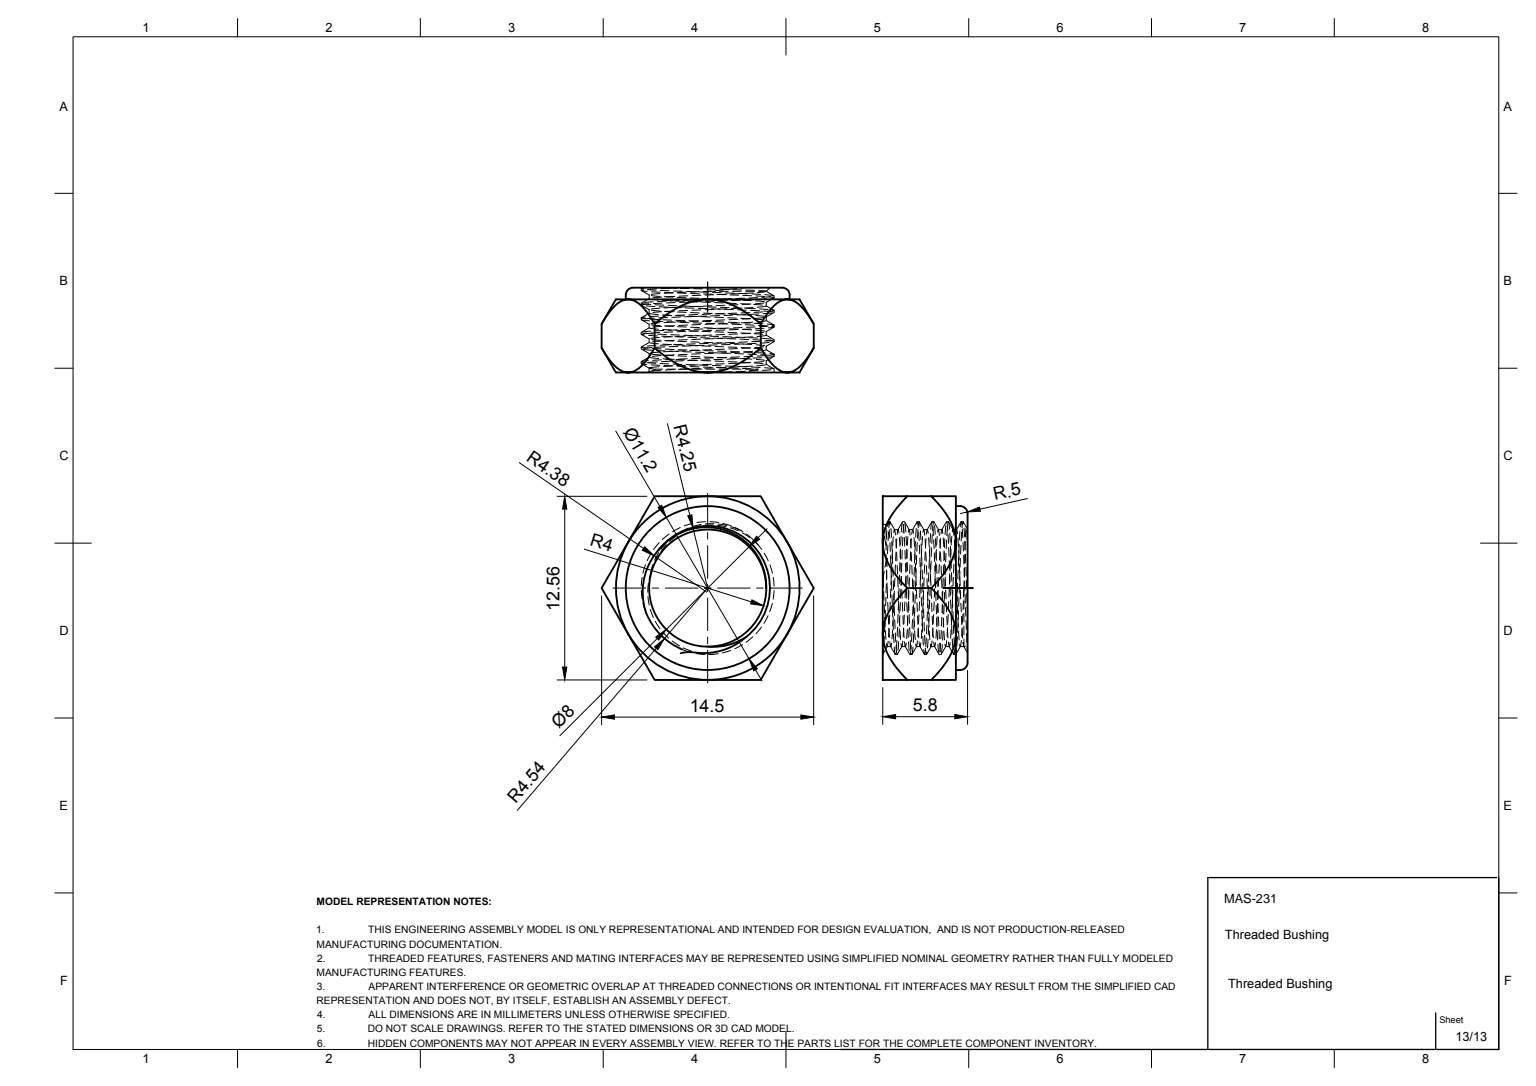
ISO-10303-21;
HEADER;
FILE_DESCRIPTION (('STEP AP214'),
    '1' );
FILE_NAME ( 'Threaded Bushing.step', '2026-10-04T02:08:54', ( '' ), ( '' ), 'STEP AP214', 'Unspecified', '' );
FILE_SCHEMA (( 'AUTOMOTIVE_DESIGN' ));
ENDSEC;
DATA;
#4=CARTESIAN_POINT ( 'NONE',  ( 0.07405724077823318263, -0.4114173227808823330, -0.1787899950787401604 ) ) ;
#5=CARTESIAN_POINT ( 'NONE',  ( -1.094772975963752103E-17, -0.9552165353793071745, -0.1787899950787401882 ) ) ;
#6=CONICAL_SURFACE ( 'NONE', #32970, 0.2471922904502826812, 0.5235987755982992597 ) ;
#7=CARTESIAN_POINT ( 'NONE',  ( -0.2471922332845153669, -0.07944658092495102131, -0.07441910580874835923 ) ) ;
#12=CARTESIAN_POINT ( 'NONE',  ( -0.07444174185955065859, -0.2446304237562738071, -0.1797182628040039087 ) ) ;
#13=CARTESIAN_POINT ( 'NONE',  ( -1.094772975963752103E-17, -0.1049468028749080684, -0.1787899950787401882 ) ) ;
#14=CARTESIAN_POINT ( 'NONE',  ( -1.094772975963752103E-17, -0.2465551180564728440, -0.1787899950787401882 ) ) ;
#15=CARTESIAN_POINT ( 'NONE',  ( 0.1787899950787401604, -0.1013779527021420185, -0.07405724077823318263 ) ) ;
#16=CARTESIAN_POINT ( 'NONE',  ( 0.2471913174570561644, -0.07307272215611475275, -0.08638584879597815958 ) ) ;
#20=DIRECTION ( 'NONE',  ( 0.000000000000000000, 0.000000000000000000, 1.000000000000000000 ) ) ;
#21=CARTESIAN_POINT ( 'NONE',  ( 0.1264236179284866091, -0.4581692912848189247, 0.1264236179284866091 ) ) ;
#25=CARTESIAN_POINT ( 'NONE',  ( -0.1632645169450111788, -0.09126532511120305502, 0.1911722030494052427 ) ) ;
#28=CARTESIAN_POINT ( 'NONE',  ( 0.000000000000000000, 0.09842519685039370636, 0.000000000000000000 ) ) ;
#30=CARTESIAN_POINT ( 'NONE',  ( -0.06523048226347956391, -0.9306102361129453548, -0.1574803149606300301 ) ) ;
#31=CARTESIAN_POINT ( 'NONE',  ( 0.1787899950787401604, -0.3425196849856064762, 0.07405724077823318263 ) ) ;
#34=CARTESIAN_POINT ( 'NONE',  ( -0.07405724077823318263, -1.016732283410803905, 0.1787899950787401604 ) ) ;
#43=CARTESIAN_POINT ( 'NONE',  ( 0.1574803149606299191, -1.139763779420031486, -1.928577636452523993E-17 ) ) ;
#55=CARTESIAN_POINT ( 'NONE',  ( 0.1787899950787401604, 0.01181102367581077228, 0.07405724077823318263 ) ) ;
#64=CARTESIAN_POINT ( 'NONE',  ( 0.1264236179284866091, -1.340183023347348623, 0.1264236179284866091 ) ) ;
#66=CARTESIAN_POINT ( 'NONE',  ( 0.1264236179284866091, -0.3006889763241893943, 0.1264236179284866091 ) ) ;
#74=CARTESIAN_POINT ( 'NONE',  ( -0.1264236179284866091, -1.693405511757259951, 0.1264236179284866091 ) ) ;
#77=CARTESIAN_POINT ( 'NONE',  ( -0.1540809957184832990, -0.09842519685039370636, 0.06850209239233011338 ) ) ;
#78=CARTESIAN_POINT ( 'NONE',  ( 0.1797182628040039087, -1.440496565488557978, 0.07444174185955046430 ) ) ;
#88=CARTESIAN_POINT ( 'NONE',  ( -0.1574803149606297803, -0.7632874014672766938, 0.06523048226347956391 ) ) ;
#89=CARTESIAN_POINT ( 'NONE',  ( 3.284318927891251994E-17, 0.1225393701325037388, 0.1787899950787401882 ) ) ;
#109=CARTESIAN_POINT ( 'NONE',  ( 0.1264236179284866091, -0.1038385826234017734, 0.1264236179284866091 ) ) ;
#117=CARTESIAN_POINT ( 'NONE',  ( 0.1113553986120547346, 0.1250000001075269596, -0.1113553986120547346 ) ) ;
#125=CARTESIAN_POINT ( 'NONE',  ( -0.1787899950787401604, -0.7668562516938051132, -0.07405724077823318263 ) ) ;
#133=ORIENTED_EDGE ( 'NONE', *, *, #14771, .F. ) ;
#135=CARTESIAN_POINT ( 'NONE',  ( 0.07405724077823318263, -0.4901574802611972093, -0.1787899950787401604 ) ) ;
#138=CARTESIAN_POINT ( 'NONE',  ( 3.301370929368692659E-17, -0.8573272741499744498, 0.1797182628040039365 ) ) ;
#149=CARTESIAN_POINT ( 'NONE',  ( 0.1113553986120547346, -0.6328740156405040507, 0.1113553986120547346 ) ) ;
#152=EDGE_CURVE ( 'NONE', #35410, #47206, #15470, .T. ) ;
#155=CARTESIAN_POINT ( 'NONE',  ( 0.1787899950787401882, -0.7288385826234015097, -2.189545951927503898E-17 ) ) ;
#164=CARTESIAN_POINT ( 'NONE',  ( 0.1113553986120547346, -1.617125984251968518, -0.1113553986120547346 ) ) ;
#171=CARTESIAN_POINT ( 'NONE',  ( 0.07405724077823318263, -1.435039370024976391, -0.1787899950787401604 ) ) ;
#177=CYLINDRICAL_SURFACE ( 'NONE', #43516, 0.1574803149606299191 ) ;
#178=CARTESIAN_POINT ( 'NONE',  ( -1.094772975963752103E-17, -0.3411672753158531690, -0.1787899950787401882 ) ) ;
#190=CARTESIAN_POINT ( 'NONE',  ( -0.1787899950787401604, -1.262795275536788386, 0.07405724077823318263 ) ) ;
#191=CARTESIAN_POINT ( 'NONE',  ( 0.1264236179284866091, -1.403051181048598384, 0.1264236179284866091 ) ) ;
#193=ADVANCED_FACE ( 'NONE', ( #1523 ), #30571, .F. ) ;
#200=CARTESIAN_POINT ( 'NONE',  ( 0.1113553986120547346, -0.3277559055118110520, 0.1113553986120547346 ) ) ;
#206=CARTESIAN_POINT ( 'NONE',  ( -0.1113553986120547346, -0.4950787400499527813, -0.1113553986120547346 ) ) ;
#211=CARTESIAN_POINT ( 'NONE',  ( -0.1574803149606297803, 0.1028543308161884995, 0.06523048226347956391 ) ) ;
#213=CARTESIAN_POINT ( 'NONE',  ( 0.07405724077823318263, -1.508858267662772867, -0.1787899950787401604 ) ) ;
#214=CARTESIAN_POINT ( 'NONE',  ( -0.1574803149606297803, -1.511318897530268712, 0.06523048226347956391 ) ) ;
#215=CARTESIAN_POINT ( 'NONE',  ( 0.1264236179284866091, -0.7780511810485984947, 0.1264236179284866091 ) ) ;
#216=CARTESIAN_POINT ( 'NONE',  ( -0.06523048226347956391, -1.097933070866141225, -0.1574803149606300301 ) ) ;
#226=CARTESIAN_POINT ( 'NONE',  ( 0.1574803149606300301, -1.339074803042078932, 0.06523048226347956391 ) ) ;
#253=CARTESIAN_POINT ( 'NONE',  ( -0.1787899950787401604, -0.4360236219934807145, 0.07405724077823318263 ) ) ;
#255=CARTESIAN_POINT ( 'NONE',  ( 0.1787899950787401604, -0.8494094487651332459, 0.07405724077823318263 ) ) ;
#258=CARTESIAN_POINT ( 'NONE',  ( -0.1797182628040039087, -0.2003390851735964984, -0.07444174185955065859 ) ) ;
#261=CARTESIAN_POINT ( 'NONE',  ( 0.1787899950787401604, -0.1172499524812071620, 0.07405724077823318263 ) ) ;
#262=CARTESIAN_POINT ( 'NONE',  ( -0.1264236179284866091, -0.1186023621509608300, 0.1264236179284866091 ) ) ;
#263=CARTESIAN_POINT ( 'NONE',  ( 0.2471920270787851259, -0.07566776403336712697, -0.08167830084036972749 ) ) ;
#268=CARTESIAN_POINT ( 'NONE',  ( -0.1787899950787401604, -0.4311023621509605386, 0.07405724077823318263 ) ) ;
#275=CARTESIAN_POINT ( 'NONE',  ( 0.1574803149606299191, -0.9429133857192442125, -1.928577636452523993E-17 ) ) ;
#276=CARTESIAN_POINT ( 'NONE',  ( 0.1264236179284866091, -0.2170275590013547307, -0.1264236179284866091 ) ) ;
#279=CARTESIAN_POINT ( 'NONE',  ( 0.1787899950787401604, -1.041338582623402287, -0.07405724077823318263 ) ) ;
#287=CARTESIAN_POINT ( 'NONE',  ( -0.06523048226347956391, -1.206200787294047228, -0.1574803149606300301 ) ) ;
#297=CARTESIAN_POINT ( 'NONE',  ( -0.1787899950787401604, 0.03149606304588949135, -0.07405724077823318263 ) ) ;
#306=CARTESIAN_POINT ( 'NONE',  ( 0.1787899950787401604, -1.258982235945774075, 0.07405724077823318263 ) ) ;
#309=CARTESIAN_POINT ( 'NONE',  ( -0.07405724077823318263, -0.2047244093950554844, -0.1787899950787401604 ) ) ;
#313=CARTESIAN_POINT ( 'NONE',  ( 0.000000000000000000, -0.09842519685039370636, 0.000000000000000000 ) ) ;
#317=CARTESIAN_POINT ( 'NONE',  ( -0.1787899950787401604, -1.656496062938362268, 0.07405724077823318263 ) ) ;
#318=CARTESIAN_POINT ( 'NONE',  ( 0.1787899950787401604, -1.715551181048599716, 0.07405724077823318263 ) ) ;
#320=APPLICATION_CONTEXT ( 'automotive_design' ) ;
#324=CARTESIAN_POINT ( 'NONE',  ( 3.301370929368692659E-17, -1.369138297772021673, 0.1797182628040039365 ) ) ;
#329=B_SPLINE_CURVE_WITH_KNOTS ( 'NONE', 3,
 ( #40653, #8085, #22708, #37314, #20055, #46161, #9758, #34449, #45674, #2308, #13357, #45919, #24148, #16938, #24370, #42328, #41837, #20757 ),
 .UNSPECIFIED., .F., .F.,
 ( 4, 2, 2, 2, 1, 1, 2, 2, 2, 4 ),
 ( 0.000000000000000000, 0.2499999999999993894, 0.3749999999999990008, 0.4374999999999987788, 0.4687499999999986122, 0.4843749999999986122, 0.4921874999999985567, 0.4999999999999985567, 0.7499999999999992228, 1.000000000000000000 ),
 .UNSPECIFIED. ) ;
#335=CARTESIAN_POINT ( 'NONE',  ( 0.1113553986120547346, -0.8198818896562519720, -0.1113553986120547346 ) ) ;
#349=CARTESIAN_POINT ( 'NONE',  ( -0.1270800023317771588, 0.1515309935665608287, -0.1270800023317771588 ) ) ;
#350=CARTESIAN_POINT ( 'NONE',  ( 0.1574803149606300301, -1.063484251860977059, 0.06523048226347956391 ) ) ;
#356=CARTESIAN_POINT ( 'NONE',  ( 0.07405724077823318263, -0.2244094487651340231, 0.1787899950787401604 ) ) ;
#360=CARTESIAN_POINT ( 'NONE',  ( -0.009745153983727199848, -0.04193537623276894638, 0.2798067035903421540 ) ) ;
#364=CARTESIAN_POINT ( 'NONE',  ( -9.642888182262618425E-18, 0.09055118120988918384, -0.1574803149606299191 ) ) ;
#368=VECTOR ( 'NONE', #12553, 39.37007874015748143 ) ;
#369=CARTESIAN_POINT ( 'NONE',  ( 0.1787899950787401882, -0.9021908973630964335, -2.189545951927503898E-17 ) ) ;
#372=AXIS2_PLACEMENT_3D ( 'NONE', #5692, #17413, #32052 ) ;
#373=ORIENTED_EDGE ( 'NONE', *, *, #26554, .F. ) ;
#379=CARTESIAN_POINT ( 'NONE',  ( -0.1787899950787401604, -0.4753937007336378473, 0.07405724077823318263 ) ) ;
#380=EDGE_CURVE ( 'NONE', #22666, #46167, #21394, .T. ) ;
#383=CARTESIAN_POINT ( 'NONE',  ( -0.1270800023317771588, -1.059098927693281622, 0.1270800023317771588 ) ) ;
#392=CARTESIAN_POINT ( 'NONE',  ( -0.1235961452251413406, -0.09842519685039370636, 0.2140748031496062798 ) ) ;
#396=CARTESIAN_POINT ( 'NONE',  ( -0.1787899950787401604, -0.8248031495525351975, 0.07405724077823318263 ) ) ;
#399=FACE_OUTER_BOUND ( 'NONE', #15103, .T. ) ;
#404=CARTESIAN_POINT ( 'NONE',  ( -0.06523048226347956391, -1.727854330708660902, -0.1574803149606300301 ) ) ;
#418=CARTESIAN_POINT ( 'NONE',  ( 0.07405724077823318263, -0.3436279052371127296, -0.1787899950787401604 ) ) ;
#419=CARTESIAN_POINT ( 'NONE',  ( 0.08603670706143877467, -0.09842519685039370636, 0.1221131442762555253 ) ) ;
#421=PLANE ( 'NONE',  #8031 ) ;
#430=CARTESIAN_POINT ( 'NONE',  ( 0.1787899950787401882, -1.284940944828125930, -2.189545951927503898E-17 ) ) ;
#431=CARTESIAN_POINT ( 'NONE',  ( 0.1264236179284866091, -1.481791338528913426, 0.1264236179284866091 ) ) ;
#438=CARTESIAN_POINT ( 'NONE',  ( -0.1113553986120547346, -0.2194881889763779514, 0.1113553986120547346 ) ) ;
#441=CARTESIAN_POINT ( 'NONE',  ( -0.1787899950787401604, -0.2047244093950554844, -0.07405724077823318263 ) ) ;
#453=CARTESIAN_POINT ( 'NONE',  ( -0.1264236179284866091, -1.531003936954110189, 0.1264236179284866091 ) ) ;
#454=CARTESIAN_POINT ( 'NONE',  ( 0.07405724077823318263, -0.8198818897100156322, 0.1787899950787401604 ) ) ;
#455=CARTESIAN_POINT ( 'NONE',  ( -0.06523048226347956391, -1.240649606299213614, 0.1574803149606297803 ) ) ;
#476=EDGE_CURVE ( 'NONE', #44070, #30751, #10635, .T. ) ;
#478=CARTESIAN_POINT ( 'NONE',  ( -0.2009290272083082973, -0.09842519685039370636, 0.1224581209280712624 ) ) ;
#484=CARTESIAN_POINT ( 'NONE',  ( 0.1787899950787401604, -0.8937007873478103326, 0.07405724077823318263 ) ) ;
#485=CARTESIAN_POINT ( 'NONE',  ( -0.1264236179284866091, -0.9010826771115905132, 0.1264236179284866091 ) ) ;
#488=CARTESIAN_POINT ( 'NONE',  ( 0.1797182628040039087, -0.2544729434413131597, -0.07444174185955065859 ) ) ;
#490=CARTESIAN_POINT ( 'NONE',  ( 0.07405724077823318263, -0.03248031490686641154, 0.1787899950787401604 ) ) ;
#501=CARTESIAN_POINT ( 'NONE',  ( -0.1787899950787401882, -0.3203740156942680994, 0.000000000000000000 ) ) ;
#503=CARTESIAN_POINT ( 'NONE',  ( 0.1787899950787401604, -1.164370078686393306, 0.07405724077823318263 ) ) ;
#524=CARTESIAN_POINT ( 'NONE',  ( -0.1264236179284866091, -0.08907480309584270284, -0.1264236179284866091 ) ) ;
#528=CARTESIAN_POINT ( 'NONE',  ( -0.1750152858685271595, -0.09851385417196180383, -0.1786646369836015769 ) ) ;
#532=CARTESIAN_POINT ( 'NONE',  ( 0.1787899950787401604, -1.455832629646562015, 0.07405724077823318263 ) ) ;
#534=CARTESIAN_POINT ( 'NONE',  ( 0.07405724077823318263, -0.4212598424659216856, 0.1787899950787401604 ) ) ;
#542=CARTESIAN_POINT ( 'NONE',  ( 0.07405724077823318263, -1.646653543253324026, 0.1787899950787401604 ) ) ;
#543=CARTESIAN_POINT ( 'NONE',  ( -0.1787899950787401604, -1.651574803095843258, 0.07405724077823318263 ) ) ;
#548=CARTESIAN_POINT ( 'NONE',  ( -1.100456976456230270E-17, -1.349453258401942746, -0.1797182628040039365 ) ) ;
#557=CARTESIAN_POINT ( 'NONE',  ( -1.094772975963752103E-17, 0.1422244095025824717, -0.1787899950787401882 ) ) ;
#570=CARTESIAN_POINT ( 'NONE',  ( 0.1797182628040039365, -0.06008317966178563369, -2.200913952912460540E-17 ) ) ;
#572=CARTESIAN_POINT ( 'NONE',  ( -0.1787899950787401604, -1.188976377898991688, -0.07405724077823318263 ) ) ;
#579=CARTESIAN_POINT ( 'NONE',  ( 3.284318927891251994E-17, -0.2268700786863941110, 0.1787899950787401882 ) ) ;
#582=EDGE_CURVE ( 'NONE', #35894, #1072, #33031, .T. ) ;
#583=CARTESIAN_POINT ( 'NONE',  ( -0.06523048226347935574, 0.09793307086614168322, 0.1574803149606300301 ) ) ;
#585=ORIENTED_EDGE ( 'NONE', *, *, #39318, .F. ) ;
#586=EDGE_CURVE ( 'NONE', #31109, #36213, #45187, .T. ) ;
#588=CARTESIAN_POINT ( 'NONE',  ( -0.1113553986120547346, 0.1348425197925665342, -0.1113553986120547346 ) ) ;
#594=CARTESIAN_POINT ( 'NONE',  ( 0.07405724077823318263, -0.9883129446071914348, 0.1787899950787401604 ) ) ;
#596=CARTESIAN_POINT ( 'NONE',  ( 0.1787899950787401604, 0.1348425197388028463, 0.07405724077823318263 ) ) ;
#605=CARTESIAN_POINT ( 'NONE',  ( -0.07444174185955065859, -1.071402077299582034, -0.1797182628040039087 ) ) ;
#612=CARTESIAN_POINT ( 'NONE',  ( 0.000000000000000000, -0.09842519685039370636, 0.000000000000000000 ) ) ;
#615=CARTESIAN_POINT ( 'NONE',  ( -0.07405724077823318263, -0.7411417322297018107, 0.1787899950787401604 ) ) ;
#620=LINE ( 'NONE', #7837, #8860 ) ;
#621=CARTESIAN_POINT ( 'NONE',  ( -0.1574803149606300301, -1.644192913385826404, -0.06523048226347956391 ) ) ;
#629=CARTESIAN_POINT ( 'NONE',  ( -0.06523048226347956391, 0.05364173239099160467, -0.1574803149606300301 ) ) ;
#642=CARTESIAN_POINT ( 'NONE',  ( -0.07405724077823318263, -0.5995334170481365632, 0.1787899950787401604 ) ) ;
#645=DIRECTION ( 'NONE',  ( 0.000000000000000000, 1.000000000000000000, 0.000000000000000000 ) ) ;
#647=CARTESIAN_POINT ( 'NONE',  ( -0.1264236179284866091, -1.743726330433962524, 0.1264236179284866091 ) ) ;
#652=CARTESIAN_POINT ( 'NONE',  ( 0.1264236179284866091, -1.289862204670645607, 0.1264236179284866091 ) ) ;
#654=CARTESIAN_POINT ( 'NONE',  ( 0.07405724077823318263, -1.587598425143086800, -0.1787899950787401604 ) ) ;
#663=CARTESIAN_POINT ( 'NONE',  ( -0.1113553986120547346, -0.2293307086614173318, -0.1113553986120547346 ) ) ;
#666=CARTESIAN_POINT ( 'NONE',  ( -0.1427036564498907201, -0.09517011092317628762, -0.1080556551396093801 ) ) ;
#672=CARTESIAN_POINT ( 'NONE',  ( -0.1690815567638284667, -0.08955967048287666321, -0.02567216645670302583 ) ) ;
#681=CARTESIAN_POINT ( 'NONE',  ( -0.07405724077823318263, -1.607283464513165949, 0.1787899950787401604 ) ) ;
#682=CARTESIAN_POINT ( 'NONE',  ( -0.1787899950787401604, -0.7952755904974174728, -0.07405724077823318263 ) ) ;
#683=CARTESIAN_POINT ( 'NONE',  ( -0.1113553986120547346, -1.252952755905511806, -0.1113553986120547346 ) ) ;
#704=CARTESIAN_POINT ( 'NONE',  ( -0.1919739359782932919, -0.09842519685039370636, 0.1351110688617698785 ) ) ;
#713=B_SPLINE_CURVE_WITH_KNOTS ( 'NONE', 3,
 ( #38757, #41598, #38277, #27534 ),
 .UNSPECIFIED., .F., .F.,
 ( 4, 4 ),
 ( 0.000000000000000000, 1.000000000000000000 ),
 .UNSPECIFIED. ) ;
#714=CARTESIAN_POINT ( 'NONE',  ( 0.1264236179284866091, -0.9256889763241890057, -0.1264236179284866091 ) ) ;
#715=CARTESIAN_POINT ( 'NONE',  ( -0.07405724077823318263, -0.9921259841982054128, -0.1787899950787401604 ) ) ;
#718=CARTESIAN_POINT ( 'NONE',  ( 0.07444174185955065859, -0.3824256993468252430, 0.1797182628040039087 ) ) ;
#719=CARTESIAN_POINT ( 'NONE',  ( -0.1574803149606297803, 0.09301181102362203468, 0.06523048226347956391 ) ) ;
#720=CARTESIAN_POINT ( 'NONE',  ( 0.1787899950787401604, -0.02755905506434671789, 0.07405724077823318263 ) ) ;
#733=CARTESIAN_POINT ( 'NONE',  ( -0.07405724077823318263, -0.2342519684501733479, 0.1787899950787401604 ) ) ;
#735=CARTESIAN_POINT ( 'NONE',  ( -1.094772975963752103E-17, -1.270177165300566902, -0.1787899950787401882 ) ) ;
#744=CARTESIAN_POINT ( 'NONE',  ( 0.1574803149606299191, -1.218503936900346529, -1.928577636452523993E-17 ) ) ;
#746=CARTESIAN_POINT ( 'NONE',  ( 0.01529509707327361516, -0.09839281432029055308, -0.1781982434423184380 ) ) ;
#757=FACE_OUTER_BOUND ( 'NONE', #34050, .T. ) ;
#762=CARTESIAN_POINT ( 'NONE',  ( 0.1264236179284866091, -1.379553102087506256, 0.1264236179284866091 ) ) ;
#763=VERTEX_POINT ( 'NONE', #18849 ) ;
#765=CARTESIAN_POINT ( 'NONE',  ( -0.07405724077823318263, -0.4655511810485986057, 0.1787899950787401604 ) ) ;
#774=CARTESIAN_POINT ( 'NONE',  ( -0.1787899950787401604, -1.740157480261197875, -0.07405724077823318263 ) ) ;
#775=CARTESIAN_POINT ( 'NONE',  ( 0.1787899950787401604, -1.710629921206078041, -0.07405724077823318263 ) ) ;
#781=CARTESIAN_POINT ( 'NONE',  ( 3.301370929368692659E-17, -1.447878455252336716, 0.1797182628040039365 ) ) ;
#790=CARTESIAN_POINT ( 'NONE',  ( -0.1574803149606297803, -0.8026574802074324388, 0.06523048226347956391 ) ) ;
#791=CARTESIAN_POINT ( 'NONE',  ( 0.1264236179284866091, 0.1274606299750234428, 0.1264236179284866091 ) ) ;
#799=VERTEX_POINT ( 'NONE', #25603 ) ;
#802=VERTEX_POINT ( 'NONE', #40870 ) ;
#803=CARTESIAN_POINT ( 'NONE',  ( 0.1797182628040039365, -0.02071310092162823024, -2.200913952912460540E-17 ) ) ;
#804=CARTESIAN_POINT ( 'NONE',  ( 0.1264236179284866091, -1.289862204670645607, 0.1264236179284866091 ) ) ;
#812=CARTESIAN_POINT ( 'NONE',  ( -1.094772975963752103E-17, -0.1678149605761578844, -0.1787899950787401882 ) ) ;
#820=CARTESIAN_POINT ( 'NONE',  ( -0.06523048226347956391, -0.08907480304207930633, 0.1574803149606297803 ) ) ;
#826=CARTESIAN_POINT ( 'NONE',  ( -0.1264236179284866091, -0.9267971965756948149, -0.1264236179284866091 ) ) ;
#828=CARTESIAN_POINT ( 'NONE',  ( -0.07405724077823318263, 0.08562992131360593062, 0.1787899950787401604 ) ) ;
#835=AXIS2_PLACEMENT_3D ( 'NONE', #29189, #20976, #40131 ) ;
#836=CARTESIAN_POINT ( 'NONE',  ( 0.07405724077823318263, -0.5442913385289138706, 0.1787899950787401604 ) ) ;
#843=CARTESIAN_POINT ( 'NONE',  ( 0.1270800023317771588, -1.039413888323202695, -0.1270800023317771588 ) ) ;
#844=CARTESIAN_POINT ( 'NONE',  ( 0.1731942250296887864, 0.1299212598425197318, 0.03910837931845940335 ) ) ;
#854=CARTESIAN_POINT ( 'NONE',  ( 0.1113553986120547346, -0.7017716534357795188, -0.1113553986120547346 ) ) ;
#858=CARTESIAN_POINT ( 'NONE',  ( -0.1787899950787401882, -0.7091535432533228045, 0.000000000000000000 ) ) ;
#866=CARTESIAN_POINT ( 'NONE',  ( -0.06523048226347956391, -1.634350393700787496, 0.1574803149606297803 ) ) ;
#874=CARTESIAN_POINT ( 'NONE',  ( -1.094772975963752103E-17, -1.471948818843874074, -0.1787899950787401882 ) ) ;
#883=CARTESIAN_POINT ( 'NONE',  ( 0.07405724077823318263, -0.5798483776780570809, -0.1787899950787401604 ) ) ;
#884=CARTESIAN_POINT ( 'NONE',  ( 0.02785187604205846545, -0.08955996554169548540, 0.2176922158899677329 ) ) ;
#891=CARTESIAN_POINT ( 'NONE',  ( 0.2471922904502826812, -0.03219022224904106305, 0.1427165354330708902 ) ) ;
#896=CARTESIAN_POINT ( 'NONE',  ( 0.1264236179284866091, -1.358759842465921297, -0.1264236179284866091 ) ) ;
#897=CARTESIAN_POINT ( 'NONE',  ( 0.07405724077823318263, -1.523622047190330564, 0.1787899950787401604 ) ) ;
#906=CARTESIAN_POINT ( 'NONE',  ( 0.1574803149606300301, -0.2416338582677168279, -0.06523048226347956391 ) ) ;
#917=CARTESIAN_POINT ( 'NONE',  ( 0.1113553986120547346, -0.5442913384751496553, -0.1113553986120547346 ) ) ;
#919=CARTESIAN_POINT ( 'NONE',  ( -0.1547363509471673670, -0.08956143428533665241, 0.05872201630027999719 ) ) ;
#925=CARTESIAN_POINT ( 'NONE',  ( 2.892866454678787531E-17, -0.01771653543307086590, 0.1574803149606299191 ) ) ;
#926=CARTESIAN_POINT ( 'NONE',  ( 0.1787899950787401604, -1.558070866087969630, 0.07405724077823318263 ) ) ;
#927=CARTESIAN_POINT ( 'NONE',  ( -0.07405724077823318263, -0.9576771653005667906, -0.1787899950787401604 ) ) ;
#928=CARTESIAN_POINT ( 'NONE',  ( 0.06523048226347956391, -1.142224409448818534, -0.1574803149606300301 ) ) ;
#949=CARTESIAN_POINT ( 'NONE',  ( -0.1522652282534474322, -0.09842519685039370636, -0.2000201865208625918 ) ) ;
#958=CARTESIAN_POINT ( 'NONE',  ( 0.1264236179284866091, -0.8174212597887557941, 0.1264236179284866091 ) ) ;
#959=CARTESIAN_POINT ( 'NONE',  ( -0.1787899950787401882, -1.063484251914740275, 0.000000000000000000 ) ) ;
#963=CARTESIAN_POINT ( 'NONE',  ( -0.1797182628040039087, -0.3922682190318645401, 0.07444174185955065859 ) ) ;
#965=CARTESIAN_POINT ( 'NONE',  ( 0.1264236179284866091, -0.1382874015210397711, -0.1264236179284866091 ) ) ;
#977=CARTESIAN_POINT ( 'NONE',  ( 0.1787899950787401604, -0.4557086613635593086, -0.07405724077823318263 ) ) ;
#979=CARTESIAN_POINT ( 'NONE',  ( -0.1787899950787401882, -1.299704724355684959, 0.000000000000000000 ) ) ;
#987=CARTESIAN_POINT ( 'NONE',  ( -0.06523048226347956391, -1.166830708553891371, -0.1574803149606300301 ) ) ;
#992=CARTESIAN_POINT ( 'NONE',  ( -0.05462378473120000494, -0.09842519705081047288, -0.1712222294880737516 ) ) ;
#1009=CARTESIAN_POINT ( 'NONE',  ( -0.1787899950787401882, -1.473057039095379883, 0.000000000000000000 ) ) ;
#1011=CARTESIAN_POINT ( 'NONE',  ( 0.1264236179284866091, -0.3695866141194649179, -0.1264236179284866091 ) ) ;
#1021=CARTESIAN_POINT ( 'NONE',  ( 0.1264236179284866091, -1.722933070812378009, 0.1264236179284866091 ) ) ;
#1022=CARTESIAN_POINT ( 'NONE',  ( -0.1787899950787401882, -1.772145669237574994, 0.000000000000000000 ) ) ;
#1024=ORIENTED_EDGE ( 'NONE', *, *, #5865, .T. ) ;
#1028=CARTESIAN_POINT ( 'NONE',  ( -0.1113553986120547346, -0.7312992125984252301, 0.1113553986120547346 ) ) ;
#1030=CARTESIAN_POINT ( 'NONE',  ( -0.1797182628040039087, -1.342071368638164675, -0.07444174185955065859 ) ) ;
#1039=CARTESIAN_POINT ( 'NONE',  ( -0.07405724077823318263, 0.1200787402112438867, 0.1787899950787401604 ) ) ;
#1051=CARTESIAN_POINT ( 'NONE',  ( 0.1797182628040039365, -0.09945325840194331468, -2.200913952912460540E-17 ) ) ;
#1052=CARTESIAN_POINT ( 'NONE',  ( -0.1787899950787401604, -1.267716535379307619, -0.07405724077823318263 ) ) ;
#1061=CARTESIAN_POINT ( 'NONE',  ( -0.06648378651140092466, -0.08350519546677943883, -0.2470477387548498660 ) ) ;
#1062=CIRCLE ( 'NONE', #4901, 0.2471922904502826812 ) ;
#1065=CARTESIAN_POINT ( 'NONE',  ( -0.06523048226347956391, 0.01427165365083412490, -0.1574803149606300301 ) ) ;
#1071=CARTESIAN_POINT ( 'NONE',  ( -1.094772975963752103E-17, -0.9317184564182144912, -0.1787899950787401882 ) ) ;
#1072=VERTEX_POINT ( 'NONE', #4941 ) ;
#1073=CARTESIAN_POINT ( 'NONE',  ( -0.07405724077823318263, 0.006889763833291078637, 0.1787899950787401604 ) ) ;
#1081=CARTESIAN_POINT ( 'NONE',  ( 3.284318927891251994E-17, -0.5467519684501732646, 0.1787899950787401882 ) ) ;
#1086=CARTESIAN_POINT ( 'NONE',  ( 3.301370929368692659E-17, -0.9360674316302894926, 0.1797182628040039365 ) ) ;
#1097=CARTESIAN_POINT ( 'NONE',  ( -0.1787899950787401604, 0.08070866147108628208, 0.07405724077823318263 ) ) ;
#1102=CARTESIAN_POINT ( 'NONE',  ( 3.284318927891251994E-17, -0.7780511810485984947, 0.1787899950787401882 ) ) ;
#1106=CARTESIAN_POINT ( 'NONE',  ( -0.1113553986120547346, -1.715551180994834723, -0.1113553986120547346 ) ) ;
#1109=CARTESIAN_POINT ( 'NONE',  ( 0.06523048226347956391, -1.654035433070866423, -0.1574803149606300301 ) ) ;
#1115=CARTESIAN_POINT ( 'NONE',  ( 0.1787899950787401604, 0.09547244099864542199, -0.07405724077823318263 ) ) ;
#1116=CARTESIAN_POINT ( 'NONE',  ( -1.094772975963752103E-17, -1.511318897584031484, -0.1787899950787401882 ) ) ;
#1128=CARTESIAN_POINT ( 'NONE',  ( -0.07405724077823318263, -0.5601633383079792639, 0.1787899950787401604 ) ) ;
#1129=CARTESIAN_POINT ( 'NONE',  ( -0.2359654055811763462, -0.08955966323838543408, 0.02109953285558708452 ) ) ;
#1133=CARTESIAN_POINT ( 'NONE',  ( 0.000000000000000000, 0.09842519685039370636, 0.000000000000000000 ) ) ;
#1135=CARTESIAN_POINT ( 'NONE',  ( 3.284318927891251994E-17, -1.778175149331602256, 0.1787899950787401882 ) ) ;
#1138=CARTESIAN_POINT ( 'NONE',  ( -0.1787899950787401604, -1.341535433017102541, 0.07405724077823318263 ) ) ;
#1139=CARTESIAN_POINT ( 'NONE',  ( 3.284318927891251994E-17, -1.486712598371433103, 0.1787899950787401882 ) ) ;
#1146=CARTESIAN_POINT ( 'NONE',  ( -0.06523048226347956391, -0.2317913385826771144, -0.1574803149606300301 ) ) ;
#1152=CARTESIAN_POINT ( 'NONE',  ( -0.1545411696117860445, -0.09842519685039370636, -0.08990488994085453489 ) ) ;
#1156=CARTESIAN_POINT ( 'NONE',  ( -0.06523048226347956391, -0.5369094487113711400, -0.1574803149606300301 ) ) ;
#1157=CARTESIAN_POINT ( 'NONE',  ( -0.1807077244524717130, -0.08350519546717886932, 0.1811005174367878168 ) ) ;
#1159=CARTESIAN_POINT ( 'NONE',  ( -0.1009669065382620273, -0.08956173115452045752, 0.1239132365318445506 ) ) ;
#1165=CARTESIAN_POINT ( 'NONE',  ( 0.07405724077823318263, -1.681102362150960650, 0.1787899950787401604 ) ) ;
#1166=CARTESIAN_POINT ( 'NONE',  ( 0.1264236179284866091, -0.9256889763241890057, -0.1264236179284866091 ) ) ;
#1167=CARTESIAN_POINT ( 'NONE',  ( 0.06523048226347956391, -1.220964566929134687, -0.1574803149606300301 ) ) ;
#1175=CARTESIAN_POINT ( 'NONE',  ( 0.1113553986120547346, -1.371062992018456717, -0.1113553986120547346 ) ) ;
#1185=CARTESIAN_POINT ( 'NONE',  ( 0.05837987205262076124, 0.07899857248962811884, 0.2517274360213053175 ) ) ;
#1191=CARTESIAN_POINT ( 'NONE',  ( 0.01579849016993808974, -0.09851382911741830839, 0.1545074369619750254 ) ) ;
#1201=CARTESIAN_POINT ( 'NONE',  ( 0.1787899950787401604, -0.8887795275052913224, -0.07405724077823318263 ) ) ;
#1202=CARTESIAN_POINT ( 'NONE',  ( -0.1787899950787401604, -1.100393700733639069, 0.07405724077823318263 ) ) ;
#1205=CARTESIAN_POINT ( 'NONE',  ( 0.07444174185955046430, -0.4070319985594234580, -0.1797182628040039087 ) ) ;
#1206=CARTESIAN_POINT ( 'NONE',  ( -0.1574803149606300301, -1.791830708553890261, -0.06523048226347956391 ) ) ;
#1207=CARTESIAN_POINT ( 'NONE',  ( -0.1113553986120547346, 0.1643700787401574936, -0.1113553986120547346 ) ) ;
#1217=CARTESIAN_POINT ( 'NONE',  ( 3.284318927891251994E-17, -0.3892716534895436786, 0.1787899950787401882 ) ) ;
#1219=CARTESIAN_POINT ( 'NONE',  ( -0.07405724077823318263, -1.292322834591905778, 0.1787899950787401604 ) ) ;
#1230=CARTESIAN_POINT ( 'NONE',  ( 0.04979026054520423183, -0.09842589400172224723, -0.1717333828277539942 ) ) ;
#1235=ADVANCED_FACE ( 'NONE', ( #12987 ), #46257, .F. ) ;
#1240=CARTESIAN_POINT ( 'NONE',  ( -0.1947286603072740374, -0.09851385302161634605, -0.1548760358685606353 ) ) ;
#1247=CARTESIAN_POINT ( 'NONE',  ( -0.1264236179284866091, -1.399238141457584739, -0.1264236179284866091 ) ) ;
#1250=CARTESIAN_POINT ( 'NONE',  ( 0.1264236179284866091, -0.4581692912848189247, 0.1264236179284866091 ) ) ;
#1254=CARTESIAN_POINT ( 'NONE',  ( -0.2471922904502826812, -0.09842519685039370636, 5.914624404477007554E-17 ) ) ;
#1257=CARTESIAN_POINT ( 'NONE',  ( -0.07405724077823318263, -1.730314960576156968, 0.1787899950787401604 ) ) ;
#1258=CARTESIAN_POINT ( 'NONE',  ( -0.07405724077823318263, -1.804133858213953889, 0.1787899950787401604 ) ) ;
#1264=CARTESIAN_POINT ( 'NONE',  ( 0.1113553986120547346, -0.7608267716535432879, 0.1113553986120547346 ) ) ;
#1266=CARTESIAN_POINT ( 'NONE',  ( -0.1797182628040039087, -1.573370581236589683, 0.07444174185955065859 ) ) ;
#1275=CARTESIAN_POINT ( 'NONE',  ( -0.1787899950787401604, -0.007874015694267972806, -0.07405724077823318263 ) ) ;
#1288=CARTESIAN_POINT ( 'NONE',  ( -0.07444174185955065859, -0.08715010879564398516, -0.1797182628040039087 ) ) ;
#1289=CARTESIAN_POINT ( 'NONE',  ( 0.1787899950787401604, -1.366141732229700478, 0.07405724077823318263 ) ) ;
#1297=EDGE_CURVE ( 'NONE', #10382, #802, #31438, .T. ) ;
#1299=EDGE_LOOP ( 'NONE', ( #44521, #27760, #38088 ) ) ;
#1306=CARTESIAN_POINT ( 'NONE',  ( -9.642888182262618425E-18, 0.01181102372957427288, -0.1574803149606299191 ) ) ;
#1311=CARTESIAN_POINT ( 'NONE',  ( 0.1787899950787401604, -1.017840503662311047, -0.07405724077823318263 ) ) ;
#1313=CARTESIAN_POINT ( 'NONE',  ( 0.07405724077823318263, 0.09055118115612580121, 0.1787899950787401604 ) ) ;
#1318=CARTESIAN_POINT ( 'NONE',  ( 0.07405724077823318263, -0.7017716534895438452, 0.1787899950787401604 ) ) ;
#1323=CARTESIAN_POINT ( 'NONE',  ( 0.1797182628040039087, -1.041874518244462422, -0.07444174185955065859 ) ) ;
#1331=CARTESIAN_POINT ( 'NONE',  ( 0.06523048226347956391, -0.6993110235145204578, -0.1574803149606300301 ) ) ;
#1337=CARTESIAN_POINT ( 'NONE',  ( -0.07405724077823318263, -0.8592519684501739308, 0.1787899950787401604 ) ) ;
#1343=CARTESIAN_POINT ( 'NONE',  ( -0.1574803149606297803, -1.668799212490898576, 0.06523048226347956391 ) ) ;
#1347=CARTESIAN_POINT ( 'NONE',  ( 2.892866454678787531E-17, -1.789370078740157410, 0.1574803149606299191 ) ) ;
#1352=CARTESIAN_POINT ( 'NONE',  ( -0.06523048226347956391, -0.3400590550105831444, -0.1574803149606300301 ) ) ;
#1353=CARTESIAN_POINT ( 'NONE',  ( 0.1787899950787401882, -1.599901574749385880, -2.189545951927503898E-17 ) ) ;
#1364=CARTESIAN_POINT ( 'NONE',  ( -0.07405724077823318263, -0.4961869603552226948, -0.1787899950787401604 ) ) ;
#1365=CARTESIAN_POINT ( 'NONE',  ( 0.1120789836339634027, -0.08956013912318722126, 0.1830409950616023740 ) ) ;
#1371=CARTESIAN_POINT ( 'NONE',  ( 0.1787899950787401604, -1.558070866087969630, -0.07405724077823318263 ) ) ;
#1372=CARTESIAN_POINT ( 'NONE',  ( 0.1264236179284866091, -1.590059055064346305, -0.1264236179284866091 ) ) ;
#1378=CARTESIAN_POINT ( 'NONE',  ( -0.1113553986120547346, -0.4261811023622047445, -0.1113553986120547346 ) ) ;
#1389=CARTESIAN_POINT ( 'NONE',  ( -0.1154458135679224812, -0.08956175409534371246, 0.1128118131157532372 ) ) ;
#1390=CARTESIAN_POINT ( 'NONE',  ( 0.1787899950787401604, -0.4901574802611972093, -0.07405724077823318263 ) ) ;
#1396=CARTESIAN_POINT ( 'NONE',  ( -0.06523048226347956391, -0.03494094488188976416, -0.1574803149606300301 ) ) ;
#1397=CARTESIAN_POINT ( 'NONE',  ( 0.1787899950787401882, -1.713090551127338657, -2.189545951927503898E-17 ) ) ;
#1398=CARTESIAN_POINT ( 'NONE',  ( 0.07405724077823318263, -0.9379921259304876413, 0.1787899950787401604 ) ) ;
#1399=CARTESIAN_POINT ( 'NONE',  ( -0.1113553986120547346, -1.282480314960629864, 0.1113553986120547346 ) ) ;
#1408=CARTESIAN_POINT ( 'NONE',  ( 0.1574803149606300301, -0.0004921258767249256719, 0.06523048226347956391 ) ) ;
#1422=CARTESIAN_POINT ( 'NONE',  ( -0.2092218244630917323, -0.09842519685039370636, 0.1092665889510173183 ) ) ;
#1424=CIRCLE ( 'NONE', #38924, 0.2471922904502826812 ) ;
#1427=CARTESIAN_POINT ( 'NONE',  ( -0.1264236179284866091, -0.9158464566391496531, -0.1264236179284866091 ) ) ;
#1429=CARTESIAN_POINT ( 'NONE',  ( -0.07405724077823318263, -1.110236220418677533, -0.1787899950787401604 ) ) ;
#1433=CARTESIAN_POINT ( 'NONE',  ( -1.100456976456230270E-17, -0.2864611324176913332, -0.1797182628040039365 ) ) ;
#1434=CARTESIAN_POINT ( 'NONE',  ( -0.06523048226347956391, -1.821358267609009651, 0.1574803149606297803 ) ) ;
#1437=CARTESIAN_POINT ( 'NONE',  ( 0.1264236179284866091, -0.1481299212060789294, 0.1264236179284866091 ) ) ;
#1447=CARTESIAN_POINT ( 'NONE',  ( -0.06523048226347956391, -0.9945866140657014798, 0.1574803149606297803 ) ) ;
#1448=CARTESIAN_POINT ( 'NONE',  ( 0.1264236179284866091, -0.3843503936470239468, 0.1264236179284866091 ) ) ;
#1450=CARTESIAN_POINT ( 'NONE',  ( 0.1787899950787401604, -1.203740157426551383, 0.07405724077823318263 ) ) ;
#1456=CARTESIAN_POINT ( 'NONE',  ( -0.1113553986120547346, -1.233267716427905336, 0.1113553986120547346 ) ) ;
#1460=CARTESIAN_POINT ( 'NONE',  ( -0.1209429854940891474, -0.09842561477428417305, -0.1316810161538188584 ) ) ;
#1465=CARTESIAN_POINT ( 'NONE',  ( -0.1158283541424031532, -0.08956345598586890056, -0.1361971163587911426 ) ) ;
#1477=CARTESIAN_POINT ( 'NONE',  ( 0.1787899950787401882, -1.571482235945773853, -2.189545951927503898E-17 ) ) ;
#1480=CARTESIAN_POINT ( 'NONE',  ( 3.284318927891251994E-17, -0.4630905511273386010, 0.1787899950787401882 ) ) ;
#1487=CARTESIAN_POINT ( 'NONE',  ( -1.094772975963752103E-17, -0.2121062991588350544, -0.1787899950787401882 ) ) ;
#1490=CARTESIAN_POINT ( 'NONE',  ( 0.1787899950787401604, -1.715551181048599716, -0.07405724077823318263 ) ) ;
#1496=CARTESIAN_POINT ( 'NONE',  ( 0.06523048226347956391, -0.8026574803149603143, 0.1574803149606297803 ) ) ;
#1498=CARTESIAN_POINT ( 'NONE',  ( 3.301370929368692659E-17, -1.644728848953123990, 0.1797182628040039365 ) ) ;
#1505=CARTESIAN_POINT ( 'NONE',  ( 0.000000000000000000, 0.09842519685039370636, 0.000000000000000000 ) ) ;
#1509=CARTESIAN_POINT ( 'NONE',  ( 0.1264236179284866091, 0.01919291343959031448, -0.1264236179284866091 ) ) ;
#1517=ORIENTED_EDGE ( 'NONE', *, *, #16320, .F. ) ;
#1521=CARTESIAN_POINT ( 'NONE',  ( -0.1787899950787401604, -1.341535433017102541, 0.07405724077823318263 ) ) ;
#1523=FACE_OUTER_BOUND ( 'NONE', #20708, .T. ) ;
#1537=CARTESIAN_POINT ( 'NONE',  ( -0.06523048226347956391, -0.02509842508932335833, -0.1574803149606300301 ) ) ;
#1539=ORIENTED_EDGE ( 'NONE', *, *, #45161, .T. ) ;
#1545=CARTESIAN_POINT ( 'NONE',  ( -0.1787899950787401882, -1.039986172953647481, 0.000000000000000000 ) ) ;
#1548=CARTESIAN_POINT ( 'NONE',  ( -0.07405724077823318263, 0.04625984257344856188, 0.1787899950787401604 ) ) ;
#1549=EDGE_LOOP ( 'NONE', ( #2403, #29375, #9278, #18291, #6691, #19468 ) ) ;
#1553=CARTESIAN_POINT ( 'NONE',  ( 0.1787899950787401882, -0.5762795275052914334, -2.189545951927503898E-17 ) ) ;
#1558=CARTESIAN_POINT ( 'NONE',  ( 0.1797182628040039087, -1.159984754464934653, -0.07444174185955065859 ) ) ;
#1559=CARTESIAN_POINT ( 'NONE',  ( 0.1540151740152538029, 0.1299212598425197041, -0.07158477921181821690 ) ) ;
#1570=CARTESIAN_POINT ( 'NONE',  ( -0.1787899950787401604, 0.07578740162856664742, -0.07405724077823318263 ) ) ;
#1578=CARTESIAN_POINT ( 'NONE',  ( 0.06523048226347956391, -1.658956692805858557, 0.1574803149606297803 ) ) ;
#1582=CARTESIAN_POINT ( 'NONE',  ( 0.05769093565149619601, -0.07859528327913710422, 0.2521251929553415816 ) ) ;
#1583=CARTESIAN_POINT ( 'NONE',  ( -0.1574803149606297803, -1.796751968503936814, 0.06523048226347956391 ) ) ;
#1586=CARTESIAN_POINT ( 'NONE',  ( 0.000000000000000000, -0.09842519685039370636, 0.000000000000000000 ) ) ;
#1589=CARTESIAN_POINT ( 'NONE',  ( -0.1574803149606297803, -0.3695866140657014243, 0.06523048226347956391 ) ) ;
#1590=CARTESIAN_POINT ( 'NONE',  ( 0.1787899950787401604, -1.518700787347811554, -0.07405724077823318263 ) ) ;
#1594=ORIENTED_EDGE ( 'NONE', *, *, #10024, .F. ) ;
#1597=CARTESIAN_POINT ( 'NONE',  ( -0.07405724077823318263, -0.5749271178355379597, -0.1787899950787401604 ) ) ;
#1598=CARTESIAN_POINT ( 'NONE',  ( 0.2035752408203165831, -0.08956008440634705137, -0.0002272480696794984621 ) ) ;
#1605=CARTESIAN_POINT ( 'NONE',  ( 0.07405724077823318263, -1.815084598150499273, 0.1787899950787401604 ) ) ;
#1609=ADVANCED_FACE ( 'NONE', ( #15284, #29934 ), #13123, .F. ) ;
#1612=CARTESIAN_POINT ( 'NONE',  ( 3.284318927891251994E-17, -1.491633858213953001, 0.1787899950787401882 ) ) ;
#1617=CARTESIAN_POINT ( 'NONE',  ( -0.1270800023317771588, -0.6653981402917066301, 0.1270800023317771588 ) ) ;
#1622=CARTESIAN_POINT ( 'NONE',  ( -0.1574803149606299191, -0.3818897637795276023, 0.000000000000000000 ) ) ;
#1637=CARTESIAN_POINT ( 'NONE',  ( 0.1787899950787401604, -0.6131889763241887836, 0.07405724077823318263 ) ) ;
#1641=CARTESIAN_POINT ( 'NONE',  ( -0.07117121207836790697, -0.08956324299011318713, 0.1404802767937309016 ) ) ;
#1645=CARTESIAN_POINT ( 'NONE',  ( -0.1264236179284866091, -1.777066929080094670, -0.1264236179284866091 ) ) ;
#1646=CARTESIAN_POINT ( 'NONE',  ( -0.1787899950787401604, -0.8346456692375755493, -0.07405724077823318263 ) ) ;
#1648=CARTESIAN_POINT ( 'NONE',  ( 0.1113553986120547346, -1.380905511811023834, -0.1113553986120547346 ) ) ;
#1665=CARTESIAN_POINT ( 'NONE',  ( -0.1572451146043662151, 0.09317026862874178139, 0.1946475616205573522 ) ) ;
#1668=CARTESIAN_POINT ( 'NONE',  ( 0.2033597642235094594, -0.09842519685039370636, -0.03144620579497787310 ) ) ;
#1675=ORIENTED_EDGE ( 'NONE', *, *, #35776, .T. ) ;
#1678=CARTESIAN_POINT ( 'NONE',  ( 0.07405724077823318263, -0.9773622046706458288, 0.1787899950787401604 ) ) ;
#1679=CARTESIAN_POINT ( 'NONE',  ( -0.07405724077823318263, -1.228346456639149542, -0.1787899950787401604 ) ) ;
#1682=CARTESIAN_POINT ( 'NONE',  ( -0.1797182628040039087, -0.3528981402917069077, 0.07444174185955065859 ) ) ;
#1683=CARTESIAN_POINT ( 'NONE',  ( -0.06523048226347956391, -1.781988188868851575, 0.1574803149606297803 ) ) ;
#1685=CARTESIAN_POINT ( 'NONE',  ( 0.1113553986120547346, 0.07578740157480315376, -0.1113553986120547346 ) ) ;
#1692=CARTESIAN_POINT ( 'NONE',  ( 0.07405724077823318263, -0.4114173227808823330, -0.1787899950787401604 ) ) ;
#1694=CARTESIAN_POINT ( 'NONE',  ( 0.1787899950787401604, -1.439960629867495401, 0.07405724077823318263 ) ) ;
#1716=CARTESIAN_POINT ( 'NONE',  ( -0.03350987669894700538, -0.09851384946037776424, 0.2233477092115621898 ) ) ;
#1723=CARTESIAN_POINT ( 'NONE',  ( -0.1787899950787401604, -1.632997983977269030, -0.07405724077823318263 ) ) ;
#1726=CARTESIAN_POINT ( 'NONE',  ( 0.07405724077823318263, -0.6181102361667089040, 0.1787899950787401604 ) ) ;
#1737=CARTESIAN_POINT ( 'NONE',  ( -0.07405724077823318263, 0.1091280002746981559, 0.1787899950787401604 ) ) ;
#1742=CARTESIAN_POINT ( 'NONE',  ( -0.1574803149606299191, -0.8149606299212598381, 0.000000000000000000 ) ) ;
#1744=CARTESIAN_POINT ( 'NONE',  ( 0.1797182628040039087, -1.514315463126352901, -0.07444174185955065859 ) ) ;
#1746=CARTESIAN_POINT ( 'NONE',  ( -9.642888182262618425E-18, -0.06692913375074074911, -0.1574803149606299191 ) ) ;
#1747=CARTESIAN_POINT ( 'NONE',  ( 0.1113553986120547346, -0.4753937006798740206, 0.1113553986120547346 ) ) ;
#1749=CARTESIAN_POINT ( 'NONE',  ( -0.1264236179284866091, -0.3991141731745826982, -0.1264236179284866091 ) ) ;
#1754=DIRECTION ( 'NONE',  ( 0.000000000000000000, 1.000000000000000000, 0.000000000000000000 ) ) ;
#1758=CARTESIAN_POINT ( 'NONE',  ( 0.1264236179284866091, -0.02017716530056720692, -0.1264236179284866091 ) ) ;
#1768=CARTESIAN_POINT ( 'NONE',  ( 0.1574803149606300301, -1.102854330601134913, 0.06523048226347956391 ) ) ;
#1769=CARTESIAN_POINT ( 'NONE',  ( 0.1787899950787401604, -1.326771653489542402, 0.07405724077823318263 ) ) ;
#1781=CARTESIAN_POINT ( 'NONE',  ( -0.07857503534280656232, -0.08918665060152188018, -0.2400663896720299229 ) ) ;
#1784=CARTESIAN_POINT ( 'NONE',  ( -0.1574803149606299191, -0.1358267715460163283, 0.000000000000000000 ) ) ;
#1789=EDGE_CURVE ( 'NONE', #46167, #19219, #12552, .T. ) ;
#1792=CARTESIAN_POINT ( 'NONE',  ( -0.1264236179284866091, -1.113805070591442847, 0.1264236179284866091 ) ) ;
#1794=CARTESIAN_POINT ( 'NONE',  ( -0.1787899950787401604, -0.03740157474938609478, 0.07405724077823318263 ) ) ;
#1802=CARTESIAN_POINT ( 'NONE',  ( -0.1264236179284866091, -0.5516732282926929409, 0.1264236179284866091 ) ) ;
#1805=CARTESIAN_POINT ( 'NONE',  ( -0.1270800023317771588, -1.216579242653911486, 0.1270800023317771588 ) ) ;
#1806=CARTESIAN_POINT ( 'NONE',  ( 0.1746296719420869226, 0.1299212598425197041, -0.002904701756485846172 ) ) ;
#1822=CARTESIAN_POINT ( 'NONE',  ( 0.1113553986120547346, -1.764763779420031486, -0.1113553986120547346 ) ) ;
#1827=CARTESIAN_POINT ( 'NONE',  ( -0.1787899950787401604, 0.1545275591088816070, -0.07405724077823318263 ) ) ;
#1830=DIRECTION ( 'NONE',  ( 1.000000000000000000, 0.000000000000000000, 0.000000000000000000 ) ) ;
#1833=CARTESIAN_POINT ( 'NONE',  ( -0.1264236179284866091, -1.585137795221826629, -0.1264236179284866091 ) ) ;
#1844=CARTESIAN_POINT ( 'NONE',  ( 3.284318927891251994E-17, -0.7151830233473485121, 0.1787899950787401882 ) ) ;
#1845=CARTESIAN_POINT ( 'NONE',  ( 0.03156423158163212256, -0.08956068939121496209, -0.1858659549881094553 ) ) ;
#1854=CARTESIAN_POINT ( 'NONE',  ( -0.1264236179284866091, -1.496555118056472677, 0.1264236179284866091 ) ) ;
#1859=CARTESIAN_POINT ( 'NONE',  ( 0.07444174185955046430, -0.6826225497405251641, -0.1797182628040039087 ) ) ;
#1864=CARTESIAN_POINT ( 'NONE',  ( 0.1574803149606300301, -0.3646653543307084577, 0.06523048226347956391 ) ) ;
#1887=CARTESIAN_POINT ( 'NONE',  ( 0.07405724077823318263, -1.720472440891118726, 0.1787899950787401604 ) ) ;
#1888=CARTESIAN_POINT ( 'NONE',  ( 0.1264236179284866091, -0.9749015747493857686, 0.1264236179284866091 ) ) ;
#1889=CARTESIAN_POINT ( 'NONE',  ( -0.1574803149606297803, -1.442421259842518566, 0.06523048226347956391 ) ) ;
#1896=CARTESIAN_POINT ( 'NONE',  ( -9.642888182262618425E-18, -1.366141732175937040, -0.1574803149606299191 ) ) ;
#1911=CARTESIAN_POINT ( 'NONE',  ( 0.2063724842062263920, -0.09842519685039370636, -0.01079757893850124065 ) ) ;
#1917=CARTESIAN_POINT ( 'NONE',  ( -0.1264236179284866091, -1.033956692859621995, -0.1264236179284866091 ) ) ;
#1918=CARTESIAN_POINT ( 'NONE',  ( -0.1787899950787401604, -1.262795275536788386, -0.07405724077823318263 ) ) ;
#1921=CARTESIAN_POINT ( 'NONE',  ( 0.1797182628040039087, -0.4906934158822578995, -0.07444174185955065859 ) ) ;
#1922=CARTESIAN_POINT ( 'NONE',  ( -9.642888182262618425E-18, -1.799212598317669443, -0.1574803149606299191 ) ) ;
#1924=CARTESIAN_POINT ( 'NONE',  ( 0.1113553986120547346, -0.01279527559055118092, 0.1113553986120547346 ) ) ;
#1925=CARTESIAN_POINT ( 'NONE',  ( -1.094772975963752103E-17, -0.1727362204186775607, -0.1787899950787401882 ) ) ;
#1931=CARTESIAN_POINT ( 'NONE',  ( -0.1787899950787401604, -0.4015748030958427028, -0.07405724077823318263 ) ) ;
#1933=CARTESIAN_POINT ( 'NONE',  ( 0.1787899950787401604, -1.400590551127339323, 0.07405724077823318263 ) ) ;
#1951=CARTESIAN_POINT ( 'NONE',  ( 0.1251454632067010020, -0.09843574689532874622, -0.1277354705666547130 ) ) ;
#1959=CARTESIAN_POINT ( 'NONE',  ( -0.2191150658379515670, -0.09851385013792676726, 0.09090310240979053436 ) ) ;
#1968=CARTESIAN_POINT ( 'NONE',  ( -0.1787899950787401604, -0.6673228345919050009, 0.07405724077823318263 ) ) ;
#1974=CARTESIAN_POINT ( 'NONE',  ( -0.1787899950787401604, -0.8248031495525351975, 0.07405724077823318263 ) ) ;
#1978=CARTESIAN_POINT ( 'NONE',  ( 0.07405724077823318263, 0.07467918137706039405, 0.1787899950787401604 ) ) ;
#1979=CARTESIAN_POINT ( 'NONE',  ( 0.1787899950787401604, 0.1348425197388028463, -0.07405724077823318263 ) ) ;
#1985=CARTESIAN_POINT ( 'NONE',  ( -0.1113553986120547346, -0.8592519685039370358, -0.1113553986120547346 ) ) ;
#1987=CARTESIAN_POINT ( 'NONE',  ( -0.07444174185955065859, -1.529079242653912152, 0.1797182628040039087 ) ) ;
#1993=CARTESIAN_POINT ( 'NONE',  ( 0.000000000000000000, 0.1299212598425196763, 0.000000000000000000 ) ) ;
#1998=CARTESIAN_POINT ( 'NONE',  ( -0.1264236179284866091, 0.1077755906049446960, -0.1264236179284866091 ) ) ;
#2007=EDGE_CURVE ( 'NONE', #36271, #46609, #4854, .T. ) ;
#2010=CARTESIAN_POINT ( 'NONE',  ( 0.1787899950787401604, -1.361220472387181690, -0.07405724077823318263 ) ) ;
#2012=DIRECTION ( 'NONE',  ( 0.000000000000000000, 1.000000000000000000, 0.000000000000000000 ) ) ;
#2022=CARTESIAN_POINT ( 'NONE',  ( -0.1235961452251415349, -0.09842519685039370636, -0.2140748031496062798 ) ) ;
#2025=CARTESIAN_POINT ( 'NONE',  ( -0.1113553986120547346, -0.2588582676090082635, -0.1113553986120547346 ) ) ;
#2029=CARTESIAN_POINT ( 'NONE',  ( 0.07405724077823318263, -1.106423180827663444, 0.1787899950787401604 ) ) ;
#2031=CARTESIAN_POINT ( 'NONE',  ( 0.1787899950787401604, -0.1013779527021420185, 0.07405724077823318263 ) ) ;
#2037=CARTESIAN_POINT ( 'NONE',  ( 0.1264236179284866091, -0.5713582676627716461, -0.1264236179284866091 ) ) ;
#2040=CARTESIAN_POINT ( 'NONE',  ( -0.07444174185955065859, -1.189512313520053821, -0.1797182628040039087 ) ) ;
#2059=EDGE_CURVE ( 'NONE', #13671, #3164, #7934, .T. ) ;
#2061=CARTESIAN_POINT ( 'NONE',  ( 0.1113553986120547346, -1.695866141624755796, 0.1113553986120547346 ) ) ;
#2066=CARTESIAN_POINT ( 'NONE',  ( 0.1178667752584772188, -0.09842519685039369248, 0.2173826564421467711 ) ) ;
#2067=CARTESIAN_POINT ( 'NONE',  ( 0.1574803149606299191, -1.779527559055118058, -1.928577636452523993E-17 ) ) ;
#2075=CARTESIAN_POINT ( 'NONE',  ( -0.1264236179284866091, -1.703248031442299304, -0.1264236179284866091 ) ) ;
#2083=CARTESIAN_POINT ( 'NONE',  ( -0.05855107416953937022, -0.08956097176436082774, -0.1736406213399021847 ) ) ;
#2084=DIRECTION ( 'NONE',  ( -2.392722035830075028E-16, 0.000000000000000000, -1.000000000000000000 ) ) ;
#2092=CARTESIAN_POINT ( 'NONE',  ( -0.1264236179284866091, -1.545767716481669218, -0.1264236179284866091 ) ) ;
#2095=CARTESIAN_POINT ( 'NONE',  ( 0.1797182628040039087, -0.6924650694255656269, 0.07444174185955046430 ) ) ;
#2099=CARTESIAN_POINT ( 'NONE',  ( 0.1113553986120547346, -0.4360236220472440971, -0.1113553986120547346 ) ) ;
#2100=CARTESIAN_POINT ( 'NONE',  ( -0.06162495753422155692, -0.09842519685039370636, 0.1485290488906215733 ) ) ;
#2103=CARTESIAN_POINT ( 'NONE',  ( -9.642888182262618425E-18, 0.04133858267716535029, -0.1574803149606299191 ) ) ;
#2112=CARTESIAN_POINT ( 'NONE',  ( -0.1264236179284866091, -0.5959645668753701386, -0.1264236179284866091 ) ) ;
#2117=EDGE_CURVE ( 'NONE', #30877, #31109, #35949, .T. ) ;
#2121=CARTESIAN_POINT ( 'NONE',  ( 0.1787899950787401604, -1.789370078686394194, -0.07405724077823318263 ) ) ;
#2122=CARTESIAN_POINT ( 'NONE',  ( -0.1787899950787401882, -1.029035433017102319, 0.000000000000000000 ) ) ;
#2123=CARTESIAN_POINT ( 'NONE',  ( 0.06523048226347956391, -1.393208661417322469, 0.1574803149606297803 ) ) ;
#2142=CARTESIAN_POINT ( 'NONE',  ( -0.07405724077823318263, -0.2452027083867192869, 0.1787899950787401604 ) ) ;
#2144=CARTESIAN_POINT ( 'NONE',  ( -0.02999430697247586555, -0.09842519685039370636, -0.1860644942534716850 ) ) ;
#2150=EDGE_LOOP ( 'NONE', ( #36178, #13805, #10108, #5274 ) ) ;
#2151=CARTESIAN_POINT ( 'NONE',  ( -0.1264236179284866091, -1.102854330654897685, 0.1264236179284866091 ) ) ;
#2152=CARTESIAN_POINT ( 'NONE',  ( 0.1264236179284866091, -1.284940944828125930, 0.1264236179284866091 ) ) ;
#2155=CARTESIAN_POINT ( 'NONE',  ( -0.07444174185955065859, -0.5448272741499744498, 0.1797182628040039087 ) ) ;
#2156=CARTESIAN_POINT ( 'NONE',  ( 0.1574803149606300301, -1.772145669183811334, 0.06523048226347956391 ) ) ;
#2159=CARTESIAN_POINT ( 'NONE',  ( -0.1113553986120547346, 0.04625984251968504046, -0.1113553986120547346 ) ) ;
#2168=CARTESIAN_POINT ( 'NONE',  ( 0.1787899950787401604, -0.6131889763241887836, -0.07405724077823318263 ) ) ;
#2169=CARTESIAN_POINT ( 'NONE',  ( -1.094772975963752103E-17, -1.427657480261196987, -0.1787899950787401882 ) ) ;
#2180=CARTESIAN_POINT ( 'NONE',  ( 0.09061490859345046334, -0.09842521672346266071, -0.1541267623450696400 ) ) ;
#2190=CARTESIAN_POINT ( 'NONE',  ( -0.1222724946009781516, -0.09851384947599900466, 0.1962728965156417260 ) ) ;
#2194=CIRCLE ( 'NONE', #36653, 0.2471922904502826812 ) ;
#2196=CARTESIAN_POINT ( 'NONE',  ( -0.1787899950787401604, -1.628076724134750020, 0.07405724077823318263 ) ) ;
#2199=CARTESIAN_POINT ( 'NONE',  ( 0.1787899950787401604, -0.5738188975840317063, 0.07405724077823318263 ) ) ;
#2204=CARTESIAN_POINT ( 'NONE',  ( -0.1787899950787401604, -0.3572834645131658382, 0.07405724077823318263 ) ) ;
#2205=CARTESIAN_POINT ( 'NONE',  ( -1.094772975963752103E-17, -0.7583661416785196785, -0.1787899950787401882 ) ) ;
#2208=ADVANCED_FACE ( 'NONE', ( #12834 ), #42012, .T. ) ;
#2209=CARTESIAN_POINT ( 'NONE',  ( 0.07405724077823318263, 0.01070280342430459698, -0.1787899950787401604 ) ) ;
#2210=CARTESIAN_POINT ( 'NONE',  ( -0.1787899950787401604, 0.07086614178604697112, -0.07405724077823318263 ) ) ;
#2216=CARTESIAN_POINT ( 'NONE',  ( -0.1574803149606300301, -0.9355314960629919074, -0.06523048226347956391 ) ) ;
#2218=CARTESIAN_POINT ( 'NONE',  ( 0.1270800023317771588, -1.600437510370446681, 0.1270800023317771588 ) ) ;
#2227=CARTESIAN_POINT ( 'NONE',  ( 0.1574803149606300301, -0.8666338581601887858, 0.06523048226347956391 ) ) ;
#2228=CARTESIAN_POINT ( 'NONE',  ( -0.1787899950787401882, 0.03395669296714932950, 0.000000000000000000 ) ) ;
#2232=CARTESIAN_POINT ( 'NONE',  ( 0.1264236179284866091, -0.8518700786863936392, 0.1264236179284866091 ) ) ;
#2239=CARTESIAN_POINT ( 'NONE',  ( -0.1787899950787401604, -1.346456692859623550, -0.07405724077823318263 ) ) ;
#2250=CARTESIAN_POINT ( 'NONE',  ( 0.1264236179284866091, 0.08809055123486594918, 0.1264236179284866091 ) ) ;
#2258=CARTESIAN_POINT ( 'NONE',  ( 0.1787899950787401882, -1.177781448544198639, -2.189545951927503898E-17 ) ) ;
#2260=CARTESIAN_POINT ( 'NONE',  ( -0.07405724077823318263, -0.1899606298674962612, 0.1787899950787401604 ) ) ;
#2270=CARTESIAN_POINT ( 'NONE',  ( -1.094772975963752103E-17, -0.6845472440407243120, -0.1787899950787401882 ) ) ;
#2274=CARTESIAN_POINT ( 'NONE',  ( 0.07444174185955065859, -1.169827274149974894, 0.1797182628040039087 ) ) ;
#2293=CARTESIAN_POINT ( 'NONE',  ( -0.1264236179284866091, 0.1520669291876218521, -0.1264236179284866091 ) ) ;
#2295=CARTESIAN_POINT ( 'NONE',  ( 0.000000000000000000, -0.09842519685039370636, 0.000000000000000000 ) ) ;
#2297=CARTESIAN_POINT ( 'NONE',  ( 0.1908328281150623862, 0.07780450164205171548, 0.1752556861836929991 ) ) ;
#2298=CARTESIAN_POINT ( 'NONE',  ( -0.02442443439252901111, 0.05525422739384169835, 0.2713316170948106287 ) ) ;
#2302=CARTESIAN_POINT ( 'NONE',  ( -0.06523048226347956391, -0.4040354329633388808, 0.1574803149606297803 ) ) ;
#2303=CARTESIAN_POINT ( 'NONE',  ( -0.1264236179284866091, -1.663877952702141672, -0.1264236179284866091 ) ) ;
#2308=CARTESIAN_POINT ( 'NONE',  ( 0.1526800167754713278, 0.1252930045944034287, -0.05620926796873287890 ) ) ;
#2310=CARTESIAN_POINT ( 'NONE',  ( 0.1787899950787401604, -0.6635097950008927992, -0.07405724077823318263 ) ) ;
#2312=CARTESIAN_POINT ( 'NONE',  ( 0.1998254672493015582, -0.08956033089349921261, -0.03070792776777759789 ) ) ;
#2317=CARTESIAN_POINT ( 'NONE',  ( 0.1113553986120547346, 0.07578740157480315376, -0.1113553986120547346 ) ) ;
#2329=CARTESIAN_POINT ( 'NONE',  ( -0.1270800023317771588, -0.7146107387169036151, -0.1270800023317771588 ) ) ;
#2333=CARTESIAN_POINT ( 'NONE',  ( 0.1574803149606299191, -0.4015748031496063630, -1.928577636452523993E-17 ) ) ;
#2334=CARTESIAN_POINT ( 'NONE',  ( -0.1650166048207457326, -0.09842519685039370636, -0.06577345936140498173 ) ) ;
#2343=CARTESIAN_POINT ( 'NONE',  ( -1.094772975963752103E-17, -0.5615157479777322935, -0.1787899950787401882 ) ) ;
#2349=CARTESIAN_POINT ( 'NONE',  ( -0.1787899950787401604, -1.809055118056471123, 0.07405724077823318263 ) ) ;
#2350=CARTESIAN_POINT ( 'NONE',  ( 0.07405724077823318263, -1.134842519631275914, 0.1787899950787401604 ) ) ;
#2351=CARTESIAN_POINT ( 'NONE',  ( -0.1574803149606297803, -1.324311023622046779, 0.06523048226347956391 ) ) ;
#2364=CARTESIAN_POINT ( 'NONE',  ( -0.1898978525284567009, 0.07836113345104847583, 0.1757954945903054400 ) ) ;
#2367=CARTESIAN_POINT ( 'NONE',  ( 0.1787899950787401882, -0.1935294800402626025, -2.189545951927503898E-17 ) ) ;
#2369=B_SPLINE_CURVE_WITH_KNOTS ( 'NONE', 3,
 ( #35071, #9669, #27672, #2450, #46306, #9435, #6043, #38657, #17549, #28125, #42232, #17315, #32187, #13036, #46773, #42684, #13720, #17789, #24511 ),
 .UNSPECIFIED., .F., .F.,
 ( 4, 1, 1, 1, 2, 2, 1, 1, 1, 1, 2, 2, 4 ),
 ( 0.000000000000000000, 0.1250000000000002498, 0.1875000000000002498, 0.2187500000000004163, 0.2343750000000003608, 0.2500000000000002776, 0.3750000000000021094, 0.4375000000000029976, 0.4687500000000034417, 0.4843750000000036082, 0.4921875000000036082, 0.5000000000000035527, 1.000000000000000000 ),
 .UNSPECIFIED. ) ;
#2370=CARTESIAN_POINT ( 'NONE',  ( -0.08392896972913758968, -0.09842519685039370636, 0.2125180856786228201 ) ) ;
#2377=CARTESIAN_POINT ( 'NONE',  ( -0.1787899950787401604, -0.9921259841982054128, -0.07405724077823318263 ) ) ;
#2378=CARTESIAN_POINT ( 'NONE',  ( -0.1264236179284866091, -1.147145669237574772, -0.1264236179284866091 ) ) ;
#2382=CARTESIAN_POINT ( 'NONE',  ( -0.1270800023317771588, -0.4783902662759590974, -0.1270800023317771588 ) ) ;
#2386=CARTESIAN_POINT ( 'NONE',  ( -0.06523048226347956391, 0.04379921259842517456, -0.1574803149606300301 ) ) ;
#2394=VERTEX_POINT ( 'NONE', #24115 ) ;
#2398=CARTESIAN_POINT ( 'NONE',  ( -0.1113553986120547346, -0.9970472439869606518, 0.1113553986120547346 ) ) ;
#2399=CARTESIAN_POINT ( 'NONE',  ( 0.07405724077823318263, -0.5295275590013543976, -0.1787899950787401604 ) ) ;
#2400=CARTESIAN_POINT ( 'NONE',  ( 0.1787899950787401604, -1.321850393647023392, 0.07405724077823318263 ) ) ;
#2403=ORIENTED_EDGE ( 'NONE', *, *, #44041, .F. ) ;
#2407=CARTESIAN_POINT ( 'NONE',  ( 0.1574803149606299191, -1.257874015640503718, -1.928577636452523993E-17 ) ) ;
#2413=CARTESIAN_POINT ( 'NONE',  ( 0.2374471364661455419, -0.04193537623317827867, 0.1483429027091067720 ) ) ;
#2421=CARTESIAN_POINT ( 'NONE',  ( 0.1947686307480071266, -0.09851384395597342913, -0.06118066026927814621 ) ) ;
#2429=CARTESIAN_POINT ( 'NONE',  ( -0.1264236179284866091, -1.556718456418214602, -0.1264236179284866091 ) ) ;
#2431=CARTESIAN_POINT ( 'NONE',  ( 0.1787899950787401604, -0.5344488188438744070, 0.07405724077823318263 ) ) ;
#2434=CARTESIAN_POINT ( 'NONE',  ( 3.284318927891251994E-17, -0.3105314960092286913, 0.1787899950787401882 ) ) ;
#2435=CARTESIAN_POINT ( 'NONE',  ( 0.1787899950787401604, -0.7706692912848194243, 0.07405724077823318263 ) ) ;
#2438=CARTESIAN_POINT ( 'NONE',  ( 0.1264236179284866091, -0.001600346181994637780, 0.1264236179284866091 ) ) ;
#2440=CARTESIAN_POINT ( 'NONE',  ( 0.06828144477518423294, -0.09842519685039377575, 0.1509156562122493384 ) ) ;
#2444=CARTESIAN_POINT ( 'NONE',  ( -0.1113553986120547346, -0.8887795275590552047, 0.1113553986120547346 ) ) ;
#2446=CARTESIAN_POINT ( 'NONE',  ( 0.1797182628040039087, -1.789906014307454551, -0.07444174185955065859 ) ) ;
#2448=CARTESIAN_POINT ( 'NONE',  ( 0.1787899950787401882, -0.3745078739619845942, -2.189545951927503898E-17 ) ) ;
#2450=CARTESIAN_POINT ( 'NONE',  ( 0.1478471407235095458, 0.09575019180979006672, -0.2000734843705069821 ) ) ;
#2455=CARTESIAN_POINT ( 'NONE',  ( -0.1465245066994781686, -0.09658349877441900488, -0.2008369897430446471 ) ) ;
#2456=ORIENTED_EDGE ( 'NONE', *, *, #26497, .T. ) ;
#2459=CARTESIAN_POINT ( 'NONE',  ( -0.1264236179284866091, -0.1579724408911182820, 0.1264236179284866091 ) ) ;
#2461=CARTESIAN_POINT ( 'NONE',  ( -0.1787899950787401882, -0.9453740156942677109, 0.000000000000000000 ) ) ;
#2488=CARTESIAN_POINT ( 'NONE',  ( -0.2471922904502826535, 0.09312491272442048607, -0.03902281811272231143 ) ) ;
#2490=CARTESIAN_POINT ( 'NONE',  ( -0.1264236179284866091, -1.202387747756797243, -0.1264236179284866091 ) ) ;
#2492=CARTESIAN_POINT ( 'NONE',  ( -1.094772975963752103E-17, -0.1284448818360001965, -0.1787899950787401882 ) ) ;
#2502=CARTESIAN_POINT ( 'NONE',  ( 0.1270800023317771588, -0.2618548332050928962, 0.1270800023317771588 ) ) ;
#2503=CARTESIAN_POINT ( 'NONE',  ( -1.094772975963752103E-17, -0.8026574802611967652, -0.1787899950787401882 ) ) ;
#2506=CARTESIAN_POINT ( 'NONE',  ( 0.1270800023317771588, -1.118154045803517738, -0.1270800023317771588 ) ) ;
#2511=DIRECTION ( 'NONE',  ( 0.000000000000000000, 0.000000000000000000, 1.000000000000000000 ) ) ;
#2524=CARTESIAN_POINT ( 'NONE',  ( -0.04517205677937032038, -0.09851383996395098042, -0.1820711016168421181 ) ) ;
#2539=CARTESIAN_POINT ( 'NONE',  ( 0.1787899950787401882, -1.757381889710015965, -2.189545951927503898E-17 ) ) ;
#2545=CARTESIAN_POINT ( 'NONE',  ( -0.07405724077823318263, -0.6782735745284524942, 0.1787899950787401604 ) ) ;
#2547=CARTESIAN_POINT ( 'NONE',  ( -0.1272683714394354237, -0.08956149644601003879, 0.1005630977721749947 ) ) ;
#2552=CARTESIAN_POINT ( 'NONE',  ( 0.06523048226347956391, -0.01525590551181101734, 0.1574803149606297803 ) ) ;
#2560=CARTESIAN_POINT ( 'NONE',  ( 0.1574803149606299191, -0.5984251968503937480, -1.928577636452523993E-17 ) ) ;
#2561=CARTESIAN_POINT ( 'NONE',  ( -0.1275149678065370662, -0.09842519685039370636, 0.1062736314024527728 ) ) ;
#2572=CARTESIAN_POINT ( 'NONE',  ( 0.1787899950787401882, -0.6500984251430865779, -2.189545951927503898E-17 ) ) ;
#2574=VERTEX_POINT ( 'NONE', #1641 ) ;
#2581=CARTESIAN_POINT ( 'NONE',  ( -0.07444174185955065859, 0.07033020616498604494, -0.1797182628040039087 ) ) ;
#2582=CARTESIAN_POINT ( 'NONE',  ( 3.284318927891251994E-17, -1.058562992072220377, 0.1787899950787401882 ) ) ;
#2583=CARTESIAN_POINT ( 'NONE',  ( -0.06523048226347956391, -1.412893700787401174, -0.1574803149606300301 ) ) ;
#2592=CARTESIAN_POINT ( 'NONE',  ( 0.1574803149606299191, -1.415354330601133803, -1.928577636452523993E-17 ) ) ;
#2599=CARTESIAN_POINT ( 'NONE',  ( -0.2471922904502826812, 0.03219022224904106305, 0.1427165354330708902 ) ) ;
#2605=CARTESIAN_POINT ( 'NONE',  ( -0.07405724077823318263, -0.2845727871268765585, 0.1787899950787401604 ) ) ;
#2606=CARTESIAN_POINT ( 'NONE',  ( 0.08207288410471162698, -0.09842519685039370636, -0.1769814723687171687 ) ) ;
#2612=CARTESIAN_POINT ( 'NONE',  ( -0.1264236179284866091, -1.265255905458047225, -0.1264236179284866091 ) ) ;
#2615=CARTESIAN_POINT ( 'NONE',  ( 3.301370929368692659E-17, -0.4636264867484000129, 0.1797182628040039365 ) ) ;
#2620=CARTESIAN_POINT ( 'NONE',  ( -0.06523048226347956391, 0.05856299212598428672, 0.1574803149606297803 ) ) ;
#2621=AXIS2_PLACEMENT_3D ( 'NONE', #28, #28130, #42687 ) ;
#2633=CARTESIAN_POINT ( 'NONE',  ( -0.1264236179284866091, -0.5910433070328504623, 0.1264236179284866091 ) ) ;
#2634=CARTESIAN_POINT ( 'NONE',  ( 0.07405724077823318263, -1.390748031442299082, -0.1787899950787401604 ) ) ;
#2645=CARTESIAN_POINT ( 'NONE',  ( 0.1116671475666351498, -0.09844346291898031787, -0.1397099940965207954 ) ) ;
#2657=CARTESIAN_POINT ( 'NONE',  ( -0.01791479000647193051, -0.09851385005614764212, 0.2243923354945216719 ) ) ;
#2661=CARTESIAN_POINT ( 'NONE',  ( -0.1264236179284866091, -1.714198771378844466, -0.1264236179284866091 ) ) ;
#2662=ORIENTED_EDGE ( 'NONE', *, *, #14716, .F. ) ;
#2663=CARTESIAN_POINT ( 'NONE',  ( 0.07405724077823318263, -0.6574803149068665364, 0.1787899950787401604 ) ) ;
#2668=CARTESIAN_POINT ( 'NONE',  ( 3.284318927891251994E-17, -0.8174212597887557941, 0.1787899950787401882 ) ) ;
#2672=CARTESIAN_POINT ( 'NONE',  ( 0.1787899950787401604, 0.07960044121958026464, 0.07405724077823318263 ) ) ;
#2673=CARTESIAN_POINT ( 'NONE',  ( -0.1787899950787401882, 0.07332677170730689253, 0.000000000000000000 ) ) ;
#2679=CARTESIAN_POINT ( 'NONE',  ( 0.1113553986120547346, -0.8690944881889763884, -0.1113553986120547346 ) ) ;
#2681=CARTESIAN_POINT ( 'NONE',  ( 0.07444174185955046430, -1.666874518244463310, -0.1797182628040039087 ) ) ;
#2682=CARTESIAN_POINT ( 'NONE',  ( -9.642888182262618425E-18, -0.4999999998924724576, -0.1574803149606299191 ) ) ;
#2685=CARTESIAN_POINT ( 'NONE',  ( 0.1787899950787401604, -0.3769685038832444324, 0.07405724077823318263 ) ) ;
#2695=CARTESIAN_POINT ( 'NONE',  ( -0.1787899950787401882, -0.04478346451316559534, 0.000000000000000000 ) ) ;
#2697=CARTESIAN_POINT ( 'NONE',  ( 0.1264236179284866091, -0.8912401574265511606, 0.1264236179284866091 ) ) ;
#2720=CARTESIAN_POINT ( 'NONE',  ( -0.1264236179284866091, -1.192545228071757890, 0.1264236179284866091 ) ) ;
#2722=CARTESIAN_POINT ( 'NONE',  ( 0.1787899950787401604, -0.09645669285962235606, -0.07405724077823318263 ) ) ;
#2728=( BOUNDED_CURVE ( )  B_SPLINE_CURVE ( 2, ( #8770, #42047, #33969 ),
 .UNSPECIFIED., .F., .T. ) 
 B_SPLINE_CURVE_WITH_KNOTS ( ( 3, 3 ),
 ( 0.1350000000000000089, 0.1355626965693000063 ),
 .UNSPECIFIED. ) 
 CURVE ( )  GEOMETRIC_REPRESENTATION_ITEM ( )  RATIONAL_B_SPLINE_CURVE ( ( 1.000000000000000000, 0.9828669096362359081, 0.9734464042078300183 ) ) 
 REPRESENTATION_ITEM ( '' )  ) ;
#2732=CARTESIAN_POINT ( 'NONE',  ( -1.100456976456230270E-17, -1.310083179661785335, -0.1797182628040039365 ) ) ;
#2742=CARTESIAN_POINT ( 'NONE',  ( 0.1264236179284866091, 0.02411417328210995956, -0.1264236179284866091 ) ) ;
#2755=CARTESIAN_POINT ( 'NONE',  ( 0.1574803149606299191, -1.021653543199559033, -1.928577636452523993E-17 ) ) ;
#2760=CARTESIAN_POINT ( 'NONE',  ( 0.07405724077823318263, -0.09153543301710270752, -0.1787899950787401604 ) ) ;
#2764=CARTESIAN_POINT ( 'NONE',  ( 0.1768440709656048937, 0.08559642391441268927, 0.1833320988895605352 ) ) ;
#2770=CARTESIAN_POINT ( 'NONE',  ( -0.07405724077823318263, -1.705708661363559253, -0.1787899950787401604 ) ) ;
#2777=CARTESIAN_POINT ( 'NONE',  ( 0.1787899950787401604, -0.6684310548434121424, 0.07405724077823318263 ) ) ;
#2791=CARTESIAN_POINT ( 'NONE',  ( 0.1270800023317771588, -0.8917760930476122949, 0.1270800023317771588 ) ) ;
#2794=EDGE_CURVE ( 'NONE', #2574, #26779, #4956, .T. ) ;
#2795=CARTESIAN_POINT ( 'NONE',  ( 0.1574803149606300301, -0.6353346456692916533, -0.06523048226347956391 ) ) ;
#2801=CARTESIAN_POINT ( 'NONE',  ( 0.1113553986120547346, -0.6230314959554646981, -0.1113553986120547346 ) ) ;
#2814=CARTESIAN_POINT ( 'NONE',  ( 0.1797182628040039087, 0.1392278439602615547, -0.07444174185955065859 ) ) ;
#2815=CARTESIAN_POINT ( 'NONE',  ( -1.094772975963752103E-17, -1.038877952702141672, -0.1787899950787401882 ) ) ;
#2816=CARTESIAN_POINT ( 'NONE',  ( 0.06523048226347956391, -1.511318897637796255, 0.1574803149606297803 ) ) ;
#2820=VERTEX_POINT ( 'NONE', #24403 ) ;
#2821=CARTESIAN_POINT ( 'NONE',  ( 0.1113553986120547346, -1.410433070758614127, -0.1113553986120547346 ) ) ;
#2830=CARTESIAN_POINT ( 'NONE',  ( -0.1787899950787401604, -0.2156751493316009516, -0.07405724077823318263 ) ) ;
#2838=CARTESIAN_POINT ( 'NONE',  ( 0.07405724077823318263, -1.213582677111591623, 0.1787899950787401604 ) ) ;
#2839=CARTESIAN_POINT ( 'NONE',  ( 0.1787899950787401604, -1.435039370024976391, -0.07405724077823318263 ) ) ;
#2842=CARTESIAN_POINT ( 'NONE',  ( -0.1797182628040039365, -0.4340989276932818997, 0.000000000000000000 ) ) ;
#2859=CARTESIAN_POINT ( 'NONE',  ( -0.1264236179284866091, -0.5123031495525355306, 0.1264236179284866091 ) ) ;
#2860=CARTESIAN_POINT ( 'NONE',  ( 0.1574803149606299191, -1.110236220472440971, -1.928577636452523993E-17 ) ) ;
#2877=CARTESIAN_POINT ( 'NONE',  ( 0.1574803149606300301, -0.1973425195775124208, 0.06523048226347956391 ) ) ;
#2882=CARTESIAN_POINT ( 'NONE',  ( -0.03000208359710393805, -0.09851384112419016292, -0.1860997263723594419 ) ) ;
#2893=CARTESIAN_POINT ( 'NONE',  ( 0.1787899950787401604, -0.2982283464029296116, -0.07405724077823318263 ) ) ;
#2895=CARTESIAN_POINT ( 'NONE',  ( 0.1264236179284866091, -0.7239173227808818334, -0.1264236179284866091 ) ) ;
#2897=CARTESIAN_POINT ( 'NONE',  ( 0.000000000000000000, -0.09842519685039370636, 0.1574803149606299191 ) ) ;
#2900=CARTESIAN_POINT ( 'NONE',  ( -1.094772975963752103E-17, 0.05253351208572189235, -0.1787899950787401882 ) ) ;
#2901=CARTESIAN_POINT ( 'NONE',  ( 0.1787899950787401604, -0.2539370078202523584, -0.07405724077823318263 ) ) ;
#2902=CARTESIAN_POINT ( 'NONE',  ( 0.1787899950787401604, 0.09547244099864542199, -0.07405724077823318263 ) ) ;
#2908=CARTESIAN_POINT ( 'NONE',  ( 0.1574803149606299191, -0.8740157480314961758, -1.928577636452523993E-17 ) ) ;
#2910=CARTESIAN_POINT ( 'NONE',  ( 0.07444174185955046430, -1.745614675724777021, -0.1797182628040039087 ) ) ;
#2919=CARTESIAN_POINT ( 'NONE',  ( 0.1113553986120547346, -0.9084645668216063674, 0.1113553986120547346 ) ) ;
#2920=CARTESIAN_POINT ( 'NONE',  ( -1.094772975963752103E-17, -0.09399606293836239301, -0.1787899950787401882 ) ) ;
#2922=CARTESIAN_POINT ( 'NONE',  ( -0.1787899950787401604, -0.9035433070328510174, 0.07405724077823318263 ) ) ;
#2928=CARTESIAN_POINT ( 'NONE',  ( -0.1113553986120547346, -1.164370078632629868, -0.1113553986120547346 ) ) ;
#2941=CARTESIAN_POINT ( 'NONE',  ( 0.07405724077823318263, -0.07185039364702389131, 0.1787899950787401604 ) ) ;
#2947=CARTESIAN_POINT ( 'NONE',  ( 0.07405724077823318263, -1.484251968450174930, 0.1787899950787401604 ) ) ;
#2950=CARTESIAN_POINT ( 'NONE',  ( 0.07405724077823318263, -1.249139716260735611, -0.1787899950787401604 ) ) ;
#2952=CARTESIAN_POINT ( 'NONE',  ( -0.1787899950787401604, -0.07677165348954355373, 0.07405724077823318263 ) ) ;
#2958=CIRCLE ( 'NONE', #35153, 0.01968503937007875723 ) ;
#2961=CARTESIAN_POINT ( 'NONE',  ( -0.1787899950787401604, -1.499015747977732627, 0.07405724077823318263 ) ) ;
#2962=CARTESIAN_POINT ( 'NONE',  ( 3.284318927891251994E-17, -0.7436023621509606496, 0.1787899950787401882 ) ) ;
#2965=CARTESIAN_POINT ( 'NONE',  ( 0.1270800023317771588, -1.315004439504305012, -0.1270800023317771588 ) ) ;
#2968=VECTOR ( 'NONE', #28083, 39.37007874015748143 ) ;
#2977=CARTESIAN_POINT ( 'NONE',  ( -0.1264236179284866091, -0.005413385773008149403, -0.1264236179284866091 ) ) ;
#2992=CARTESIAN_POINT ( 'NONE',  ( -0.1787899950787401604, -0.002952755851748307785, -0.07405724077823318263 ) ) ;
#2997=CARTESIAN_POINT ( 'NONE',  ( 0.1594274916601849112, 0.09247100924358107876, 0.1933875656399073328 ) ) ;
#3002=CARTESIAN_POINT ( 'NONE',  ( -0.1787899950787401882, -1.658956692859621995, 0.000000000000000000 ) ) ;
#3011=CARTESIAN_POINT ( 'NONE',  ( 0.07405724077823318263, -0.7766987713788455761, -0.1787899950787401604 ) ) ;
#3013=CARTESIAN_POINT ( 'NONE',  ( 0.1020804098320771541, -0.08956209254691890886, 0.1018622834461950927 ) ) ;
#3028=CARTESIAN_POINT ( 'NONE',  ( -0.1797182628040039087, -0.8696304237562747508, -0.07444174185955065859 ) ) ;
#3032=CARTESIAN_POINT ( 'NONE',  ( -0.1113553986120547346, -0.5344488188976378451, 0.1113553986120547346 ) ) ;
#3050=CARTESIAN_POINT ( 'NONE',  ( -0.1270800023317771588, 0.04326327703112763101, 0.1270800023317771588 ) ) ;
#3051=CARTESIAN_POINT ( 'NONE',  ( -0.1787899950787401604, -0.9872047243556864027, 0.07405724077823318263 ) ) ;
#3052=CARTESIAN_POINT ( 'NONE',  ( -0.06523048226347956391, -1.491633858267717549, -0.1574803149606300301 ) ) ;
#3072=CARTESIAN_POINT ( 'NONE',  ( 0.1264236179284866091, -0.2771908973630972661, 0.1264236179284866091 ) ) ;
#3087=CARTESIAN_POINT ( 'NONE',  ( -0.07405724077823318263, -1.193897637741512696, -0.1787899950787401604 ) ) ;
#3088=CARTESIAN_POINT ( 'NONE',  ( -0.07405724077823318263, -1.331692913332063855, 0.1787899950787401604 ) ) ;
#3094=CARTESIAN_POINT ( 'NONE',  ( 0.06523048226347956391, -0.1333661417322835052, 0.1574803149606297803 ) ) ;
#3096=VERTEX_POINT ( 'NONE', #47145 ) ;
#3104=CONICAL_SURFACE ( 'NONE', #11585, 0.2471922904502826812, 0.5235987755982992597 ) ;
#3107=CARTESIAN_POINT ( 'NONE',  ( -0.1574803149606300301, -1.594980314853101877, -0.06523048226347956391 ) ) ;
#3108=CARTESIAN_POINT ( 'NONE',  ( -0.1574803149606297803, -0.9995078739082206010, 0.06523048226347956391 ) ) ;
#3109=CARTESIAN_POINT ( 'NONE',  ( 0.1264236179284866091, -0.5812007873478111097, 0.1264236179284866091 ) ) ;
#3111=CARTESIAN_POINT ( 'NONE',  ( -0.1574803149606300301, -1.014271653543308060, -0.06523048226347956391 ) ) ;
#3119=CARTESIAN_POINT ( 'NONE',  ( -0.06523048226347956391, -1.270177165246803463, 0.1574803149606297803 ) ) ;
#3121=EDGE_CURVE ( 'NONE', #763, #4939, #47422, .T. ) ;
#3126=CARTESIAN_POINT ( 'NONE',  ( 0.1574803149606299191, -0.1555118109160950890, -1.928577636452523993E-17 ) ) ;
#3128=VERTEX_POINT ( 'NONE', #28974 ) ;
#3133=CARTESIAN_POINT ( 'NONE',  ( 0.02145388603015350309, -0.09851384249135294868, -0.1903720119548976408 ) ) ;
#3136=CARTESIAN_POINT ( 'NONE',  ( 3.284318927891251994E-17, -1.699434991851285659, 0.1787899950787401882 ) ) ;
#3144=CARTESIAN_POINT ( 'NONE',  ( 0.07405724077823318263, -0.2687007873478113318, 0.1787899950787401604 ) ) ;
#3146=CARTESIAN_POINT ( 'NONE',  ( -0.1787899950787401604, -0.8641732282926931630, 0.07405724077823318263 ) ) ;
#3151=CARTESIAN_POINT ( 'NONE',  ( -0.07405724077823318263, -0.1812263304339632453, -0.1787899950787401604 ) ) ;
#3152=CARTESIAN_POINT ( 'NONE',  ( -1.094772975963752103E-17, 0.06348425202226751218, -0.1787899950787401882 ) ) ;
#3159=CARTESIAN_POINT ( 'NONE',  ( -0.1270800023317771588, -1.698862707220840429, -0.1270800023317771588 ) ) ;
#3164=VERTEX_POINT ( 'NONE', #21748 ) ;
#3166=CARTESIAN_POINT ( 'NONE',  ( 0.1787899950787401604, -0.06692913380450424277, 0.07405724077823318263 ) ) ;
#3168=CARTESIAN_POINT ( 'NONE',  ( -0.1787899950787401604, -1.100393700733639069, 0.07405724077823318263 ) ) ;
#3177=CARTESIAN_POINT ( 'NONE',  ( -0.1113553986120547346, -1.154527558947590515, 0.1113553986120547346 ) ) ;
#3192=CARTESIAN_POINT ( 'NONE',  ( -0.1787899950787401604, -0.04232283459190575026, 0.07405724077823318263 ) ) ;
#3200=CARTESIAN_POINT ( 'NONE',  ( 0.1264236179284866091, -1.369710582402466681, -0.1264236179284866091 ) ) ;
#3202=CARTESIAN_POINT ( 'NONE',  ( -0.1787899950787401882, -0.2367125983714334636, 0.000000000000000000 ) ) ;
#3206=CARTESIAN_POINT ( 'NONE',  ( -0.2471914725378674960, -0.08966515697905538818, 0.05042473337808872635 ) ) ;
#3209=CARTESIAN_POINT ( 'NONE',  ( -0.07405724077823318263, -1.626968503883244876, -0.1787899950787401604 ) ) ;
#3216=DIRECTION ( 'NONE',  ( 0.000000000000000000, 1.000000000000000000, 0.000000000000000000 ) ) ;
#3219=CARTESIAN_POINT ( 'NONE',  ( -0.1787899950787401604, 0.001968503990771383692, 0.07405724077823318263 ) ) ;
#3229=CARTESIAN_POINT ( 'NONE',  ( 0.1113553986120547346, -1.026574803042078710, 0.1113553986120547346 ) ) ;
#3236=CARTESIAN_POINT ( 'NONE',  ( -0.07405724077823318263, -0.08661417317458304510, -0.1787899950787401604 ) ) ;
#3243=CARTESIAN_POINT ( 'NONE',  ( 0.1350242358428265510, -0.09796987684348243408, -0.2074744707780996344 ) ) ;
#3248=CARTESIAN_POINT ( 'NONE',  ( 0.1264236179284866091, -1.791830708607653699, -0.1264236179284866091 ) ) ;
#3257=CARTESIAN_POINT ( 'NONE',  ( -0.1787899950787401882, -0.8825058579930176172, 0.000000000000000000 ) ) ;
#3260=CARTESIAN_POINT ( 'NONE',  ( -0.1113553986120547346, -0.01279527548302413463, 0.1113553986120547346 ) ) ;
#3274=CARTESIAN_POINT ( 'NONE',  ( -0.07444174185955065859, -0.8597879040712341769, 0.1797182628040039087 ) ) ;
#3278=CARTESIAN_POINT ( 'NONE',  ( -0.1574803149606299191, -0.6574803149606299746, 0.000000000000000000 ) ) ;
#3280=CARTESIAN_POINT ( 'NONE',  ( -9.642888182262618425E-18, 0.1200787401574803237, -0.1574803149606299191 ) ) ;
#3287=CARTESIAN_POINT ( 'NONE',  ( 0.1574803149606299191, -0.6279527557979843744, -1.928577636452523993E-17 ) ) ;
#3291=CARTESIAN_POINT ( 'NONE',  ( -1.094772975963752103E-17, -0.6796259841982046357, -0.1787899950787401882 ) ) ;
#3299=CARTESIAN_POINT ( 'NONE',  ( 0.1270800023317771588, 0.02357823766104893623, -0.1270800023317771588 ) ) ;
#3300=CARTESIAN_POINT ( 'NONE',  ( 0.1264236179284866091, -1.211122047190330786, 0.1264236179284866091 ) ) ;
#3301=CARTESIAN_POINT ( 'NONE',  ( 0.1113553986120547346, -1.548228346456692828, 0.1113553986120547346 ) ) ;
#3308=CARTESIAN_POINT ( 'NONE',  ( 0.1574803149606300301, -1.412893700679873632, -0.06523048226347956391 ) ) ;
#3309=CARTESIAN_POINT ( 'NONE',  ( -0.1264236179284866091, -1.417814960576157635, 0.1264236179284866091 ) ) ;
#3321=CARTESIAN_POINT ( 'NONE',  ( 0.07405724077823318263, -0.3829979839772702510, -0.1787899950787401604 ) ) ;
#3322=CARTESIAN_POINT ( 'NONE',  ( -0.06611196094510747578, -0.09842519685039370636, 0.1467257540889139733 ) ) ;
#3337=CARTESIAN_POINT ( 'NONE',  ( 3.284318927891251994E-17, -1.137303149552535420, 0.1787899950787401882 ) ) ;
#3339=CARTESIAN_POINT ( 'NONE',  ( -0.1264236179284866091, -1.343996062938362268, -0.1264236179284866091 ) ) ;
#3341=CARTESIAN_POINT ( 'NONE',  ( -0.1270800023317771588, -0.5965005024964310509, -0.1270800023317771588 ) ) ;
#3344=CARTESIAN_POINT ( 'NONE',  ( -0.06523048226347956391, -0.1136811023622046890, -0.1574803149606300301 ) ) ;
#3355=CARTESIAN_POINT ( 'NONE',  ( 0.1113553986120547346, -1.567913385719246211, -0.1113553986120547346 ) ) ;
#3356=CARTESIAN_POINT ( 'NONE',  ( 0.1264236179284866091, -0.7386811023084409733, 0.1264236179284866091 ) ) ;
#3358=CARTESIAN_POINT ( 'NONE',  ( 0.1574803149606300301, -1.112696850393701142, 0.06523048226347956391 ) ) ;
#3370=CARTESIAN_POINT ( 'NONE',  ( -0.06523048226347956391, -1.284940944774363158, -0.1574803149606300301 ) ) ;
#3379=CARTESIAN_POINT ( 'NONE',  ( -0.1574803149606300301, -0.2170275589475910150, -0.06523048226347956391 ) ) ;
#3386=CARTESIAN_POINT ( 'NONE',  ( 0.1787899950787401604, -1.765871999725300512, -0.07405724077823318263 ) ) ;
#3391=CARTESIAN_POINT ( 'NONE',  ( -0.1264236179284866091, -0.9502952755367874982, -0.1264236179284866091 ) ) ;
#3396=CARTESIAN_POINT ( 'NONE',  ( 0.1270800023317771588, -0.1732721560397383898, -0.1270800023317771588 ) ) ;
#3397=CARTESIAN_POINT ( 'NONE',  ( -0.1787899950787401604, -0.09756491311112856779, -0.07405724077823318263 ) ) ;
#3398=CARTESIAN_POINT ( 'NONE',  ( 0.07405724077823318263, -0.2883858267178899260, -0.1787899950787401604 ) ) ;
#3399=CARTESIAN_POINT ( 'NONE',  ( -0.1787899950787401882, -0.08415354325332302654, 0.000000000000000000 ) ) ;
#3400=CARTESIAN_POINT ( 'NONE',  ( 0.2471922891335101569, -0.07779967023291604888, -0.07764737426208698223 ) ) ;
#3404=CARTESIAN_POINT ( 'NONE',  ( 0.1235961452251413406, -0.09842519685039370636, 0.2140748031496062798 ) ) ;
#3405=CARTESIAN_POINT ( 'NONE',  ( -0.07444174185955065859, -1.725929636354700536, 0.1797182628040039087 ) ) ;
#3406=CARTESIAN_POINT ( 'NONE',  ( 0.1787899950787401604, -0.4507874015210400209, -0.07405724077823318263 ) ) ;
#3415=CARTESIAN_POINT ( 'NONE',  ( -0.07405724077823318263, -0.07677165348954355373, 0.1787899950787401604 ) ) ;
#3417=CARTESIAN_POINT ( 'NONE',  ( 0.1787899950787401882, -1.043799212544661348, -2.189545951927503898E-17 ) ) ;
#3422=ORIENTED_EDGE ( 'NONE', *, *, #18617, .F. ) ;
#3439=CARTESIAN_POINT ( 'NONE',  ( -0.07405724077823318263, 0.06594488194352732258, -0.1787899950787401604 ) ) ;
#3448=CARTESIAN_POINT ( 'NONE',  ( -1.094772975963752103E-17, -1.364789322559947005, -0.1787899950787401882 ) ) ;
#3450=CARTESIAN_POINT ( 'NONE',  ( -0.07405724077823318263, -0.2834645668753703052, -0.1787899950787401604 ) ) ;
#3454=CARTESIAN_POINT ( 'NONE',  ( -0.2471921892202598448, -0.09660984127287174095, 0.02628542481997977326 ) ) ;
#3459=CARTESIAN_POINT ( 'NONE',  ( 0.1787899950787401882, -1.599901574749385880, -2.189545951927503898E-17 ) ) ;
#3460=CARTESIAN_POINT ( 'NONE',  ( 0.1787899950787401604, -0.7362204723871804690, 0.07405724077823318263 ) ) ;
#3464=CARTESIAN_POINT ( 'NONE',  ( -0.1797182628040039365, -1.260870581236588350, 0.000000000000000000 ) ) ;
#3472=CARTESIAN_POINT ( 'NONE',  ( -0.06523048226347956391, -0.7977362203649133177, 0.1574803149606297803 ) ) ;
#3489=CARTESIAN_POINT ( 'NONE',  ( 0.1264236179284866091, 0.01427165359707059308, 0.1264236179284866091 ) ) ;
#3492=ORIENTED_EDGE ( 'NONE', *, *, #31532, .T. ) ;
#3498=VERTEX_POINT ( 'NONE', #26535 ) ;
#3500=CARTESIAN_POINT ( 'NONE',  ( 0.1787899950787401604, -1.794291338528913426, -0.07405724077823318263 ) ) ;
#3501=AXIS2_PLACEMENT_3D ( 'NONE', #22957, #645, #4726 ) ;
#3509=CARTESIAN_POINT ( 'NONE',  ( -0.1787899950787401882, -0.8037657005127029075, 0.000000000000000000 ) ) ;
#3511=CARTESIAN_POINT ( 'NONE',  ( -0.06523048226347956391, -0.02509842508932336180, -0.1574803149606300301 ) ) ;
#3513=ORIENTED_EDGE ( 'NONE', *, *, #18454, .T. ) ;
#3517=VERTEX_POINT ( 'NONE', #19319 ) ;
#3524=CARTESIAN_POINT ( 'NONE',  ( 0.1797182628040039087, -0.8450241245436764803, -0.07444174185955065859 ) ) ;
#3529=CARTESIAN_POINT ( 'NONE',  ( -9.642888182262618425E-18, -0.5885826771653542844, -0.1574803149606299191 ) ) ;
#3531=CARTESIAN_POINT ( 'NONE',  ( -0.1082836541852444240, 0.1230260985689107939, -0.1186662996108784202 ) ) ;
#3538=CARTESIAN_POINT ( 'NONE',  ( -0.1574803149606299191, -0.6476377951680629685, 0.000000000000000000 ) ) ;
#3543=CARTESIAN_POINT ( 'NONE',  ( -0.1787899950787401604, -0.6279527558517482566, 0.07405724077823318263 ) ) ;
#3549=CARTESIAN_POINT ( 'NONE',  ( 0.1787899950787401604, -1.169291338528914537, 0.07405724077823318263 ) ) ;
#3550=CARTESIAN_POINT ( 'NONE',  ( -0.1113553986120547346, -1.489173228346456712, -0.1113553986120547346 ) ) ;
#3555=CARTESIAN_POINT ( 'NONE',  ( -0.07405724077823318263, -1.415354330654897019, 0.1787899950787401604 ) ) ;
#3558=AXIS2_PLACEMENT_3D ( 'NONE', #20219, #16415, #38686 ) ;
#3561=CARTESIAN_POINT ( 'NONE',  ( -0.2471922904502826535, 0.08969147984774068771, 0.05033842647026517958 ) ) ;
#3565=CARTESIAN_POINT ( 'NONE',  ( -0.1264236179284866091, -0.3657735745284516060, 0.1264236179284866091 ) ) ;
#3569=CARTESIAN_POINT ( 'NONE',  ( 0.2471922904502827645, -0.09842519685039372024, 0.006644306898576237720 ) ) ;
#3573=CARTESIAN_POINT ( 'NONE',  ( 3.284318927891251994E-17, -1.176673228292692830, 0.1787899950787401882 ) ) ;
#3574=CARTESIAN_POINT ( 'NONE',  ( -0.07405724077823318263, -1.425196850339937482, -0.1787899950787401604 ) ) ;
#3578=CARTESIAN_POINT ( 'NONE',  ( 3.301370929368692659E-17, -0.5817367229688724661, 0.1797182628040039365 ) ) ;
#3586=CARTESIAN_POINT ( 'NONE',  ( 0.000000000000000000, -0.09842519685039370636, 0.000000000000000000 ) ) ;
#3592=CARTESIAN_POINT ( 'NONE',  ( 0.1787899950787401604, -1.631889763725764553, -0.07405724077823318263 ) ) ;
#3593=CARTESIAN_POINT ( 'NONE',  ( -0.1113553986120547346, -1.597440944774362048, -0.1113553986120547346 ) ) ;
#3594=CARTESIAN_POINT ( 'NONE',  ( -0.1264236179284866091, -0.7189960629383621571, -0.1264236179284866091 ) ) ;
#3596=CARTESIAN_POINT ( 'NONE',  ( -0.1113553986120547346, -1.046259842519685179, 0.1113553986120547346 ) ) ;
#3615=ORIENTED_EDGE ( 'NONE', *, *, #41505, .T. ) ;
#3619=CARTESIAN_POINT ( 'NONE',  ( -0.04013712062794118351, -0.09851384031509645423, -0.1835615954122362392 ) ) ;
#3622=CARTESIAN_POINT ( 'NONE',  ( 0.1787899950787401604, -1.731423180827664110, 0.07405724077823318263 ) ) ;
#3626=CARTESIAN_POINT ( 'NONE',  ( -0.07405724077823318263, -0.9527559054580476694, -0.1787899950787401604 ) ) ;
#3628=CARTESIAN_POINT ( 'NONE',  ( -0.2471922599940329923, -0.09336655125506164443, -0.03811991455052992500 ) ) ;
#3630=CARTESIAN_POINT ( 'NONE',  ( -0.1797182628040039087, -0.1954178253310769053, 0.07444174185955065859 ) ) ;
#3631=CARTESIAN_POINT ( 'NONE',  ( -0.1787899950787401882, -0.1738444406701836475, 0.000000000000000000 ) ) ;
#3632=CARTESIAN_POINT ( 'NONE',  ( -0.1264236179284866091, -0.3105314960092286913, 0.1264236179284866091 ) ) ;
#3633=CARTESIAN_POINT ( 'NONE',  ( -1.094772975963752103E-17, -0.01525590545804752021, -0.1787899950787401882 ) ) ;
#3636=ADVANCED_FACE ( 'NONE', ( #14019 ), #31615, .T. ) ;
#3640=DIRECTION ( 'NONE',  ( 0.000000000000000000, 1.000000000000000000, 0.000000000000000000 ) ) ;
#3641=CARTESIAN_POINT ( 'NONE',  ( 0.1787899950787401604, -0.4557086613635593086, 0.07405724077823318263 ) ) ;
#3644=CARTESIAN_POINT ( 'NONE',  ( -0.1350242358423168476, -0.09796987684348246184, 0.2074744707784313413 ) ) ;
#3648=CARTESIAN_POINT ( 'NONE',  ( -0.1787899950787401882, -0.2022637794737956740, 0.000000000000000000 ) ) ;
#3651=CARTESIAN_POINT ( 'NONE',  ( 0.1787899950787401882, -1.122539370024976391, -2.189545951927503898E-17 ) ) ;
#3670=CARTESIAN_POINT ( 'NONE',  ( -0.1787899950787401604, 0.07086614178604697112, -0.07405724077823318263 ) ) ;
#3677=CARTESIAN_POINT ( 'NONE',  ( -0.1787899950787401882, -1.236836566654435199, 0.000000000000000000 ) ) ;
#3679=CARTESIAN_POINT ( 'NONE',  ( 0.1787899950787401882, -0.3351377952218271283, -2.189545951927503898E-17 ) ) ;
#3685=CARTESIAN_POINT ( 'NONE',  ( -0.2471922904502826812, -0.03219022224904102836, 0.1427165354330708902 ) ) ;
#3689=CARTESIAN_POINT ( 'NONE',  ( 0.1787899950787401604, -1.602362204670647161, 0.07405724077823318263 ) ) ;
#3690=CARTESIAN_POINT ( 'NONE',  ( 0.1787899950787401882, -1.673720472387181024, -2.189545951927503898E-17 ) ) ;
#3704=CARTESIAN_POINT ( 'NONE',  ( -0.1264236179284866091, 0.1471456693451021758, -0.1264236179284866091 ) ) ;
#3722=CARTESIAN_POINT ( 'NONE',  ( -0.1787899950787401604, -0.1210629920722208208, -0.07405724077823318263 ) ) ;
#3730=CARTESIAN_POINT ( 'NONE',  ( 0.1787899950787401882, -1.796751968450173376, -2.189545951927503898E-17 ) ) ;
#3736=ADVANCED_FACE ( 'NONE', ( #31374 ), #30099, .T. ) ;
#3739=CARTESIAN_POINT ( 'NONE',  ( -0.07405724077823318263, -0.7963838107489246143, 0.1787899950787401604 ) ) ;
#3745=( BOUNDED_CURVE ( )  B_SPLINE_CURVE ( 2, ( #37142, #40012, #44316, #43856, #18462, #22056, #36920, #43377, #43615 ),
 .UNSPECIFIED., .F., .T. ) 
 B_SPLINE_CURVE_WITH_KNOTS ( ( 3, 2, 2, 2, 3 ),
 ( 0.1049999999999999961, 0.1074999999999999983, 0.1100000000000000006, 0.1125000000000000028, 0.1150000000000000050 ),
 .UNSPECIFIED. ) 
 CURVE ( )  GEOMETRIC_REPRESENTATION_ITEM ( )  RATIONAL_B_SPLINE_CURVE ( ( 1.000000000000000000, 0.9238795325112869605, 1.000000000000000000, 0.9238795325112869605, 1.000000000000000000, 0.9238795325112869605, 1.000000000000000000, 0.9238795325112869605, 1.000000000000000000 ) ) 
 REPRESENTATION_ITEM ( '' )  ) ;
#3749=CARTESIAN_POINT ( 'NONE',  ( 0.1264236179284866091, -0.4926181101824567143, -0.1264236179284866091 ) ) ;
#3751=CARTESIAN_POINT ( 'NONE',  ( 0.1270800023317771588, -0.8425634946224153099, -0.1270800023317771588 ) ) ;
#3765=CARTESIAN_POINT ( 'NONE',  ( -0.1264236179284866091, -0.8223425196312754704, 0.1264236179284866091 ) ) ;
#3766=CARTESIAN_POINT ( 'NONE',  ( 0.000000000000000000, 0.0004086818895575684884, 0.000000000000000000 ) ) ;
#3772=CARTESIAN_POINT ( 'NONE',  ( 0.1574803149606299191, -1.582677165354330784, -1.928577636452523993E-17 ) ) ;
#3780=CARTESIAN_POINT ( 'NONE',  ( -0.1787899950787401604, -1.425196850339937482, -0.07405724077823318263 ) ) ;
#3792=CARTESIAN_POINT ( 'NONE',  ( -0.1787899950787401604, -0.3731554642922310649, -0.07405724077823318263 ) ) ;
#3800=CARTESIAN_POINT ( 'NONE',  ( -0.1787899950787401604, -1.302165354276944242, 0.07405724077823318263 ) ) ;
#3802=CARTESIAN_POINT ( 'NONE',  ( 0.07405724077823318263, -1.312007873961984705, -0.1787899950787401604 ) ) ;
#3808=CARTESIAN_POINT ( 'NONE',  ( 0.1574803149606300301, -0.1284448818897638567, 0.06523048226347956391 ) ) ;
#3821=CARTESIAN_POINT ( 'NONE',  ( 0.1264236179284866091, -1.550688976324188895, -0.1264236179284866091 ) ) ;
#3822=CARTESIAN_POINT ( 'NONE',  ( -0.1113553986120547346, -1.479330708553889817, -0.1113553986120547346 ) ) ;
#3823=CARTESIAN_POINT ( 'NONE',  ( -0.1264236179284866091, -0.7091535432533228045, 0.1264236179284866091 ) ) ;
#3825=CARTESIAN_POINT ( 'NONE',  ( 2.892866454678787531E-17, -1.001968503937007871, 0.1574803149606299191 ) ) ;
#3849=CARTESIAN_POINT ( 'NONE',  ( 0.1468505162521946683, -0.09851384555016987066, -0.1345416994043196757 ) ) ;
#3858=CARTESIAN_POINT ( 'NONE',  ( 3.284318927891251994E-17, -0.4286417322297008115, 0.1787899950787401882 ) ) ;
#3859=CARTESIAN_POINT ( 'NONE',  ( 0.1264236179284866091, -0.9601377952218268508, -0.1264236179284866091 ) ) ;
#3864=CARTESIAN_POINT ( 'NONE',  ( 0.07444174185955065859, -0.2643154631263528453, 0.1797182628040039087 ) ) ;
#3865=CARTESIAN_POINT ( 'NONE',  ( 0.1787899950787401882, -0.07541924381978995506, -2.189545951927503898E-17 ) ) ;
#3867=CARTESIAN_POINT ( 'NONE',  ( -1.094772975963752103E-17, -0.05462598419820496182, -0.1787899950787401882 ) ) ;
#3870=CIRCLE ( 'NONE', #45935, 0.2204724409448818867 ) ;
#3875=DIRECTION ( 'NONE',  ( 0.000000000000000000, 0.000000000000000000, 1.000000000000000000 ) ) ;
#3878=CARTESIAN_POINT ( 'NONE',  ( 0.06523048226347956391, -0.9355314959554644760, -0.1574803149606300301 ) ) ;
#3879=CARTESIAN_POINT ( 'NONE',  ( 0.1787899950787401604, -0.3031496062454492879, 0.07405724077823318263 ) ) ;
#3882=CARTESIAN_POINT ( 'NONE',  ( -0.1264236179284866091, -1.097933070812378009, 0.1264236179284866091 ) ) ;
#3886=ORIENTED_EDGE ( 'NONE', *, *, #18130, .T. ) ;
#3898=CARTESIAN_POINT ( 'NONE',  ( -0.1264236179284866091, -0.01033464561552783524, -0.1264236179284866091 ) ) ;
#3907=CARTESIAN_POINT ( 'NONE',  ( -0.1787899950787401604, -1.357407432796167379, -0.07405724077823318263 ) ) ;
#3910=CARTESIAN_POINT ( 'NONE',  ( -0.1787899950787401604, -0.1998031495525358359, -0.07405724077823318263 ) ) ;
#3917=CARTESIAN_POINT ( 'NONE',  ( 0.1264236179284866091, -1.604822834591905556, 0.1264236179284866091 ) ) ;
#3918=CARTESIAN_POINT ( 'NONE',  ( 0.1787899950787401882, -1.634350393647023614, -2.189545951927503898E-17 ) ) ;
#3924=CARTESIAN_POINT ( 'NONE',  ( -0.1797182628040039087, -1.376520187535801520, 0.07444174185955065859 ) ) ;
#3948=CARTESIAN_POINT ( 'NONE',  ( -0.1787899950787401882, -0.1973425196312759700, 0.000000000000000000 ) ) ;
#3951=CARTESIAN_POINT ( 'NONE',  ( 2.892866454678787531E-17, 0.1003937007874015908, 0.1574803149606299191 ) ) ;
#3952=CARTESIAN_POINT ( 'NONE',  ( -0.05612302249891534811, -0.07766248740294821873, 0.2530304272095453277 ) ) ;
#3957=CARTESIAN_POINT ( 'NONE',  ( -0.1787899950787401882, -1.777066929080094670, 0.000000000000000000 ) ) ;
#3960=CIRCLE ( 'NONE', #43844, 0.1574803149606299191 ) ;
#3968=CARTESIAN_POINT ( 'NONE',  ( -0.1264236179284866091, -0.8775845981504979409, 0.1264236179284866091 ) ) ;
#3970=CARTESIAN_POINT ( 'NONE',  ( -0.1787899950787401604, 0.1200787402112438867, 0.07405724077823318263 ) ) ;
#3979=CARTESIAN_POINT ( 'NONE',  ( -0.07444174185955065859, -0.9926619198192657700, -0.1797182628040039087 ) ) ;
#3990=CARTESIAN_POINT ( 'NONE',  ( 0.1787899950787401882, -0.8075787401037164415, -2.189545951927503898E-17 ) ) ;
#3998=CARTESIAN_POINT ( 'NONE',  ( -0.1574803149606297803, -1.599901574803148652, 0.06523048226347956391 ) ) ;
#4004=CARTESIAN_POINT ( 'NONE',  ( -0.07405724077823318263, -1.454724409395055096, 0.1787899950787401604 ) ) ;
#4016=CARTESIAN_POINT ( 'NONE',  ( 0.07405724077823318263, -0.3583916847646721471, 0.1787899950787401604 ) ) ;
#4017=CARTESIAN_POINT ( 'NONE',  ( -0.2061074570449838439, -0.08955986677483838976, 0.1074491168787045231 ) ) ;
#4027=CARTESIAN_POINT ( 'NONE',  ( -1.094772975963752103E-17, -1.314468503883243988, -0.1787899950787401882 ) ) ;
#4028=CARTESIAN_POINT ( 'NONE',  ( -0.1264236179284866091, -1.462106299158834721, -0.1264236179284866091 ) ) ;
#4032=CARTESIAN_POINT ( 'NONE',  ( -0.1797182628040039365, -0.5915792426539113746, 0.000000000000000000 ) ) ;
#4038=CARTESIAN_POINT ( 'NONE',  ( 0.1574803149606300301, -0.3252952755905512694, 0.06523048226347956391 ) ) ;
#4045=CARTESIAN_POINT ( 'NONE',  ( 0.06523048226347956391, -0.5172244093412917687, 0.1574803149606297803 ) ) ;
#4048=CARTESIAN_POINT ( 'NONE',  ( -0.1676346118796341045, -0.08956121678320581869, 0.01619327428367629829 ) ) ;
#4055=CARTESIAN_POINT ( 'NONE',  ( -0.1787899950787401604, -1.499015747977732627, -0.07405724077823318263 ) ) ;
#4056=CARTESIAN_POINT ( 'NONE',  ( 0.1787899950787401604, -0.8149606298674965110, 0.07405724077823318263 ) ) ;
#4057=CARTESIAN_POINT ( 'NONE',  ( 0.1113553986120547346, -1.154527559055118058, 0.1113553986120547346 ) ) ;
#4074=CARTESIAN_POINT ( 'NONE',  ( 0.09432024557780893659, 0.09445537554013619386, 0.2309772516917621976 ) ) ;
#4080=CARTESIAN_POINT ( 'NONE',  ( -0.03607162715213074744, -0.09851382849536771680, 0.1546661156032805018 ) ) ;
#4084=CARTESIAN_POINT ( 'NONE',  ( -0.07405724077823318263, -0.8248031495525351975, 0.1787899950787401604 ) ) ;
#4085=CARTESIAN_POINT ( 'NONE',  ( 0.1787899950787401604, -0.4163385826234020093, -0.07405724077823318263 ) ) ;
#4086=CARTESIAN_POINT ( 'NONE',  ( -0.1787899950787401604, -0.9822834645131651721, 0.07405724077823318263 ) ) ;
#4087=CARTESIAN_POINT ( 'NONE',  ( 0.1270800023317771588, -0.2126422347798960499, -0.1270800023317771588 ) ) ;
#4088=CARTESIAN_POINT ( 'NONE',  ( -0.1574803149606299191, 0.1299212598425196763, 0.000000000000000000 ) ) ;
#4090=CARTESIAN_POINT ( 'NONE',  ( 0.07405724077823318263, -0.01771653537930735489, -0.1787899950787401604 ) ) ;
#4107=CARTESIAN_POINT ( 'NONE',  ( -0.1574803149606300301, -0.9650590550105839771, -0.06523048226347956391 ) ) ;
#4108=CARTESIAN_POINT ( 'NONE',  ( -0.1264236179284866091, -0.2760826771115909573, 0.1264236179284866091 ) ) ;
#4110=CARTESIAN_POINT ( 'NONE',  ( 0.1264236179284866091, -1.284940944828125930, 0.1264236179284866091 ) ) ;
#4135=CARTESIAN_POINT ( 'NONE',  ( 0.1264236179284866091, -1.409080661142624091, -0.1264236179284866091 ) ) ;
#4139=CARTESIAN_POINT ( 'NONE',  ( -0.07405724077823318263, -0.3474409448281265411, 0.1787899950787401604 ) ) ;
#4146=CARTESIAN_POINT ( 'NONE',  ( 3.284318927891251994E-17, -1.688484251914740275, 0.1787899950787401882 ) ) ;
#4147=CARTESIAN_POINT ( 'NONE',  ( 0.1787899950787401604, -1.749999999946236340, -0.07405724077823318263 ) ) ;
#4153=CARTESIAN_POINT ( 'NONE',  ( 0.1797182628040039087, -1.401126486748399458, 0.07444174185955046430 ) ) ;
#4158=CONICAL_SURFACE ( 'NONE', #12620, 0.2471922904502826812, 0.5235987755982992597 ) ;
#4171=CARTESIAN_POINT ( 'NONE',  ( 0.1113553986120547346, -0.05216535433070866590, 0.1113553986120547346 ) ) ;
#4173=CARTESIAN_POINT ( 'NONE',  ( -0.07444174185955065859, -0.1117564080082424360, 0.1797182628040039087 ) ) ;
#4179=CARTESIAN_POINT ( 'NONE',  ( 0.1787899950787401604, -0.1751968503399373434, -0.07405724077823318263 ) ) ;
#4182=CARTESIAN_POINT ( 'NONE',  ( -0.05264611394417081230, -0.07553294269950990014, 0.2550375247538705925 ) ) ;
#4184=CARTESIAN_POINT ( 'NONE',  ( 0.1787899950787401604, -1.799212598371432659, 0.07405724077823318263 ) ) ;
#4192=CARTESIAN_POINT ( 'NONE',  ( -0.1787899950787401882, -0.9612460154733326601, 0.000000000000000000 ) ) ;
#4194=CARTESIAN_POINT ( 'NONE',  ( -0.1787899950787401604, 0.1545275591088816070, -0.07405724077823318263 ) ) ;
#4200=CARTESIAN_POINT ( 'NONE',  ( 0.1787899950787401882, -0.4975393700249764461, -2.189545951927503898E-17 ) ) ;
#4205=CARTESIAN_POINT ( 'NONE',  ( -0.1797182628040039087, -0.9828194001342275277, 0.07444174185955065859 ) ) ;
#4217=CARTESIAN_POINT ( 'NONE',  ( -0.1787899950787401604, -0.7509842519147402751, -0.07405724077823318263 ) ) ;
#4224=CARTESIAN_POINT ( 'NONE',  ( -0.1113553986120547346, -1.646653543307086798, -0.1113553986120547346 ) ) ;
#4229=CARTESIAN_POINT ( 'NONE',  ( 0.1574803149606300301, -0.3105314959554651977, -0.06523048226347956391 ) ) ;
#4233=CARTESIAN_POINT ( 'NONE',  ( 0.1574803149606299191, -0.03740157469562260112, -1.928577636452523993E-17 ) ) ;
#4237=CARTESIAN_POINT ( 'NONE',  ( -0.1264236179284866091, -0.4543562516938055573, -0.1264236179284866091 ) ) ;
#4238=CARTESIAN_POINT ( 'NONE',  ( -0.2343560426797417495, -0.08955971028938346234, 0.03132653569787429565 ) ) ;
#4242=ORIENTED_EDGE ( 'NONE', *, *, #38095, .T. ) ;
#4247=CARTESIAN_POINT ( 'NONE',  ( -0.1264236179284866091, -1.348917322780881944, -0.1264236179284866091 ) ) ;
#4248=CARTESIAN_POINT ( 'NONE',  ( -0.1787899950787401604, -1.577755905458046115, -0.07405724077823318263 ) ) ;
#4257=CARTESIAN_POINT ( 'NONE',  ( -0.1574803149606297803, -0.2219488188976377896, 0.06523048226347956391 ) ) ;
#4262=ADVANCED_FACE ( 'NONE', ( #39565 ), #35497, .T. ) ;
#4266=CARTESIAN_POINT ( 'NONE',  ( -0.1574803149606300301, -0.5713582676090083190, -0.06523048226347956391 ) ) ;
#4267=CARTESIAN_POINT ( 'NONE',  ( -0.1345756647787081373, -0.08956061689499753009, 0.09177022885256264084 ) ) ;
#4270=AXIS2_PLACEMENT_3D ( 'NONE', #26413, #43887, #40980 ) ;
#4274=CARTESIAN_POINT ( 'NONE',  ( -0.07405724077823318263, -0.7460629920722210429, 0.1787899950787401604 ) ) ;
#4275=CARTESIAN_POINT ( 'NONE',  ( 0.1113553986120547346, -1.193897637795275690, 0.1113553986120547346 ) ) ;
#4280=ORIENTED_EDGE ( 'NONE', *, *, #27532, .F. ) ;
#4299=CARTESIAN_POINT ( 'NONE',  ( -0.02050768364047031445, -0.09851382972412085770, 0.1561483119320291324 ) ) ;
#4304=EDGE_CURVE ( 'NONE', #24004, #44436, #35757, .T. ) ;
#4306=CARTESIAN_POINT ( 'NONE',  ( 3.284318927891251994E-17, -0.9010826771115905132, 0.1787899950787401882 ) ) ;
#4307=CARTESIAN_POINT ( 'NONE',  ( 0.1787899950787401882, -0.3794291338045042705, -2.189545951927503898E-17 ) ) ;
#4308=CARTESIAN_POINT ( 'NONE',  ( -0.1787899950787401604, -1.144685039316316599, -0.07405724077823318263 ) ) ;
#4311=CARTESIAN_POINT ( 'NONE',  ( 3.301370929368692659E-17, -0.3455162505279275598, 0.1797182628040039365 ) ) ;
#4312=CARTESIAN_POINT ( 'NONE',  ( 0.1574803149606300301, 0.1077755905511811885, 0.06523048226347956391 ) ) ;
#4316=SURFACE_STYLE_USAGE ( .BOTH. , #8166 ) ;
#4325=CARTESIAN_POINT ( 'NONE',  ( 3.284318927891251994E-17, -0.2317913385289138151, 0.1787899950787401882 ) ) ;
#4327=CARTESIAN_POINT ( 'NONE',  ( 0.1787899950787401882, -1.240649606245448622, -2.189545951927503898E-17 ) ) ;
#4337=CARTESIAN_POINT ( 'NONE',  ( -0.07262103558693376593, -0.09842518455345698747, -0.1633777802328124917 ) ) ;
#4354=CARTESIAN_POINT ( 'NONE',  ( 0.1264236179284866091, -1.497663338307978487, 0.1264236179284866091 ) ) ;
#4356=CARTESIAN_POINT ( 'NONE',  ( 0.1787899950787401882, -0.3745078739619845942, -2.189545951927503898E-17 ) ) ;
#4368=CARTESIAN_POINT ( 'NONE',  ( -0.1264236179284866091, 0.1361949294085564865, -0.1264236179284866091 ) ) ;
#4369=CARTESIAN_POINT ( 'NONE',  ( -0.1264236179284866091, -1.698326771599779628, -0.1264236179284866091 ) ) ;
#4373=CARTESIAN_POINT ( 'NONE',  ( -0.1113553986120547346, -0.8198818897637795144, -0.1113553986120547346 ) ) ;
#4375=CARTESIAN_POINT ( 'NONE',  ( 0.07444174185955046430, -1.351913888323203139, -0.1797182628040039087 ) ) ;
#4383=CARTESIAN_POINT ( 'NONE',  ( 0.1113553986120547346, -0.8297244093412913246, 0.1113553986120547346 ) ) ;
#4398=CARTESIAN_POINT ( 'NONE',  ( 0.07444174185955065859, -0.02809499068540773775, 0.1797182628040039087 ) ) ;
#4401=CARTESIAN_POINT ( 'NONE',  ( 0.1264236179284866091, -1.240649606245448622, -0.1264236179284866091 ) ) ;
#4406=CARTESIAN_POINT ( 'NONE',  ( -0.2471922904502826812, -0.03219022224904102836, 0.1427165354330708902 ) ) ;
#4408=CARTESIAN_POINT ( 'NONE',  ( 0.1787899950787401604, -0.1013779527021420185, 0.07405724077823318263 ) ) ;
#4414=CARTESIAN_POINT ( 'NONE',  ( 0.1113553986120547346, 0.006889763887054606122, -0.1113553986120547346 ) ) ;
#4420=CARTESIAN_POINT ( 'NONE',  ( -0.1787899950787401882, -0.9218759367331751386, 0.000000000000000000 ) ) ;
#4422=CARTESIAN_POINT ( 'NONE',  ( -0.1264236179284866091, 0.03395669296714932950, -0.1264236179284866091 ) ) ;
#4423=ORIENTED_EDGE ( 'NONE', *, *, #15019, .T. ) ;
#4432=CARTESIAN_POINT ( 'NONE',  ( 0.1270800023317771588, -1.049256408008242270, 0.1270800023317771588 ) ) ;
#4443=CARTESIAN_POINT ( 'NONE',  ( 3.284318927891251994E-17, -0.7386811023084409733, 0.1787899950787401882 ) ) ;
#4449=CARTESIAN_POINT ( 'NONE',  ( 0.1113553986120547346, -1.666338582677165503, 0.1113553986120547346 ) ) ;
#4456=CARTESIAN_POINT ( 'NONE',  ( 0.1787899950787401604, -1.479330708607653699, -0.07405724077823318263 ) ) ;
#4463=CARTESIAN_POINT ( 'NONE',  ( 0.000000000000000000, 0.09842519685039370636, 0.000000000000000000 ) ) ;
#4464=CARTESIAN_POINT ( 'NONE',  ( 0.05613986198065472333, 0.07767250275969861395, -0.2530207064393421579 ) ) ;
#4466=CARTESIAN_POINT ( 'NONE',  ( 3.284318927891251994E-17, -0.5183326296465614602, 0.1787899950787401882 ) ) ;
#4467=CARTESIAN_POINT ( 'NONE',  ( 0.06899553503110708585, -0.09842519685039370636, 0.1342099080972281588 ) ) ;
#4473=CARTESIAN_POINT ( 'NONE',  ( -0.07405724077823318263, -1.780635779252860651, 0.1787899950787401604 ) ) ;
#4478=ORIENTED_EDGE ( 'NONE', *, *, #27532, .T. ) ;
#4479=CARTESIAN_POINT ( 'NONE',  ( -0.07405724077823318263, -1.312007873961984705, -0.1787899950787401604 ) ) ;
#4480=CARTESIAN_POINT ( 'NONE',  ( 0.1787899950787401604, -1.592519684985606254, -0.07405724077823318263 ) ) ;
#4488=CARTESIAN_POINT ( 'NONE',  ( -0.1574803149606300301, -0.3056102362204722867, -0.06523048226347956391 ) ) ;
#4495=AXIS2_PLACEMENT_3D ( 'NONE', #30589, #15731, #19531 ) ;
#4500=CARTESIAN_POINT ( 'NONE',  ( -0.1564850196914947811, -0.08956157248042134755, 0.05474941646345270196 ) ) ;
#4505=CARTESIAN_POINT ( 'NONE',  ( -0.09216395708618665972, 0.09383642490574134465, -0.2322221854328508361 ) ) ;
#4507=CARTESIAN_POINT ( 'NONE',  ( 0.07405724077823318263, -1.548228346402928723, -0.1787899950787401604 ) ) ;
#4508=CARTESIAN_POINT ( 'NONE',  ( -0.1113553986120547346, -1.006889763672000004, -0.1113553986120547346 ) ) ;
#4509=CARTESIAN_POINT ( 'NONE',  ( -0.07405724077823318263, -0.9429133857730090940, 0.1787899950787401604 ) ) ;
#4535=CARTESIAN_POINT ( 'NONE',  ( -0.2333336438806818958, -0.09842519685039370636, 0.05221132881278717219 ) ) ;
#4547=CARTESIAN_POINT ( 'NONE',  ( -0.07405724077823318263, -0.9035433070328510174, 0.1787899950787401604 ) ) ;
#4548=CARTESIAN_POINT ( 'NONE',  ( 0.1264236179284866091, -1.088090551127338657, 0.1264236179284866091 ) ) ;
#4550=CARTESIAN_POINT ( 'NONE',  ( 0.07444174185955046430, -0.3282918410791086927, -0.1797182628040039087 ) ) ;
#4551=CARTESIAN_POINT ( 'NONE',  ( 0.1113553986120547346, 0.1446850393700787329, 0.1113553986120547346 ) ) ;
#4564=CARTESIAN_POINT ( 'NONE',  ( 0.1787899950787401604, -0.2982283464029296116, -0.07405724077823318263 ) ) ;
#4567=CARTESIAN_POINT ( 'NONE',  ( 3.284318927891251994E-17, -1.289862204670645607, 0.1787899950787401882 ) ) ;
#4579=CARTESIAN_POINT ( 'NONE',  ( 0.02733683484473901221, -0.09840216969744279563, -0.1767045507392152881 ) ) ;
#4597=CARTESIAN_POINT ( 'NONE',  ( -0.1787899950787401604, -1.436147590276483088, -0.07405724077823318263 ) ) ;
#4600=CARTESIAN_POINT ( 'NONE',  ( -0.1787899950787401882, -0.4335629920722205433, 0.000000000000000000 ) ) ;
#4606=CARTESIAN_POINT ( 'NONE',  ( -0.07405724077823318263, -0.2342519684501733479, 0.1787899950787401604 ) ) ;
#4609=CARTESIAN_POINT ( 'NONE',  ( 0.1264236179284866091, -1.713090551127338657, -0.1264236179284866091 ) ) ;
#4610=CARTESIAN_POINT ( 'NONE',  ( 0.1787899950787401882, -1.713090551127338657, -2.189545951927503898E-17 ) ) ;
#4612=CARTESIAN_POINT ( 'NONE',  ( 0.1781957201322358353, -0.09842519685039370636, -0.01456528979491370120 ) ) ;
#4614=CARTESIAN_POINT ( 'NONE',  ( 0.1574803149606300301, -0.6747047244094498408, -0.06523048226347956391 ) ) ;
#4616=CARTESIAN_POINT ( 'NONE',  ( -1.100456976456230270E-17, -1.428193415882257788, -0.1797182628040039365 ) ) ;
#4618=CARTESIAN_POINT ( 'NONE',  ( 0.2471922904502825702, 0.09210780053718577165, -0.04262551151394824989 ) ) ;
#4622=CARTESIAN_POINT ( 'NONE',  ( 0.1235961452251413406, 0.09842519685039370636, 0.2140748031496062798 ) ) ;
#4632=CARTESIAN_POINT ( 'NONE',  ( -9.642888182262618425E-18, 0.01181102372957427288, -0.1574803149606299191 ) ) ;
#4638=VERTEX_POINT ( 'NONE', #27368 ) ;
#4643=CARTESIAN_POINT ( 'NONE',  ( -1.100456976456230270E-17, -0.08961073871690393433, -0.1797182628040039365 ) ) ;
#4645=CARTESIAN_POINT ( 'NONE',  ( -0.06523048226347956391, -1.048720472333417142, -0.1574803149606300301 ) ) ;
#4646=CARTESIAN_POINT ( 'NONE',  ( 0.07405724077823318263, -1.238188976324190005, -0.1787899950787401604 ) ) ;
#4661=CARTESIAN_POINT ( 'NONE',  ( 0.06523048226347956391, -0.1235236219397170543, 0.1574803149606297803 ) ) ;
#4666=CARTESIAN_POINT ( 'NONE',  ( -0.03598878106637547203, -0.09842522444525984848, 0.1542999736886214723 ) ) ;
#4667=CARTESIAN_POINT ( 'NONE',  ( -0.07405724077823318263, -1.007997983977270140, -0.1787899950787401604 ) ) ;
#4669=CARTESIAN_POINT ( 'NONE',  ( 0.1787899950787401882, 0.01919291343959027632, -2.189545951927503898E-17 ) ) ;
#4670=VERTEX_POINT ( 'NONE', #5519 ) ;
#4680=CARTESIAN_POINT ( 'NONE',  ( 0.1797182628040039087, -1.007425699346825576, 0.07444174185955046430 ) ) ;
#4695=CARTESIAN_POINT ( 'NONE',  ( -0.07405724077823318263, -0.7952755904974174728, -0.1787899950787401604 ) ) ;
#4699=CARTESIAN_POINT ( 'NONE',  ( -0.1574803149606299191, -1.553149606191686960, 0.000000000000000000 ) ) ;
#4704=CARTESIAN_POINT ( 'NONE',  ( -9.642888182262618425E-18, -1.612204724409448842, -0.1574803149606299191 ) ) ;
#4712=CARTESIAN_POINT ( 'NONE',  ( -0.1264236179284866091, -1.457185039316315045, 0.1264236179284866091 ) ) ;
#4722=CARTESIAN_POINT ( 'NONE',  ( 3.284318927891251994E-17, -0.4789625509064039943, 0.1787899950787401882 ) ) ;
#4723=CARTESIAN_POINT ( 'NONE',  ( -0.1723604372983632005, -0.08955946469359528372, -0.1761694098153657739 ) ) ;
#4724=CARTESIAN_POINT ( 'NONE',  ( 0.06523048226347956391, 0.04872047254847189368, -0.1574803149606300301 ) ) ;
#4726=DIRECTION ( 'NONE',  ( 0.000000000000000000, 0.000000000000000000, 1.000000000000000000 ) ) ;
#4729=CARTESIAN_POINT ( 'NONE',  ( 0.2471922927914619317, -0.07821957050365321851, 0.07683452368278725908 ) ) ;
#4732=CARTESIAN_POINT ( 'NONE',  ( -0.1264236179284866091, -1.388287401521039355, -0.1264236179284866091 ) ) ;
#4733=CARTESIAN_POINT ( 'NONE',  ( 0.07405724077823318263, -1.508858267662772867, -0.1787899950787401604 ) ) ;
#4740=CARTESIAN_POINT ( 'NONE',  ( 0.1574803149606299191, -0.3228346456692913757, -1.928577636452523993E-17 ) ) ;
#4753=CARTESIAN_POINT ( 'NONE',  ( -0.1622643153356901069, -0.08956225154872389516, 0.03952951923502038417 ) ) ;
#4762=CARTESIAN_POINT ( 'NONE',  ( 0.1787899950787401604, -1.676181102308441639, 0.07405724077823318263 ) ) ;
#4763=CARTESIAN_POINT ( 'NONE',  ( -0.07405724077823318263, -0.8789370078202529690, -0.1787899950787401604 ) ) ;
#4764=CARTESIAN_POINT ( 'NONE',  ( 0.06523048226347956391, -1.275098425196850016, 0.1574803149606297803 ) ) ;
#4786=CARTESIAN_POINT ( 'NONE',  ( 0.1048411618717816907, -0.09851382789342855162, 0.1042575923466826787 ) ) ;
#4790=EDGE_CURVE ( 'NONE', #40254, #11736, #43157, .T. ) ;
#4792=ORIENTED_EDGE ( 'NONE', *, *, #11592, .T. ) ;
#4793=CARTESIAN_POINT ( 'NONE',  ( -1.094772975963752103E-17, -0.9601377952218268508, -0.1787899950787401882 ) ) ;
#4794=CARTESIAN_POINT ( 'NONE',  ( -0.07405724077823318263, -1.095472440891117838, 0.1787899950787401604 ) ) ;
#4796=CARTESIAN_POINT ( 'NONE',  ( 0.1270800023317771588, -0.3307524710003684754, -0.1270800023317771588 ) ) ;
#4805=DIRECTION ( 'NONE',  ( -0.4999999999999998890, 0.000000000000000000, -0.8660254037844388186 ) ) ;
#4814=CARTESIAN_POINT ( 'NONE',  ( -0.07405724077823318263, -0.3671259841982050798, -0.1787899950787401604 ) ) ;
#4816=CARTESIAN_POINT ( 'NONE',  ( -1.094772975963752103E-17, -1.230807086560409269, -0.1787899950787401882 ) ) ;
#4825=CARTESIAN_POINT ( 'NONE',  ( -0.08205013688028725549, -0.09842440306376359915, -0.1588770961503328805 ) ) ;
#4841=CARTESIAN_POINT ( 'NONE',  ( -1.094772975963752103E-17, -1.443529480040261825, -0.1787899950787401882 ) ) ;
#4844=CARTESIAN_POINT ( 'NONE',  ( 0.1264236179284866091, -0.4876968503399370380, -0.1264236179284866091 ) ) ;
#4854=( BOUNDED_CURVE ( )  B_SPLINE_CURVE ( 2, ( #3951, #583, #18575, #26267, #11879, #40130, #15240, #44661, #29429 ),
 .UNSPECIFIED., .F., .T. ) 
 B_SPLINE_CURVE_WITH_KNOTS ( ( 3, 2, 2, 2, 3 ),
 ( 0.03500000000000000333, 0.03749999999999999861, 0.04000000000000000083, 0.04250000000000000305, 0.04499999999999999833 ),
 .UNSPECIFIED. ) 
 CURVE ( )  GEOMETRIC_REPRESENTATION_ITEM ( )  RATIONAL_B_SPLINE_CURVE ( ( 1.000000000000000000, 0.9238795325112869605, 1.000000000000000000, 0.9238795325112869605, 1.000000000000000000, 0.9238795325112869605, 1.000000000000000000, 0.9238795325112869605, 1.000000000000000000 ) ) 
 REPRESENTATION_ITEM ( '' )  ) ;
#4856=CARTESIAN_POINT ( 'NONE',  ( 0.1787899950787401604, -1.720472440891118726, 0.07405724077823318263 ) ) ;
#4857=CARTESIAN_POINT ( 'NONE',  ( 0.1784937925128310954, -0.09842519685039369248, -0.001216461463074396381 ) ) ;
#4860=CARTESIAN_POINT ( 'NONE',  ( -0.1574803149606297803, -0.7337598425196847352, 0.06523048226347956391 ) ) ;
#4862=CARTESIAN_POINT ( 'NONE',  ( -0.1270800023317771588, -1.423272156039738112, -0.1270800023317771588 ) ) ;
#4863=CARTESIAN_POINT ( 'NONE',  ( -0.1574803149606297803, -0.05462598414444141959, 0.06523048226347956391 ) ) ;
#4864=CARTESIAN_POINT ( 'NONE',  ( 0.2471922904502826257, 0.09255273792768259344, -0.04108768875596677250 ) ) ;
#4873=CARTESIAN_POINT ( 'NONE',  ( -0.07405724077823318263, 0.04133858273092887170, 0.1787899950787401604 ) ) ;
#4876=EDGE_CURVE ( 'NONE', #5551, #2820, #1062, .T. ) ;
#4887=CARTESIAN_POINT ( 'NONE',  ( 0.1270800023317771588, -0.06500443950430531692, 0.1270800023317771588 ) ) ;
#4889=CARTESIAN_POINT ( 'NONE',  ( -0.1264236179284866091, -1.260334645615527549, 0.1264236179284866091 ) ) ;
#4899=ORIENTED_EDGE ( 'NONE', *, *, #26845, .F. ) ;
#4901=AXIS2_PLACEMENT_3D ( 'NONE', #46697, #39274, #32111 ) ;
#4903=CARTESIAN_POINT ( 'NONE',  ( -0.1113553986120547346, -0.02263779516806350284, -0.1113553986120547346 ) ) ;
#4910=CARTESIAN_POINT ( 'NONE',  ( 3.284318927891251994E-17, -0.9120334170481357861, 0.1787899950787401882 ) ) ;
#4912=CARTESIAN_POINT ( 'NONE',  ( -0.07405724077823318263, -0.007874015694267993623, -0.1787899950787401604 ) ) ;
#4921=CARTESIAN_POINT ( 'NONE',  ( 0.1264236179284866091, -0.6993110235682834519, 0.1264236179284866091 ) ) ;
#4925=CARTESIAN_POINT ( 'NONE',  ( 0.1270800023317771588, -0.9705162505279271157, 0.1270800023317771588 ) ) ;
#4933=CARTESIAN_POINT ( 'NONE',  ( 0.1113553986120547346, -0.6722440943806614611, 0.1113553986120547346 ) ) ;
#4934=CARTESIAN_POINT ( 'NONE',  ( 0.1787899950787401604, 0.06102362210100767403, -0.07405724077823318263 ) ) ;
#4937=CARTESIAN_POINT ( 'NONE',  ( 0.1264236179284866091, -0.9699803149068660924, 0.1264236179284866091 ) ) ;
#4939=VERTEX_POINT ( 'NONE', #33306 ) ;
#4941=CARTESIAN_POINT ( 'NONE',  ( 0.1781957201322358353, -0.09842519685039370636, -0.01456528979491370120 ) ) ;
#4942=CARTESIAN_POINT ( 'NONE',  ( 0.1574803149606300301, -1.614665354223181470, 0.06523048226347956391 ) ) ;
#4951=CARTESIAN_POINT ( 'NONE',  ( -1.094772975963752103E-17, -1.550688976324188895, -0.1787899950787401882 ) ) ;
#4956=B_SPLINE_CURVE_WITH_KNOTS ( 'NONE', 3,
 ( #30676, #22501, #19135, #37842, #16048, #1159, #26834, #5000, #45237, #19380, #44526, #12461, #8836, #11742, #1389, #15579, #22982, #41154, #8591, #15101, #4267, #19618, #12210, #30441, #11979, #41391, #37347, #37592, #29980, #37118, #33800, #919, #30217, #26362, #34258, #4500, #41629, #4753, #8117, #23471, #15814, #29746, #40922, #4048, #22742, #33326, #44996, #44291, #8357, #11495, #26115, #18900, #44762, #33554, #672, #15327, #26600, #38073, #38782, #38548, #23941, #31381, #16514, #42806, #28020, #5712, #17207, #9792, #23696, #5228, #5937, #20329, #20559, #5477, #35201, #31846 ),
 .UNSPECIFIED., .F., .F.,
 ( 4, 2, 2, 1, 1, 1, 1, 1, 2, 2, 2, 2, 2, 2, 2, 2, 2, 2, 1, 1, 2, 2, 2, 2, 1, 1, 2, 2, 2, 2, 1, 1, 1, 1, 2, 2, 2, 2, 2, 1, 1, 1, 2, 2, 2, 4 ),
 ( 0.000000000000000000, 0.06249999999999453215, 0.09374999999999182598, 0.1093749999999904104, 0.1171874999999898137, 0.1210937499999895361, 0.1230468749999893002, 0.1240234374999892725, 0.1245117187499892586, 0.1249999999999892308, 0.1874999999999879263, 0.2187499999999873157, 0.2343749999999871214, 0.2421874999999870104, 0.2499999999999868994, 0.3124999999999853451, 0.3437499999999846789, 0.3593749999999843459, 0.3671874999999841238, 0.3710937499999840128, 0.3730468749999839573, 0.3749999999999839018, 0.4374999999999833467, 0.4687499999999831246, 0.4843749999999830136, 0.4921874999999829026, 0.4960937499999828471, 0.4999999999999827915, 0.5624999999999827915, 0.5937499999999826805, 0.6093749999999826805, 0.6171874999999826805, 0.6210937499999826805, 0.6230468749999826805, 0.6240234374999826805, 0.6249999999999826805, 0.6874999999999852340, 0.7187499999999866773, 0.7343749999999872324, 0.7421874999999875655, 0.7460937499999876765, 0.7480468749999877875, 0.7490234374999877875, 0.7499999999999877875, 0.8749999999999938938, 1.000000000000000000 ),
 .UNSPECIFIED. ) ;
#4962=CARTESIAN_POINT ( 'NONE',  ( 0.1787899950787401604, -0.6241397162607352778, -0.07405724077823318263 ) ) ;
#4963=CARTESIAN_POINT ( 'NONE',  ( -0.2199481559187673185, -0.08955985715031791750, 0.08004915535381516845 ) ) ;
#4964=CARTESIAN_POINT ( 'NONE',  ( 0.1574803149606299191, 0.04133858278469235842, -1.928577636452523993E-17 ) ) ;
#4971=CARTESIAN_POINT ( 'NONE',  ( -0.1787899950787401604, -1.785557039095380105, 0.07405724077823318263 ) ) ;
#4974=CARTESIAN_POINT ( 'NONE',  ( 0.2471922599940329923, -0.09336655125506174158, 0.03811991455052975847 ) ) ;
#4978=CARTESIAN_POINT ( 'NONE',  ( 0.07405724077823318263, -1.553149606245448178, -0.1787899950787401604 ) ) ;
#4979=CARTESIAN_POINT ( 'NONE',  ( -0.1787899950787401882, -1.575295275536787276, 0.000000000000000000 ) ) ;
#4989=CARTESIAN_POINT ( 'NONE',  ( 0.06523048226347956391, -0.3941929133858267931, -0.1574803149606300301 ) ) ;
#4994=CARTESIAN_POINT ( 'NONE',  ( -0.1368215936367279117, -0.09383385973766106281, -0.1150912892199234677 ) ) ;
#5000=CARTESIAN_POINT ( 'NONE',  ( -0.1047703448690850969, -0.08956136656883036118, 0.1211223604329432629 ) ) ;
#5001=CARTESIAN_POINT ( 'NONE',  ( -1.094772975963752103E-17, -0.5221456692375747721, -0.1787899950787401882 ) ) ;
#5007=CARTESIAN_POINT ( 'NONE',  ( -1.094772975963752103E-17, -1.703248031442299304, -0.1787899950787401882 ) ) ;
#5008=CARTESIAN_POINT ( 'NONE',  ( -0.1787899950787401604, -0.8297244093950564281, 0.07405724077823318263 ) ) ;
#5009=CARTESIAN_POINT ( 'NONE',  ( 0.06523048226347956391, -1.196358267716536306, 0.1574803149606297803 ) ) ;
#5017=CARTESIAN_POINT ( 'NONE',  ( -0.1113553986120547346, -1.390748031388535422, 0.1113553986120547346 ) ) ;
#5031=CARTESIAN_POINT ( 'NONE',  ( -0.2006030091703118190, -0.09842519685039370636, -0.1463775445859769597 ) ) ;
#5039=CARTESIAN_POINT ( 'NONE',  ( -0.1264236179284866091, -0.8666338582139527791, 0.1264236179284866091 ) ) ;
#5040=CARTESIAN_POINT ( 'NONE',  ( 0.1787899950787401604, -1.085629921206079374, 0.07405724077823318263 ) ) ;
#5044=CARTESIAN_POINT ( 'NONE',  ( 3.301370929368692659E-17, -0.3848863292680850257, 0.1797182628040039365 ) ) ;
#5045=CARTESIAN_POINT ( 'NONE',  ( 0.1574803149606300301, -1.811515747923969410, 0.06523048226347956391 ) ) ;
#5047=CARTESIAN_POINT ( 'NONE',  ( 0.1787899950787401604, -0.1801181101824570474, -0.07405724077823318263 ) ) ;
#5048=CIRCLE ( 'NONE', #3558, 0.2471922904502826812 ) ;
#5056=CARTESIAN_POINT ( 'NONE',  ( 0.06523048226347956391, -0.9749015746956224415, -0.1574803149606300301 ) ) ;
#5057=CARTESIAN_POINT ( 'NONE',  ( -0.07405724077823318263, -0.3917322834108032947, 0.1787899950787401604 ) ) ;
#5059=CARTESIAN_POINT ( 'NONE',  ( -0.1787899950787401604, -1.179133858213953001, 0.07405724077823318263 ) ) ;
#5061=EDGE_CURVE ( 'NONE', #36464, #14105, #37111, .T. ) ;
#5069=CARTESIAN_POINT ( 'NONE',  ( -0.07210009817454927916, -0.09842519241363902049, -0.1636076842217463745 ) ) ;
#5083=CARTESIAN_POINT ( 'NONE',  ( 3.284318927891251994E-17, -1.384474361930025932, 0.1787899950787401882 ) ) ;
#5086=CARTESIAN_POINT ( 'NONE',  ( -0.1264236179284866091, -0.3597440944344256208, -0.1264236179284866091 ) ) ;
#5093=CARTESIAN_POINT ( 'NONE',  ( -1.094772975963752103E-17, 0.1312736695660370045, -0.1787899950787401882 ) ) ;
#5094=CARTESIAN_POINT ( 'NONE',  ( 0.07405724077823318263, -1.784448818843874962, -0.1787899950787401604 ) ) ;
#5095=CARTESIAN_POINT ( 'NONE',  ( 0.1564304382124598325, -0.09842519685039370636, 0.07442043211813872960 ) ) ;
#5097=CARTESIAN_POINT ( 'NONE',  ( 0.1574803149606300301, -0.7928149606299216279, -0.06523048226347956391 ) ) ;
#5099=CARTESIAN_POINT ( 'NONE',  ( -0.07444174185955065859, -1.622583179661785779, -0.1797182628040039087 ) ) ;
#5101=CARTESIAN_POINT ( 'NONE',  ( 0.2471922904502826535, 0.09275221067063772751, -0.04038095640780214185 ) ) ;
#5110=CARTESIAN_POINT ( 'NONE',  ( -9.642888182262618425E-18, -0.8543307085538898171, -0.1574803149606299191 ) ) ;
#5111=CARTESIAN_POINT ( 'NONE',  ( 0.1787899950787401882, 0.05364173233722811102, -2.189545951927503898E-17 ) ) ;
#5118=CARTESIAN_POINT ( 'NONE',  ( 0.000000000000000000, 0.1102362204724409434, 0.000000000000000000 ) ) ;
#5121=CARTESIAN_POINT ( 'NONE',  ( 0.06523048226347956391, -1.093011810916094451, -0.1574803149606300301 ) ) ;
#5122=CARTESIAN_POINT ( 'NONE',  ( 0.1787899950787401882, -1.324311023568283341, -2.189545951927503898E-17 ) ) ;
#5133=CARTESIAN_POINT ( 'NONE',  ( -0.01960094289347295154, -0.05179116514251731057, -0.2741164612102225950 ) ) ;
#5138=CARTESIAN_POINT ( 'NONE',  ( 0.1113553986120547346, -0.002952755797984771627, 0.1113553986120547346 ) ) ;
#5148=CARTESIAN_POINT ( 'NONE',  ( 0.1787899950787401604, -0.9833916847646722026, 0.07405724077823318263 ) ) ;
#5150=CARTESIAN_POINT ( 'NONE',  ( 0.1264236179284866091, -0.02509842514308689362, 0.1264236179284866091 ) ) ;
#5156=PRODUCT ( 'Threaded Bushing', 'Threaded Bushing', '', ( #33903 ) ) ;
#5157=CARTESIAN_POINT ( 'NONE',  ( -0.1264236179284866091, -0.6402559054580471143, -0.1264236179284866091 ) ) ;
#5162=CARTESIAN_POINT ( 'NONE',  ( -0.07444174185955065859, -1.110772156039737890, -0.1797182628040039087 ) ) ;
#5170=CARTESIAN_POINT ( 'NONE',  ( -0.06523048226347956391, -0.7337598424121570817, -0.1574803149606300301 ) ) ;
#5179=CARTESIAN_POINT ( 'NONE',  ( -0.1574803149606300301, -1.713090551073575662, -0.06523048226347956391 ) ) ;
#5183=CARTESIAN_POINT ( 'NONE',  ( 0.1121660444095479159, -0.09796987684348244796, 0.2206716537553182755 ) ) ;
#5184=CARTESIAN_POINT ( 'NONE',  ( -0.1787899950787401604, 0.1151574803687242243, -0.07405724077823318263 ) ) ;
#5188=CARTESIAN_POINT ( 'NONE',  ( -0.04878249046419594337, 0.07306521771081592176, 0.2572684868648978385 ) ) ;
#5190=CARTESIAN_POINT ( 'NONE',  ( -0.1787899950787401882, -1.501476377898992354, 0.000000000000000000 ) ) ;
#5197=CARTESIAN_POINT ( 'NONE',  ( 0.1787899950787401604, -0.5453995587804200129, -0.07405724077823318263 ) ) ;
#5198=CARTESIAN_POINT ( 'NONE',  ( 0.1875465240539248013, -0.08956051620222618692, -0.06933865474359547643 ) ) ;
#5204=CARTESIAN_POINT ( 'NONE',  ( 0.1787899950787401882, -1.807702708386720536, -2.189545951927503898E-17 ) ) ;
#5207=CARTESIAN_POINT ( 'NONE',  ( 0.1264236179284866091, -1.476870078686393750, -0.1264236179284866091 ) ) ;
#5211=CARTESIAN_POINT ( 'NONE',  ( -0.1797182628040039087, -0.7072288489531255440, 0.07444174185955065859 ) ) ;
#5215=CARTESIAN_POINT ( 'NONE',  ( -0.1574803149606300301, -0.3843503937007873850, -0.06523048226347956391 ) ) ;
#5228=CARTESIAN_POINT ( 'NONE',  ( -0.1604156661162643716, -0.08956087497259392072, -0.06661183193370925903 ) ) ;
#5229=CARTESIAN_POINT ( 'NONE',  ( 0.1264236179284866091, -0.6058070865604094912, -0.1264236179284866091 ) ) ;
#5239=CARTESIAN_POINT ( 'NONE',  ( 0.1787899950787401604, -1.749999999946236340, -0.07405724077823318263 ) ) ;
#5240=CARTESIAN_POINT ( 'NONE',  ( 0.1787899950787401604, -0.9675196849856075865, -0.07405724077823318263 ) ) ;
#5241=CARTESIAN_POINT ( 'NONE',  ( -9.642888182262618425E-18, -1.415354330708661568, -0.1574803149606299191 ) ) ;
#5253=CARTESIAN_POINT ( 'NONE',  ( 0.1113553986120547346, -0.002952755797984771627, 0.1113553986120547346 ) ) ;
#5267=B_SPLINE_CURVE_WITH_KNOTS ( 'NONE', 3,
 ( #21864, #28848, #3644, #18262, #10619, #32908, #25218, #22980, #39809, #25, #19377, #21624, #1157, #14675, #29347, #11091, #25710, #40281, #7468, #18493, #33146 ),
 .UNSPECIFIED., .F., .F.,
 ( 4, 2, 1, 1, 2, 2, 2, 1, 1, 1, 2, 2, 4 ),
 ( 0.000000000000000000, 0.1250000000000051625, 0.1875000000000077161, 0.2187500000000088540, 0.2343750000000091593, 0.2500000000000094369, 0.3750000000000128786, 0.4375000000000147105, 0.4687500000000155431, 0.4843750000000156541, 0.4921875000000158207, 0.5000000000000159872, 1.000000000000000000 ),
 .UNSPECIFIED. ) ;
#5269=CARTESIAN_POINT ( 'NONE',  ( 0.2073772511631539750, -0.09842519685039548272, 0.004767299578884354530 ) ) ;
#5274=ORIENTED_EDGE ( 'NONE', *, *, #44773, .F. ) ;
#5275=CARTESIAN_POINT ( 'NONE',  ( 0.1787899950787401604, -1.006889763725763220, -0.07405724077823318263 ) ) ;
#5278=CARTESIAN_POINT ( 'NONE',  ( -0.1264236179284866091, -1.137303149552535420, 0.1264236179284866091 ) ) ;
#5280=CARTESIAN_POINT ( 'NONE',  ( 0.07444174185955065859, -0.4217957780869824869, 0.1797182628040039087 ) ) ;
#5282=CARTESIAN_POINT ( 'NONE',  ( -9.642888182262618425E-18, 0.001968503937007873988, -0.1574803149606299191 ) ) ;
#5290=CARTESIAN_POINT ( 'NONE',  ( -1.094772975963752103E-17, -0.4876968503399370380, -0.1787899950787401882 ) ) ;
#5292=CARTESIAN_POINT ( 'NONE',  ( 0.1787899950787401882, -1.437499999946236340, -2.189545951927503898E-17 ) ) ;
#5300=CARTESIAN_POINT ( 'NONE',  ( -0.1113553986120547346, -1.243110236112944689, -0.1113553986120547346 ) ) ;
#5303=CARTESIAN_POINT ( 'NONE',  ( 0.07763954121060755165, -0.09842560762780139250, -0.1611213105868851969 ) ) ;
#5318=CARTESIAN_POINT ( 'NONE',  ( 0.07405724077823318263, -1.564100346181993562, -0.1787899950787401604 ) ) ;
#5326=CARTESIAN_POINT ( 'NONE',  ( -0.1787899950787401604, -1.774606299158834277, 0.07405724077823318263 ) ) ;
#5327=CARTESIAN_POINT ( 'NONE',  ( -0.1787899950787401604, -1.774606299158834277, -0.07405724077823318263 ) ) ;
#5332=CARTESIAN_POINT ( 'NONE',  ( 2.892866454678787531E-17, -0.6870078740157480324, 0.1574803149606299191 ) ) ;
#5333=CARTESIAN_POINT ( 'NONE',  ( -8.354793841626791791E-17, 0.03219022224904082713, -0.2854330708661417804 ) ) ;
#5334=CARTESIAN_POINT ( 'NONE',  ( 0.1797182628040039087, -1.593055620606666389, -0.07444174185955065859 ) ) ;
#5337=CARTESIAN_POINT ( 'NONE',  ( 0.1264236179284866091, -0.4089566928596221063, -0.1264236179284866091 ) ) ;
#5342=DIRECTION ( 'NONE',  ( 0.000000000000000000, 0.000000000000000000, 1.000000000000000000 ) ) ;
#5345=CARTESIAN_POINT ( 'NONE',  ( -0.1787899950787401882, 0.1126968504474643862, 0.000000000000000000 ) ) ;
#5355=B_SPLINE_CURVE_WITH_KNOTS ( 'NONE', 3,
 ( #14980, #7524, #6812, #32491, #21191, #22143, #28665, #36770, #21683, #35825, #11377, #18550, #29634, #10674 ),
 .UNSPECIFIED., .F., .F.,
 ( 4, 2, 2, 2, 2, 2, 4 ),
 ( 0.000000000000000000, 0.001154605602278699957, 0.001731908403418049936, 0.002309211204557399914, 0.003463816806836099438, 0.004041119607975449633, 0.004618422409114799829 ),
 .UNSPECIFIED. ) ;
#5358=CARTESIAN_POINT ( 'NONE',  ( -0.1574803149606300301, -1.083169291231055986, -0.06523048226347956391 ) ) ;
#5359=CARTESIAN_POINT ( 'NONE',  ( 0.1787899950787401604, -1.321850393647023392, -0.07405724077823318263 ) ) ;
#5372=CARTESIAN_POINT ( 'NONE',  ( -0.1121660444094383646, -0.09796987684348240633, -0.2206716537553740642 ) ) ;
#5374=CARTESIAN_POINT ( 'NONE',  ( 0.1574803149606300301, -0.03494094477436274909, -0.06523048226347956391 ) ) ;
#5381=CARTESIAN_POINT ( 'NONE',  ( 0.1264236179284866091, -1.212230267441836595, -0.1264236179284866091 ) ) ;
#5383=CARTESIAN_POINT ( 'NONE',  ( -0.07405724077823318263, -0.03248031490686641154, 0.1787899950787401604 ) ) ;
#5384=ORIENTED_EDGE ( 'NONE', *, *, #13323, .T. ) ;
#5390=CARTESIAN_POINT ( 'NONE',  ( -0.1787899950787401604, -0.5935039369541101895, 0.07405724077823318263 ) ) ;
#5393=CARTESIAN_POINT ( 'NONE',  ( 0.1270800023317771588, -1.157524124543675148, -0.1270800023317771588 ) ) ;
#5404=CARTESIAN_POINT ( 'NONE',  ( 3.284318927891251994E-17, 0.08809055123486594918, 0.1787899950787401882 ) ) ;
#5410=ORIENTED_EDGE ( 'NONE', *, *, #13323, .F. ) ;
#5415=CARTESIAN_POINT ( 'NONE',  ( -0.06523048226347956391, -1.718011810916095783, -0.1574803149606300301 ) ) ;
#5422=CARTESIAN_POINT ( 'NONE',  ( 0.1787899950787401604, 0.1003937008411650705, -0.07405724077823318263 ) ) ;
#5423=CARTESIAN_POINT ( 'NONE',  ( -0.2471922904502826812, 0.03219022224904098672, -0.1427165354330708902 ) ) ;
#5429=CARTESIAN_POINT ( 'NONE',  ( -0.06523048226347956391, -0.3794291337507407769, -0.1574803149606300301 ) ) ;
#5430=CARTESIAN_POINT ( 'NONE',  ( 0.1787899950787401882, -1.521161417269070837, -2.189545951927503898E-17 ) ) ;
#5436=AXIS2_PLACEMENT_3D ( 'NONE', #5596, #28136, #39118 ) ;
#5440=CARTESIAN_POINT ( 'NONE',  ( 3.284318927891251994E-17, -0.5577027083867189816, 0.1787899950787401882 ) ) ;
#5441=CARTESIAN_POINT ( 'NONE',  ( 0.09486442506688562426, -0.08956016536800728844, 0.1938892545125885658 ) ) ;
#5453=CARTESIAN_POINT ( 'NONE',  ( 0.07405724077823318263, -1.435039370024976391, -0.1787899950787401604 ) ) ;
#5458=CARTESIAN_POINT ( 'NONE',  ( 3.301370929368692659E-17, -0.6604768804491869538, 0.1797182628040039365 ) ) ;
#5463=CARTESIAN_POINT ( 'NONE',  ( 0.1574803149606300301, -0.3991141732283464694, -0.06523048226347956391 ) ) ;
#5477=CARTESIAN_POINT ( 'NONE',  ( -0.1321454132681490201, -0.08956771084344543332, -0.1191853298852298265 ) ) ;
#5478=CARTESIAN_POINT ( 'NONE',  ( -0.07405724077823318263, -0.5196850393163150450, -0.1787899950787401604 ) ) ;
#5483=CARTESIAN_POINT ( 'NONE',  ( -0.05940473271389184323, 0.07959431159476158812, -0.2511357324426385929 ) ) ;
#5485=CARTESIAN_POINT ( 'NONE',  ( -0.07405724077823318263, -1.686023621993479882, 0.1787899950787401604 ) ) ;
#5486=CARTESIAN_POINT ( 'NONE',  ( 0.1264236179284866091, -0.8567913385289133155, 0.1264236179284866091 ) ) ;
#5488=CARTESIAN_POINT ( 'NONE',  ( 0.1574803149606299191, -1.425196850393700920, -1.928577636452523993E-17 ) ) ;
#5504=CARTESIAN_POINT ( 'NONE',  ( -0.1564664719456511366, 0.09340956239926197224, 0.1950971111691690296 ) ) ;
#5508=CARTESIAN_POINT ( 'NONE',  ( 0.1468252362971212699, -0.09842519685039370636, -0.1345159704478356422 ) ) ;
#5517=CARTESIAN_POINT ( 'NONE',  ( -0.1264236179284866091, -1.073326771599779628, -0.1264236179284866091 ) ) ;
#5518=CARTESIAN_POINT ( 'NONE',  ( -1.094772975963752103E-17, -1.191437007820251859, -0.1787899950787401882 ) ) ;
#5519=CARTESIAN_POINT ( 'NONE',  ( 2.892866454678787531E-17, -0.01771653543307086590, 0.1574803149606299191 ) ) ;
#5520=CARTESIAN_POINT ( 'NONE',  ( -0.1797182628040039087, -0.5152997150948566141, -0.07444174185955065859 ) ) ;
#5521=CARTESIAN_POINT ( 'NONE',  ( -0.1574803149606299191, -1.828740157372787278, 0.000000000000000000 ) ) ;
#5523=CARTESIAN_POINT ( 'NONE',  ( -0.1574803149606300301, 0.009350393700787397108, -0.06523048226347956391 ) ) ;
#5524=CARTESIAN_POINT ( 'NONE',  ( 0.1787899950787401882, -0.1432086613635592531, -2.189545951927503898E-17 ) ) ;
#5531=CARTESIAN_POINT ( 'NONE',  ( 3.284318927891251994E-17, -0.4286417322297008115, 0.1787899950787401882 ) ) ;
#5533=CARTESIAN_POINT ( 'NONE',  ( -0.1787899950787401604, -1.454724409395055096, 0.07405724077823318263 ) ) ;
#5542=CARTESIAN_POINT ( 'NONE',  ( 0.1113553986120547346, -1.223425196742866206, 0.1113553986120547346 ) ) ;
#5546=CARTESIAN_POINT ( 'NONE',  ( 0.09164215658464343328, -0.09842519685974014665, -0.1535173901171399125 ) ) ;
#5551=VERTEX_POINT ( 'NONE', #13241 ) ;
#5555=CARTESIAN_POINT ( 'NONE',  ( 0.09663292179451181407, -0.09851384716521771612, 0.1970772057663724430 ) ) ;
#5559=( BOUNDED_CURVE ( )  B_SPLINE_CURVE ( 2, ( #22000, #18630, #33290, #40651, #4233, #18862, #26796, #45441, #20290 ),
 .UNSPECIFIED., .F., .F. ) 
 B_SPLINE_CURVE_WITH_KNOTS ( ( 3, 2, 2, 2, 3 ),
 ( 0.08500000000000000611, 0.08749999999999999445, 0.08999999999999999667, 0.09249999999999999889, 0.09500000000000000111 ),
 .UNSPECIFIED. ) 
 CURVE ( )  GEOMETRIC_REPRESENTATION_ITEM ( )  RATIONAL_B_SPLINE_CURVE ( ( 1.000000000000000000, 0.9238795325112869605, 1.000000000000000000, 0.9238795325112869605, 1.000000000000000000, 0.9238795325112869605, 1.000000000000000000, 0.9238795325112869605, 1.000000000000000000 ) ) 
 REPRESENTATION_ITEM ( '' )  ) ;
#5561=CARTESIAN_POINT ( 'NONE',  ( -0.1264236179284866091, -1.586246015473332882, 0.1264236179284866091 ) ) ;
#5564=CARTESIAN_POINT ( 'NONE',  ( 3.284318927891251994E-17, -0.5418307086076535883, 0.1787899950787401882 ) ) ;
#5571=CARTESIAN_POINT ( 'NONE',  ( -0.07405724077823318263, -0.8198818897100156322, 0.1787899950787401604 ) ) ;
#5575=CONICAL_SURFACE ( 'NONE', #29350, 0.2471922904502826812, 0.5235987755982992597 ) ;
#5576=CARTESIAN_POINT ( 'NONE',  ( 3.284318927891251994E-17, -0.04589168476467180707, 0.1787899950787401882 ) ) ;
#5577=CARTESIAN_POINT ( 'NONE',  ( 0.07405724077823318263, 0.1397637795813224670, -0.1787899950787401604 ) ) ;
#5583=CARTESIAN_POINT ( 'NONE',  ( 0.06523048226347956391, -0.8272637795275583628, -0.1574803149606300301 ) ) ;
#5585=CARTESIAN_POINT ( 'NONE',  ( -0.07444174185955065859, -1.504472943441313770, -0.1797182628040039087 ) ) ;
#5594=CARTESIAN_POINT ( 'NONE',  ( 0.07405724077823318263, 0.006889763833291078637, 0.1787899950787401604 ) ) ;
#5596=CARTESIAN_POINT ( 'NONE',  ( 0.000000000000000000, -0.09842519685039370636, 0.000000000000000000 ) ) ;
#5606=CARTESIAN_POINT ( 'NONE',  ( 2.892866454678787531E-17, -1.110236220364913429, 0.1574803149606299191 ) ) ;
#5607=CARTESIAN_POINT ( 'NONE',  ( -0.1264236179284866091, -1.378444881836000002, 0.1264236179284866091 ) ) ;
#5618=VERTEX_POINT ( 'NONE', #13928 ) ;
#5623=CARTESIAN_POINT ( 'NONE',  ( 0.1113553986120547346, -0.2391732282389295028, 0.1113553986120547346 ) ) ;
#5628=CARTESIAN_POINT ( 'NONE',  ( -0.1264236179284866091, -1.074434991851285437, 0.1264236179284866091 ) ) ;
#5630=CARTESIAN_POINT ( 'NONE',  ( 0.1787899950787401604, -0.1407480314422995815, 0.07405724077823318263 ) ) ;
#5633=PLANE ( 'NONE',  #8752 ) ;
#5635=ADVANCED_FACE ( 'NONE', ( #33117 ), #26431, .T. ) ;
#5638=CARTESIAN_POINT ( 'NONE',  ( -0.07405724077823318263, -0.6820866141194646959, -0.1787899950787401604 ) ) ;
#5642=CARTESIAN_POINT ( 'NONE',  ( 3.301370929368692659E-17, -1.211657982811391809, 0.1797182628040039365 ) ) ;
#5661=CARTESIAN_POINT ( 'NONE',  ( -0.1113553986120547346, -1.676181102254677091, -0.1113553986120547346 ) ) ;
#5667=CARTESIAN_POINT ( 'NONE',  ( -0.1787899950787401882, 0.1176181102899840625, 0.000000000000000000 ) ) ;
#5671=CARTESIAN_POINT ( 'NONE',  ( -0.06218625040858933445, 0.08128102204192425018, 0.2495298224528491315 ) ) ;
#5674=CARTESIAN_POINT ( 'NONE',  ( 0.1787899950787401882, -1.678641732229700922, -2.189545951927503898E-17 ) ) ;
#5682=CARTESIAN_POINT ( 'NONE',  ( -0.1264236179284866091, -0.6413641257095532566, 0.1264236179284866091 ) ) ;
#5692=CARTESIAN_POINT ( 'NONE',  ( 0.000000000000000000, 0.09842519685039370636, 0.000000000000000000 ) ) ;
#5695=CARTESIAN_POINT ( 'NONE',  ( 0.1787899950787401604, -1.518700787347811554, -0.07405724077823318263 ) ) ;
#5698=CARTESIAN_POINT ( 'NONE',  ( 0.07444174185955065859, -0.7367564080082430467, 0.1797182628040039087 ) ) ;
#5701=CARTESIAN_POINT ( 'NONE',  ( 0.06523048226347956391, -0.4335629921259839814, -0.1574803149606300301 ) ) ;
#5712=CARTESIAN_POINT ( 'NONE',  ( -0.1619057349516830613, -0.08956057142125727066, -0.06208618848698507081 ) ) ;
#5713=CARTESIAN_POINT ( 'NONE',  ( 0.1264236179284866091, -0.6156496062454488438, 0.1264236179284866091 ) ) ;
#5722=CARTESIAN_POINT ( 'NONE',  ( -0.1787899950787401604, -1.651574803095843258, 0.07405724077823318263 ) ) ;
#5723=CARTESIAN_POINT ( 'NONE',  ( 3.284318927891251994E-17, -0.9798228345919054449, 0.1787899950787401882 ) ) ;
#5724=CARTESIAN_POINT ( 'NONE',  ( -0.1574803149606297803, -1.403051181102363154, 0.06523048226347956391 ) ) ;
#5732=CARTESIAN_POINT ( 'NONE',  ( -0.1574803149606297803, -1.353838582569638849, 0.06523048226347956391 ) ) ;
#5746=CARTESIAN_POINT ( 'NONE',  ( -0.009585880836737756955, -0.09842519685039370636, -0.1896059596911200962 ) ) ;
#5757=CARTESIAN_POINT ( 'NONE',  ( 0.07405724077823318263, -1.095472440891117838, 0.1787899950787401604 ) ) ;
#5758=CARTESIAN_POINT ( 'NONE',  ( 0.1787899950787401604, -1.277559055064345861, -0.07405724077823318263 ) ) ;
#5763=CARTESIAN_POINT ( 'NONE',  ( 0.1797182628040039087, -0.4956146757247781309, 0.07444174185955046430 ) ) ;
#5766=CARTESIAN_POINT ( 'NONE',  ( -0.06523048226347956391, -0.03494094488188976416, -0.1574803149606300301 ) ) ;
#5773=CARTESIAN_POINT ( 'NONE',  ( -0.07405724077823318263, -0.6033464566391496531, -0.1787899950787401604 ) ) ;
#5774=CARTESIAN_POINT ( 'NONE',  ( 0.1787899950787401882, -1.398129921206078707, -2.189545951927503898E-17 ) ) ;
#5788=CARTESIAN_POINT ( 'NONE',  ( 0.1003010584927840482, -0.09843450717735198474, -0.1483099721156116158 ) ) ;
#5791=CARTESIAN_POINT ( 'NONE',  ( 0.2137641352132148842, -0.06208088008958128484, 0.1620118252827001948 ) ) ;
#5797=CARTESIAN_POINT ( 'NONE',  ( 0.1225873787495714712, -0.09851384768301142680, 0.1799582249796369826 ) ) ;
#5802=CARTESIAN_POINT ( 'NONE',  ( -0.07405724077823318263, -1.623155464292230565, 0.1787899950787401604 ) ) ;
#5803=ORIENTED_EDGE ( 'NONE', *, *, #30598, .T. ) ;
#5805=CARTESIAN_POINT ( 'NONE',  ( 0.1264236179284866091, -0.5762795275052914334, 0.1264236179284866091 ) ) ;
#5811=CARTESIAN_POINT ( 'NONE',  ( -0.07405724077823318263, -0.2883858267178899260, -0.1787899950787401604 ) ) ;
#5812=CARTESIAN_POINT ( 'NONE',  ( 0.1264236179284866091, -0.7337598424659212970, 0.1264236179284866091 ) ) ;
#5817=CARTESIAN_POINT ( 'NONE',  ( -0.1264236179284866091, 0.06729729161328090736, 0.1264236179284866091 ) ) ;
#5818=CARTESIAN_POINT ( 'NONE',  ( -0.07405724077823318263, 0.1053149606836847191, -0.1787899950787401604 ) ) ;
#5823=CARTESIAN_POINT ( 'NONE',  ( -0.1113553986120547346, -0.8986220472440945573, -0.1113553986120547346 ) ) ;
#5825=CARTESIAN_POINT ( 'NONE',  ( -0.1270800023317771588, -1.570909951315328623, 0.1270800023317771588 ) ) ;
#5827=CARTESIAN_POINT ( 'NONE',  ( 0.07405724077823318263, -0.3818897637257640532, 0.1787899950787401604 ) ) ;
#5835=CARTESIAN_POINT ( 'NONE',  ( 0.1264236179284866091, 0.04872047249470835839, 0.1264236179284866091 ) ) ;
#5836=CARTESIAN_POINT ( 'NONE',  ( 0.07405724077823318263, -0.05216535427694517224, -0.1787899950787401604 ) ) ;
#5838=CARTESIAN_POINT ( 'NONE',  ( 0.07405724077823318263, -0.9330708660879686311, 0.1787899950787401604 ) ) ;
#5847=CARTESIAN_POINT ( 'NONE',  ( -1.094772975963752103E-17, -1.353838582623401621, -0.1787899950787401882 ) ) ;
#5852=EDGE_CURVE ( 'NONE', #2820, #799, #35748, .T. ) ;
#5865=EDGE_CURVE ( 'NONE', #31109, #5618, #25496, .T. ) ;
#5869=CARTESIAN_POINT ( 'NONE',  ( -0.2471922904502826257, 0.07945684066377885213, -0.07439773916327591108 ) ) ;
#5871=CARTESIAN_POINT ( 'NONE',  ( 0.1787899950787401882, -1.138411369804041451, -2.189545951927503898E-17 ) ) ;
#5873=CARTESIAN_POINT ( 'NONE',  ( 0.1787899950787401604, -0.1801181101824570474, 0.07405724077823318263 ) ) ;
#5879=CARTESIAN_POINT ( 'NONE',  ( 0.1264236179284866091, -0.6205708660879685201, 0.1264236179284866091 ) ) ;
#5883=CARTESIAN_POINT ( 'NONE',  ( -0.07444174185955065859, -1.150142234779895745, -0.1797182628040039087 ) ) ;
#5890=DIRECTION ( 'NONE',  ( 0.000000000000000000, 1.000000000000000000, 0.000000000000000000 ) ) ;
#5898=CARTESIAN_POINT ( 'NONE',  ( -0.1113553986120547346, -1.666338582569637738, 0.1113553986120547346 ) ) ;
#5902=CARTESIAN_POINT ( 'NONE',  ( -0.1787899950787401882, 0.07824803154982658271, 0.000000000000000000 ) ) ;
#5905=DIRECTION ( 'NONE',  ( -0.000000000000000000, 1.000000000000000000, 0.000000000000000000 ) ) ;
#5909=CARTESIAN_POINT ( 'NONE',  ( 0.1264236179284866091, -1.752460629867496067, -0.1264236179284866091 ) ) ;
#5930=CARTESIAN_POINT ( 'NONE',  ( 0.06523048226347956391, -0.4876968503937005872, 0.1574803149606297803 ) ) ;
#5931=CARTESIAN_POINT ( 'NONE',  ( 0.000000000000000000, 0.1200787401574803237, 0.000000000000000000 ) ) ;
#5933=CARTESIAN_POINT ( 'NONE',  ( 0.1113553986120547346, 0.02657480314960630058, 0.1113553986120547346 ) ) ;
#5937=CARTESIAN_POINT ( 'NONE',  ( -0.1603352656429097856, -0.08956088745009382901, -0.06684612809662447697 ) ) ;
#5939=CARTESIAN_POINT ( 'NONE',  ( 0.1787899950787401604, -0.5295275590013543976, -0.07405724077823318263 ) ) ;
#5947=CARTESIAN_POINT ( 'NONE',  ( 0.1270800023317771588, 0.06294831640120648886, -0.1270800023317771588 ) ) ;
#5948=CARTESIAN_POINT ( 'NONE',  ( -0.07405724077823318263, -1.100393700733639069, 0.1787899950787401604 ) ) ;
#5949=CARTESIAN_POINT ( 'NONE',  ( 0.06523048226347956391, -1.378444881889764551, -0.1574803149606300301 ) ) ;
#5966=CARTESIAN_POINT ( 'NONE',  ( 0.05636151600968929837, -0.07780576619186881093, -0.2528927375204811923 ) ) ;
#5969=CARTESIAN_POINT ( 'NONE',  ( -0.1264236179284866091, -0.2575058579930181168, -0.1264236179284866091 ) ) ;
#5970=CARTESIAN_POINT ( 'NONE',  ( -0.06937174427877500216, -0.09842519685039370636, -0.1728322085960811161 ) ) ;
#5976=CARTESIAN_POINT ( 'NONE',  ( -0.1264236179284866091, -1.024114173174582643, 0.1264236179284866091 ) ) ;
#5978=CARTESIAN_POINT ( 'NONE',  ( 0.1787899950787401882, -1.240649606245448622, -2.189545951927503898E-17 ) ) ;
#5982=CARTESIAN_POINT ( 'NONE',  ( -0.1270800023317771588, -0.5177603450161165632, -0.1270800023317771588 ) ) ;
#5986=CARTESIAN_POINT ( 'NONE',  ( -0.1574803149606299191, -0.06692913385826770867, 0.000000000000000000 ) ) ;
#5995=CARTESIAN_POINT ( 'NONE',  ( 0.1787899950787401882, -0.6550196849856062542, -2.189545951927503898E-17 ) ) ;
#5997=CARTESIAN_POINT ( 'NONE',  ( 0.07405724077823318263, -1.469488188922614791, -0.1787899950787401604 ) ) ;
#5999=EDGE_CURVE ( 'NONE', #3498, #763, #329, .T. ) ;
#6001=ORIENTED_EDGE ( 'NONE', *, *, #8765, .T. ) ;
#6012=CARTESIAN_POINT ( 'NONE',  ( 0.1594432092295600123, -0.09246610911307991121, 0.1933784749626996369 ) ) ;
#6017=CARTESIAN_POINT ( 'NONE',  ( 0.2010203987887842214, -0.09851384488251044291, -0.04151172976903000356 ) ) ;
#6022=CARTESIAN_POINT ( 'NONE',  ( -0.07405724077823318263, -1.559179086339476550, -0.1787899950787401604 ) ) ;
#6025=CARTESIAN_POINT ( 'NONE',  ( 0.07405724077823318263, -0.5639763778989922427, -0.1787899950787401604 ) ) ;
#6028=CARTESIAN_POINT ( 'NONE',  ( 0.1787899950787401604, -0.7312992125446612368, 0.07405724077823318263 ) ) ;
#6031=CARTESIAN_POINT ( 'NONE',  ( 0.1264236179284866091, 0.008242173503044743221, -0.1264236179284866091 ) ) ;
#6032=CARTESIAN_POINT ( 'NONE',  ( 0.1264236179284866091, 0.08809055123486594918, 0.1264236179284866091 ) ) ;
#6039=CARTESIAN_POINT ( 'NONE',  ( 0.1574803149606299191, -0.9133858267716534751, -1.928577636452523993E-17 ) ) ;
#6041=CARTESIAN_POINT ( 'NONE',  ( 3.301370929368692659E-17, -1.723469006433439032, 0.1797182628040039365 ) ) ;
#6043=CARTESIAN_POINT ( 'NONE',  ( 0.1564664719456493325, 0.09340956239926197224, -0.1950971111691700843 ) ) ;
#6048=CARTESIAN_POINT ( 'NONE',  ( -0.2471922904502826812, -0.03219022224904098672, -0.1427165354330708902 ) ) ;
#6051=CARTESIAN_POINT ( 'NONE',  ( -0.1113553986120547346, -0.8789370077664881986, 0.1113553986120547346 ) ) ;
#6052=CARTESIAN_POINT ( 'NONE',  ( -0.1264236179284866091, -0.1186023621509608300, 0.1264236179284866091 ) ) ;
#6055=CARTESIAN_POINT ( 'NONE',  ( -0.1264236179284866091, -0.9896653542769447975, -0.1264236179284866091 ) ) ;
#6062=CARTESIAN_POINT ( 'NONE',  ( 0.1264236179284866091, -1.358759842465921297, -0.1264236179284866091 ) ) ;
#6079=CARTESIAN_POINT ( 'NONE',  ( 3.284318927891251994E-17, -1.108883810748923171, 0.1787899950787401882 ) ) ;
#6080=VERTEX_POINT ( 'NONE', #9989 ) ;
#6081=CARTESIAN_POINT ( 'NONE',  ( -0.07405724077823318263, -0.1505905511273389341, 0.1787899950787401604 ) ) ;
#6089=CARTESIAN_POINT ( 'NONE',  ( 0.1797182628040039087, -0.1412839670633605771, 0.07444174185955046430 ) ) ;
#6090=CARTESIAN_POINT ( 'NONE',  ( 3.284318927891251994E-17, -0.7829724408911181710, 0.1787899950787401882 ) ) ;
#6093=CARTESIAN_POINT ( 'NONE',  ( 0.1270800023317771588, -1.236264282023989969, -0.1270800023317771588 ) ) ;
#6099=LINE ( 'NONE', #6337, #45249 ) ;
#6105=CARTESIAN_POINT ( 'NONE',  ( -0.07405724077823318263, -0.007874015694267993623, -0.1787899950787401604 ) ) ;
#6109=CIRCLE ( 'NONE', #36747, 0.2471922904502826812 ) ;
#6112=VERTEX_POINT ( 'NONE', #46868 ) ;
#6119=CARTESIAN_POINT ( 'NONE',  ( 0.1787899950787401604, -0.06200787396198446239, 0.07405724077823318263 ) ) ;
#6126=CARTESIAN_POINT ( 'NONE',  ( 0.06523048226347956391, -0.3991141731208192045, 0.1574803149606297803 ) ) ;
#6127=CARTESIAN_POINT ( 'NONE',  ( -1.094772975963752103E-17, -1.668799212544661348, -0.1787899950787401882 ) ) ;
#6136=CARTESIAN_POINT ( 'NONE',  ( -0.02422842392870433459, -0.08956072386513425077, -0.1835680598173657641 ) ) ;
#6146=AXIS2_PLACEMENT_3D ( 'NONE', #1505, #26951, #5342 ) ;
#6155=CARTESIAN_POINT ( 'NONE',  ( 0.2471922904502826812, 0.09842519685039370636, -5.914624404477007554E-17 ) ) ;
#6159=CARTESIAN_POINT ( 'NONE',  ( 0.1574803149606300301, -0.6402559055118107745, 0.06523048226347956391 ) ) ;
#6169=CARTESIAN_POINT ( 'NONE',  ( 2.892866454678787531E-17, -0.5984251967428660945, 0.1574803149606299191 ) ) ;
#6173=CARTESIAN_POINT ( 'NONE',  ( -0.07405724077823318263, -0.6377952755367874982, -0.1787899950787401604 ) ) ;
#6178=CARTESIAN_POINT ( 'NONE',  ( 3.301370929368692659E-17, 0.1269246943539624195, 0.1797182628040039365 ) ) ;
#6179=CARTESIAN_POINT ( 'NONE',  ( 0.1264236179284866091, -1.083169291284818980, -0.1264236179284866091 ) ) ;
#6180=CARTESIAN_POINT ( 'NONE',  ( 2.892866454678787531E-17, -1.395669291338582862, 0.1574803149606299191 ) ) ;
#6194=CARTESIAN_POINT ( 'NONE',  ( -0.2471922904502826535, 0.09842519685039370636, 0.01310751975302586886 ) ) ;
#6196=CARTESIAN_POINT ( 'NONE',  ( -0.1888124183976708226, 0.07899857248962416367, 0.1764221702779021350 ) ) ;
#6199=CARTESIAN_POINT ( 'NONE',  ( 0.008044285442517225965, -0.09842519685039370636, 0.2239033890101252144 ) ) ;
#6203=CARTESIAN_POINT ( 'NONE',  ( 0.1787899950787401882, -1.009350393647023614, -2.189545951927503898E-17 ) ) ;
#6204=CARTESIAN_POINT ( 'NONE',  ( 0.1787899950787401604, -1.243110236166709459, 0.07405724077823318263 ) ) ;
#6208=CARTESIAN_POINT ( 'NONE',  ( -1.100456976456230270E-17, -0.5620516835987936499, -0.1797182628040039365 ) ) ;
#6212=CARTESIAN_POINT ( 'NONE',  ( -0.1574803149606299191, -0.02755905511811023584, 0.000000000000000000 ) ) ;
#6227=CARTESIAN_POINT ( 'NONE',  ( -0.07405724077823318263, -0.5492125983714331028, 0.1787899950787401604 ) ) ;
#6228=CARTESIAN_POINT ( 'NONE',  ( 0.1264236179284866091, -1.393208661363559031, -0.1264236179284866091 ) ) ;
#6233=CARTESIAN_POINT ( 'NONE',  ( -0.1574803149606299191, -1.277559055010582645, 0.000000000000000000 ) ) ;
#6240=ADVANCED_FACE ( 'NONE', ( #33474 ), #40604, .F. ) ;
#6243=CARTESIAN_POINT ( 'NONE',  ( 0.1574803149606300301, -0.08415354330708660346, -0.06523048226347956391 ) ) ;
#6249=CARTESIAN_POINT ( 'NONE',  ( -0.05398180662860094930, -0.09851384891491477003, 0.2205059587191452730 ) ) ;
#6253=CARTESIAN_POINT ( 'NONE',  ( -0.1264236179284866091, -1.635458613898529645, -0.1264236179284866091 ) ) ;
#6255=CARTESIAN_POINT ( 'NONE',  ( -0.1787899950787401882, -0.6304133857730078727, 0.000000000000000000 ) ) ;
#6261=CARTESIAN_POINT ( 'NONE',  ( 0.1787899950787401604, -0.3425196849856064762, 0.07405724077823318263 ) ) ;
#6262=CARTESIAN_POINT ( 'NONE',  ( 0.1787899950787401604, -0.8051181101824581576, -0.07405724077823318263 ) ) ;
#6266=CARTESIAN_POINT ( 'NONE',  ( 0.1787899950787401604, -0.03358853515837262327, -0.07405724077823318263 ) ) ;
#6267=CARTESIAN_POINT ( 'NONE',  ( 0.1264236179284866091, 0.05856299217974780119, -0.1264236179284866091 ) ) ;
#6268=CARTESIAN_POINT ( 'NONE',  ( -0.03598878106637547203, -0.09842522444525984848, 0.1542999736886214723 ) ) ;
#6274=CARTESIAN_POINT ( 'NONE',  ( -0.1113553986120547346, -0.8494094488188976833, 0.1113553986120547346 ) ) ;
#6276=CARTESIAN_POINT ( 'NONE',  ( -0.1797182628040039365, -1.772681604858638016, 0.000000000000000000 ) ) ;
#6278=CARTESIAN_POINT ( 'NONE',  ( -0.1574803149606299191, -0.4901574802074331050, 0.000000000000000000 ) ) ;
#6279=CARTESIAN_POINT ( 'NONE',  ( -0.1787899950787401604, -0.3523622046706461619, 0.07405724077823318263 ) ) ;
#6291=CARTESIAN_POINT ( 'NONE',  ( -0.1787899950787401604, -0.04724409443442544737, -0.07405724077823318263 ) ) ;
#6312=CARTESIAN_POINT ( 'NONE',  ( 0.1264236179284866091, -1.481791338528913426, 0.1264236179284866091 ) ) ;
#6316=CARTESIAN_POINT ( 'NONE',  ( -0.07405724077823318263, -1.165478298937900448, -0.1787899950787401604 ) ) ;
#6318=CARTESIAN_POINT ( 'NONE',  ( 0.07405724077823318263, -0.05216535427694517224, -0.1787899950787401604 ) ) ;
#6329=CARTESIAN_POINT ( 'NONE',  ( -0.1787899950787401882, -0.7534448818360000022, 0.000000000000000000 ) ) ;
#6337=CARTESIAN_POINT ( 'NONE',  ( 0.000000000000000000, -0.09842519685039370636, 0.1574803149606299191 ) ) ;
#6357=CARTESIAN_POINT ( 'NONE',  ( -0.1787899950787401604, -0.04232283459190578495, -0.07405724077823318263 ) ) ;
#6361=CARTESIAN_POINT ( 'NONE',  ( 0.1984097999861146600, 0.07306521771078811067, 0.1708811194342987061 ) ) ;
#6366=CARTESIAN_POINT ( 'NONE',  ( -0.1264236179284866091, -1.742618110182456714, -0.1264236179284866091 ) ) ;
#6371=EDGE_CURVE ( 'NONE', #14105, #28863, #19529, .T. ) ;
#6377=CARTESIAN_POINT ( 'NONE',  ( -0.07405724077823318263, -0.7176436532686085723, 0.1787899950787401604 ) ) ;
#6379=CARTESIAN_POINT ( 'NONE',  ( -0.1238056228176431101, -0.08956144685902442393, 0.1042814069884555189 ) ) ;
#6380=CARTESIAN_POINT ( 'NONE',  ( -0.01196991696110410314, -0.08706565000358124085, 0.1574804073918250613 ) ) ;
#6386=CARTESIAN_POINT ( 'NONE',  ( 0.1574803149606299191, 0.07086614173228346358, -1.928577636452523993E-17 ) ) ;
#6395=CARTESIAN_POINT ( 'NONE',  ( -0.1270800023317771588, -0.7933508961972184359, -0.1270800023317771588 ) ) ;
#6398=CARTESIAN_POINT ( 'NONE',  ( 0.06523048226347956391, -0.6058070866141728184, 0.1574803149606297803 ) ) ;
#6399=CARTESIAN_POINT ( 'NONE',  ( -0.06564852040591530324, 0.1217688336447599051, -0.1452423310039973325 ) ) ;
#6402=CARTESIAN_POINT ( 'NONE',  ( 2.892866454678787531E-17, 0.07086614183981043702, 0.1574803149606299191 ) ) ;
#6415=CARTESIAN_POINT ( 'NONE',  ( 0.1797182628040039365, 0.09739713529884430621, -2.200913952912460540E-17 ) ) ;
#6416=CARTESIAN_POINT ( 'NONE',  ( 0.1264236179284866091, -1.014271653489543290, 0.1264236179284866091 ) ) ;
#6417=CARTESIAN_POINT ( 'NONE',  ( 0.06523048226347956391, -1.575295275590552713, -0.1574803149606300301 ) ) ;
#6424=CARTESIAN_POINT ( 'NONE',  ( 0.1574803149606300301, -1.417814960522395085, 0.06523048226347956391 ) ) ;
#6438=CARTESIAN_POINT ( 'NONE',  ( 0.07405724077823318263, -0.3190216060245144036, 0.1787899950787401604 ) ) ;
#6439=CARTESIAN_POINT ( 'NONE',  ( -0.1204983120504163341, -0.09842519685039370636, -0.1370941885240791192 ) ) ;
#6447=CARTESIAN_POINT ( 'NONE',  ( 0.1787899950787401604, -1.129921259788756682, 0.07405724077823318263 ) ) ;
#6448=CARTESIAN_POINT ( 'NONE',  ( 0.07405724077823318263, -1.193897637741512696, -0.1787899950787401604 ) ) ;
#6450=CARTESIAN_POINT ( 'NONE',  ( 0.1797182628040039087, -0.5743548332050922856, 0.07444174185955046430 ) ) ;
#6453=CARTESIAN_POINT ( 'NONE',  ( -9.642888182262618425E-18, -0.1948818897637795422, -0.1574803149606299191 ) ) ;
#6459=DIRECTION ( 'NONE',  ( 0.000000000000000000, 1.000000000000000000, 0.000000000000000000 ) ) ;
#6466=CARTESIAN_POINT ( 'NONE',  ( 0.07405724077823318263, -0.6230314960092281362, 0.1787899950787401604 ) ) ;
#6467=CARTESIAN_POINT ( 'NONE',  ( 0.1113553986120547346, -0.9970472440944881942, 0.1113553986120547346 ) ) ;
#6475=CARTESIAN_POINT ( 'NONE',  ( 0.1574803149606300301, -1.294783464459401845, -0.06523048226347956391 ) ) ;
#6483=CARTESIAN_POINT ( 'NONE',  ( 0.1113553986120547346, -0.2687007872940476716, -0.1113553986120547346 ) ) ;
#6495=CARTESIAN_POINT ( 'NONE',  ( -1.094772975963752103E-17, -1.719120031221364142, -0.1787899950787401882 ) ) ;
#6501=CARTESIAN_POINT ( 'NONE',  ( 3.284318927891251994E-17, -0.3499015747493862127, 0.1787899950787401882 ) ) ;
#6503=CARTESIAN_POINT ( 'NONE',  ( 0.1264236179284866091, -0.8026574802611967652, -0.1264236179284866091 ) ) ;
#6504=CARTESIAN_POINT ( 'NONE',  ( -0.2471921300642929697, -0.09379707428445160922, -0.03645430680490755609 ) ) ;
#6509=CARTESIAN_POINT ( 'NONE',  ( -0.07405724077823318263, -0.04835231468593165216, 0.1787899950787401604 ) ) ;
#6514=CARTESIAN_POINT ( 'NONE',  ( 0.1113553986120547346, -0.9478346456692913202, -0.1113553986120547346 ) ) ;
#6516=CARTESIAN_POINT ( 'NONE',  ( 3.301370929368692659E-17, -1.684098927693281400, 0.1797182628040039365 ) ) ;
#6517=CARTESIAN_POINT ( 'NONE',  ( 0.1574803149606299191, -0.5098425195775118102, -1.928577636452523993E-17 ) ) ;
#6528=CARTESIAN_POINT ( 'NONE',  ( 0.1574803149606299191, -0.9035433069790866911, -1.928577636452523993E-17 ) ) ;
#6529=CARTESIAN_POINT ( 'NONE',  ( 0.1264236179284866091, -0.1382874015210397711, -0.1264236179284866091 ) ) ;
#6531=CARTESIAN_POINT ( 'NONE',  ( 0.1787899950787401604, -0.9675196849856075865, 0.07405724077823318263 ) ) ;
#6540=CARTESIAN_POINT ( 'NONE',  ( -0.1574803149606297803, -1.156988188868850465, 0.06523048226347956391 ) ) ;
#6553=EDGE_CURVE ( 'NONE', #19219, #46651, #28772, .T. ) ;
#6554=B_SPLINE_CURVE_WITH_KNOTS ( 'NONE', 3,
 ( #33135, #25925, #43644, #32898, #36705, #47004, #16, #263, #32426, #40507, #3400, #14665, #28841, #18011, #29339, #7696, #43400, #39798, #11311, #43883, #25208, #14908, #11083 ),
 .UNSPECIFIED., .F., .F.,
 ( 4, 2, 2, 1, 1, 1, 2, 2, 2, 1, 1, 2, 2, 4 ),
 ( 0.000000000000000000, 0.2499999999999987788, 0.3749999999999982792, 0.4374999999999980571, 0.4687499999999980016, 0.4843749999999980571, 0.4921874999999981126, 0.4999999999999981126, 0.6249999999999982236, 0.6874999999999983347, 0.7187499999999982236, 0.7343749999999983347, 0.7499999999999983347, 1.000000000000000000 ),
 .UNSPECIFIED. ) ;
#6555=CARTESIAN_POINT ( 'NONE',  ( 0.1787899950787401604, -0.06200787396198446239, -0.07405724077823318263 ) ) ;
#6560=CARTESIAN_POINT ( 'NONE',  ( 0.1264236179284866091, -1.471948818843874074, -0.1264236179284866091 ) ) ;
#6563=CARTESIAN_POINT ( 'NONE',  ( 0.1264236179284866091, -1.300812944607191213, 0.1264236179284866091 ) ) ;
#6565=CARTESIAN_POINT ( 'NONE',  ( -0.07405724077823318263, -0.04724409443442544737, -0.1787899950787401604 ) ) ;
#6571=CARTESIAN_POINT ( 'NONE',  ( 0.1787899950787401604, -1.439960629867495401, -0.07405724077823318263 ) ) ;
#6584=CARTESIAN_POINT ( 'NONE',  ( -0.1264236179284866091, 0.004429133912031228346, 0.1264236179284866091 ) ) ;
#6599=CARTESIAN_POINT ( 'NONE',  ( -0.07405724077823318263, 0.04625984257344856188, 0.1787899950787401604 ) ) ;
#6604=CARTESIAN_POINT ( 'NONE',  ( 0.2471922904502826812, 0.03219022224904106305, 0.1427165354330708902 ) ) ;
#6609=CARTESIAN_POINT ( 'NONE',  ( -0.1113553986120547346, -0.4163385825696385711, -0.1113553986120547346 ) ) ;
#6610=CARTESIAN_POINT ( 'NONE',  ( 0.1787899950787401604, -1.641732283410802573, 0.07405724077823318263 ) ) ;
#6615=ADVANCED_FACE ( 'NONE', ( #12181 ), #8565, .F. ) ;
#6620=CARTESIAN_POINT ( 'NONE',  ( 0.07405724077823318263, -0.7127223934260893401, 0.1787899950787401604 ) ) ;
#6622=CARTESIAN_POINT ( 'NONE',  ( -0.07443497905850630925, -0.08956195077354547895, 0.1394259959420596495 ) ) ;
#6631=CARTESIAN_POINT ( 'NONE',  ( -0.07444174185955065859, -0.9139217623389520595, -0.1797182628040039087 ) ) ;
#6632=CARTESIAN_POINT ( 'NONE',  ( 0.2471922904502826257, 0.05203836715086061077, 0.1197978718291115713 ) ) ;
#6635=CARTESIAN_POINT ( 'NONE',  ( -0.06523048226347956391, -0.5319881889763778959, 0.1574803149606297803 ) ) ;
#6654=CARTESIAN_POINT ( 'NONE',  ( 0.000000000000000000, -0.09842519685039370636, 0.000000000000000000 ) ) ;
#6655=CARTESIAN_POINT ( 'NONE',  ( 0.07444174185955046430, 0.1441491038027811755, -0.1797182628040039087 ) ) ;
#6656=CARTESIAN_POINT ( 'NONE',  ( -0.1264236179284866091, -1.102854330654897685, 0.1264236179284866091 ) ) ;
#6657=CARTESIAN_POINT ( 'NONE',  ( 0.1574803149606300301, -1.540846456692913868, -0.06523048226347956391 ) ) ;
#6664=CARTESIAN_POINT ( 'NONE',  ( 0.1113553986120547346, -1.449803149498771759, -0.1113553986120547346 ) ) ;
#6672=CARTESIAN_POINT ( 'NONE',  ( 0.1264236179284866091, -0.2378208186229397725, 0.1264236179284866091 ) ) ;
#6678=VERTEX_POINT ( 'NONE', #38516 ) ;
#6681=CARTESIAN_POINT ( 'NONE',  ( 0.1787899950787401604, -1.361220472387181690, 0.07405724077823318263 ) ) ;
#6683=( CONVERSION_BASED_UNIT ( 'INCH', #46465 ) LENGTH_UNIT ( ) NAMED_UNIT ( #20364 ) ) ;
#6684=CARTESIAN_POINT ( 'NONE',  ( -0.1270800023317771588, -0.6260280615515491087, 0.1270800023317771588 ) ) ;
#6688=CARTESIAN_POINT ( 'NONE',  ( 0.06523048226347956391, -0.1579724409448819422, -0.1574803149606300301 ) ) ;
#6689=ORIENTED_EDGE ( 'NONE', *, *, #16001, .T. ) ;
#6691=ORIENTED_EDGE ( 'NONE', *, *, #380, .F. ) ;
#6707=CARTESIAN_POINT ( 'NONE',  ( -0.06523048226347956391, -1.545767716427905336, 0.1574803149606297803 ) ) ;
#6708=CARTESIAN_POINT ( 'NONE',  ( -0.07405724077823318263, -0.5639763778989922427, -0.1787899950787401604 ) ) ;
#6709=CARTESIAN_POINT ( 'NONE',  ( 0.06523048226347956391, -1.102854330708662456, -0.1574803149606300301 ) ) ;
#6721=CARTESIAN_POINT ( 'NONE',  ( 0.1607876024857142205, -0.09201407021838738098, 0.1926022046198413995 ) ) ;
#6723=CARTESIAN_POINT ( 'NONE',  ( -0.1574803149606299191, -0.1751968502861738219, 0.000000000000000000 ) ) ;
#6728=CARTESIAN_POINT ( 'NONE',  ( -0.1344904043211537503, -0.09851384275058189255, -0.1217015355611421323 ) ) ;
#6739=CARTESIAN_POINT ( 'NONE',  ( 0.1787899950787401882, -0.8469488188438739629, -2.189545951927503898E-17 ) ) ;
#6744=CARTESIAN_POINT ( 'NONE',  ( -0.1787899950787401882, -0.09510428318986871576, 0.000000000000000000 ) ) ;
#6745=CARTESIAN_POINT ( 'NONE',  ( -0.1264236179284866091, -0.2810039369541106336, -0.1264236179284866091 ) ) ;
#6753=CARTESIAN_POINT ( 'NONE',  ( -0.1797182628040039087, -1.809591053677533479, 0.07444174185955065859 ) ) ;
#6762=CARTESIAN_POINT ( 'NONE',  ( -0.1910692666444312182, -0.07766248740295460251, -0.1751191768260007275 ) ) ;
#6766=CARTESIAN_POINT ( 'NONE',  ( -0.06523048226347956391, -0.9158464565853854378, 0.1574803149606297803 ) ) ;
#6767=CARTESIAN_POINT ( 'NONE',  ( -0.07405724077823318263, -0.1309055117572600901, -0.1787899950787401604 ) ) ;
#6769=CARTESIAN_POINT ( 'NONE',  ( -1.094772975963752103E-17, -1.152066929080094448, -0.1787899950787401882 ) ) ;
#6786=CARTESIAN_POINT ( 'NONE',  ( 0.07405724077823318263, -0.03248031490686641154, 0.1787899950787401604 ) ) ;
#6793=CARTESIAN_POINT ( 'NONE',  ( -0.07405724077823318263, -1.308194834370970616, 0.1787899950787401604 ) ) ;
#6795=CARTESIAN_POINT ( 'NONE',  ( 3.284318927891251994E-17, -0.2268700786863941110, 0.1787899950787401882 ) ) ;
#6800=CARTESIAN_POINT ( 'NONE',  ( -0.2471911387362889789, -0.08795568039072379496, 0.05508755932689571311 ) ) ;
#6802=CARTESIAN_POINT ( 'NONE',  ( 0.07405724077823318263, -1.607283464513165949, 0.1787899950787401604 ) ) ;
#6812=CARTESIAN_POINT ( 'NONE',  ( 0.03906282586613502722, 0.1299212598425196485, 0.1731955441111237004 ) ) ;
#6814=LINE ( 'NONE', #35139, #47359 ) ;
#6830=CARTESIAN_POINT ( 'NONE',  ( 0.07405724077823318263, 0.02657480320336980464, -0.1787899950787401604 ) ) ;
#6834=CARTESIAN_POINT ( 'NONE',  ( 0.1924606493446845146, 0.07681961335490640475, 0.1743158631585779439 ) ) ;
#6838=ORIENTED_EDGE ( 'NONE', *, *, #38581, .T. ) ;
#6839=CARTESIAN_POINT ( 'NONE',  ( -0.06523048226347956391, 0.09301181113114917465, -0.1574803149606300301 ) ) ;
#6849=CARTESIAN_POINT ( 'NONE',  ( 0.1787899950787401604, -0.8652814485442000825, 0.07405724077823318263 ) ) ;
#6851=CARTESIAN_POINT ( 'NONE',  ( 0.07971570266418918915, -0.08956247127877224601, 0.1225084993081602541 ) ) ;
#6853=CARTESIAN_POINT ( 'NONE',  ( -0.07405724077823318263, 0.1250000000537635492, 0.1787899950787401604 ) ) ;
#6862=EDGE_CURVE ( 'NONE', #5618, #47458, #45474, .T. ) ;
#6866=CARTESIAN_POINT ( 'NONE',  ( 0.1797182628040039087, -0.8105753056460376360, 0.07444174185955046430 ) ) ;
#6870=CARTESIAN_POINT ( 'NONE',  ( 2.892866454678787531E-17, -0.6476377952755905110, 0.1574803149606299191 ) ) ;
#6871=CARTESIAN_POINT ( 'NONE',  ( -0.1272003972225189405, 0.1291484615524529089, 0.1088019360944664504 ) ) ;
#6881=DIRECTION ( 'NONE',  ( 0.000000000000000000, 0.000000000000000000, -1.000000000000000000 ) ) ;
#6883=DIRECTION ( 'NONE',  ( 0.000000000000000000, 1.000000000000000000, 0.000000000000000000 ) ) ;
#6889=CARTESIAN_POINT ( 'NONE',  ( -0.1270800023317771588, 0.08263335577128524956, 0.1270800023317771588 ) ) ;
#6890=CARTESIAN_POINT ( 'NONE',  ( 0.1264236179284866091, -1.280019684985606254, -0.1264236179284866091 ) ) ;
#6891=CARTESIAN_POINT ( 'NONE',  ( -0.06523048226347956391, -1.570374015748031704, -0.1574803149606300301 ) ) ;
#6897=CARTESIAN_POINT ( 'NONE',  ( -0.06523048226347956391, -1.403051180994835390, -0.1574803149606300301 ) ) ;
#6902=CARTESIAN_POINT ( 'NONE',  ( -0.1607584476970242982, 0.09202339627320738069, -0.1926191378137585286 ) ) ;
#6907=CARTESIAN_POINT ( 'NONE',  ( 0.1787899950787401604, -0.4666594013001046926, -0.07405724077823318263 ) ) ;
#6908=CARTESIAN_POINT ( 'NONE',  ( -0.1537350773408287519, -0.09842519685039370636, 0.06905093064059350527 ) ) ;
#6918=CARTESIAN_POINT ( 'NONE',  ( 0.07405724077823318263, -1.174212598371433769, 0.1787899950787401604 ) ) ;
#6919=CARTESIAN_POINT ( 'NONE',  ( -0.1787899950787401604, -1.341535433017102541, -0.07405724077823318263 ) ) ;
#6921=CARTESIAN_POINT ( 'NONE',  ( 0.000000000000000000, 0.1102362204724409434, 0.2007874015748031815 ) ) ;
#6923=CARTESIAN_POINT ( 'NONE',  ( -0.1797182628040039087, -0.5891186127326517585, 0.07444174185955065859 ) ) ;
#6928=CARTESIAN_POINT ( 'NONE',  ( 0.1113553986120547346, -0.1998031496062991907, -0.1113553986120547346 ) ) ;
#6941=CARTESIAN_POINT ( 'NONE',  ( -0.1787899950787401604, -0.07677165348954355373, 0.07405724077823318263 ) ) ;
#6943=CARTESIAN_POINT ( 'NONE',  ( 0.1574803149606299191, -1.533464566821606034, -1.928577636452523993E-17 ) ) ;
#6944=CARTESIAN_POINT ( 'NONE',  ( -0.1264236179284866091, -0.7583661416785196785, -0.1264236179284866091 ) ) ;
#6947=CARTESIAN_POINT ( 'NONE',  ( 0.1574803149606300301, -0.9896653543307096790, -0.06523048226347956391 ) ) ;
#6965=CARTESIAN_POINT ( 'NONE',  ( 0.06523048226347956391, -0.1481299211523154913, -0.1574803149606300301 ) ) ;
#6971=CARTESIAN_POINT ( 'NONE',  ( -0.1717461275140602373, -0.09851383607918347274, -0.03673640942690917233 ) ) ;
#6976=CARTESIAN_POINT ( 'NONE',  ( -0.1787899950787401604, -1.751108220197743259, -0.07405724077823318263 ) ) ;
#6979=EDGE_LOOP ( 'NONE', ( #9941, #42278 ) ) ;
#6983=CARTESIAN_POINT ( 'NONE',  ( -1.094772975963752103E-17, -0.8764763778989921317, -0.1787899950787401882 ) ) ;
#6984=CARTESIAN_POINT ( 'NONE',  ( -0.2471921406146342093, -0.06698952652845348299, -0.09859233283838723938 ) ) ;
#6987=CARTESIAN_POINT ( 'NONE',  ( 0.1797182628040039087, -0.2151028647011559158, -0.07444174185955065859 ) ) ;
#6988=CARTESIAN_POINT ( 'NONE',  ( 0.1264236179284866091, -0.1886082201977429262, -0.1264236179284866091 ) ) ;
#6989=CARTESIAN_POINT ( 'NONE',  ( 0.07405724077823318263, -0.07185039364702387743, 0.1787899950787401604 ) ) ;
#6994=CARTESIAN_POINT ( 'NONE',  ( 0.1270800023317771588, -1.708705226905880004, -0.1270800023317771588 ) ) ;
#7000=ORIENTED_EDGE ( 'NONE', *, *, #16935, .T. ) ;
#7002=CARTESIAN_POINT ( 'NONE',  ( -9.642888182262618425E-18, -0.8937007872940473385, -0.1574803149606299191 ) ) ;
#7003=CARTESIAN_POINT ( 'NONE',  ( -0.07405724077823318263, -0.1702755904974175283, -0.1787899950787401604 ) ) ;
#7006=CARTESIAN_POINT ( 'NONE',  ( 0.07405724077823318263, -1.075787401521038689, -0.1787899950787401604 ) ) ;
#7015=CARTESIAN_POINT ( 'NONE',  ( -0.1574803149606297803, -1.117618110128692832, 0.06523048226347956391 ) ) ;
#7019=DIRECTION ( 'NONE',  ( 0.000000000000000000, 1.000000000000000000, 0.000000000000000000 ) ) ;
#7029=CARTESIAN_POINT ( 'NONE',  ( -0.07405724077823318263, 0.04133858273092887170, 0.1787899950787401604 ) ) ;
#7038=CARTESIAN_POINT ( 'NONE',  ( -1.094772975963752103E-17, -1.325419243819789594, -0.1787899950787401882 ) ) ;
#7040=CARTESIAN_POINT ( 'NONE',  ( -0.07405724077823318263, -0.3228346456155278266, -0.1787899950787401604 ) ) ;
#7050=CARTESIAN_POINT ( 'NONE',  ( -0.1264236179284866091, -1.614665354276944909, 0.1264236179284866091 ) ) ;
#7051=CARTESIAN_POINT ( 'NONE',  ( 0.1787899950787401882, -0.7731299212060788184, -2.189545951927503898E-17 ) ) ;
#7053=CARTESIAN_POINT ( 'NONE',  ( 0.07444174185955046430, -1.312543809583045284, -0.1797182628040039087 ) ) ;
#7060=CARTESIAN_POINT ( 'NONE',  ( -9.642888182262618425E-18, -0.7755905510735748853, -0.1574803149606299191 ) ) ;
#7078=CARTESIAN_POINT ( 'NONE',  ( -0.1264236179284866091, -0.04478346451316559534, -0.1264236179284866091 ) ) ;
#7089=CARTESIAN_POINT ( 'NONE',  ( -0.1787899950787401604, -1.779527559001355952, -0.07405724077823318263 ) ) ;
#7097=CARTESIAN_POINT ( 'NONE',  ( -0.07405724077823318263, -0.8505176690166401654, -0.1787899950787401604 ) ) ;
#7098=ORIENTED_EDGE ( 'NONE', *, *, #30598, .F. ) ;
#7099=CARTESIAN_POINT ( 'NONE',  ( 0.0001126629808640675258, -0.08956164707051811336, 0.1524538216589708950 ) ) ;
#7100=CARTESIAN_POINT ( 'NONE',  ( -0.07405724077823318263, 0.1496062992663619862, -0.1787899950787401604 ) ) ;
#7112=VERTEX_POINT ( 'NONE', #20482 ) ;
#7114=CARTESIAN_POINT ( 'NONE',  ( -0.1797182628040039087, -0.8302603450161165632, -0.07444174185955065859 ) ) ;
#7118=CARTESIAN_POINT ( 'NONE',  ( 2.892866454678787531E-17, -0.5688976377952755792, 0.1574803149606299191 ) ) ;
#7121=CARTESIAN_POINT ( 'NONE',  ( -0.1613734868294114388, 0.1271050926819339011, 0.03304375603688991525 ) ) ;
#7138=CARTESIAN_POINT ( 'NONE',  ( -0.07405724077823318263, -1.218503936954111300, 0.1787899950787401604 ) ) ;
#7139=CARTESIAN_POINT ( 'NONE',  ( -0.1113553986120547346, -1.449803149606299080, -0.1113553986120547346 ) ) ;
#7150=CARTESIAN_POINT ( 'NONE',  ( -0.1924606493446819333, 0.07681961335490891662, -0.1743158631585794982 ) ) ;
#7152=CARTESIAN_POINT ( 'NONE',  ( 0.08837038158042308245, -0.09266989036297280935, -0.2344124146308698975 ) ) ;
#7155=CARTESIAN_POINT ( 'NONE',  ( 0.1264236179284866091, -0.3559310548434121979, 0.1264236179284866091 ) ) ;
#7156=CARTESIAN_POINT ( 'NONE',  ( 0.04596748140029709162, -0.09842519685039370636, 0.1460059822399198959 ) ) ;
#7166=CARTESIAN_POINT ( 'NONE',  ( -0.07405724077823318263, -1.154527559001354842, -0.1787899950787401604 ) ) ;
#7167=CARTESIAN_POINT ( 'NONE',  ( 0.1787899950787401882, -1.398129921206078707, -2.189545951927503898E-17 ) ) ;
#7171=CARTESIAN_POINT ( 'NONE',  ( -0.1797182628040039087, -0.6284886914728088358, 0.07444174185955065859 ) ) ;
#7174=CARTESIAN_POINT ( 'NONE',  ( 0.1574803149606299191, -0.2047244094488188948, -1.928577636452523993E-17 ) ) ;
#7188=CARTESIAN_POINT ( 'NONE',  ( -0.1574803149606299191, -1.474409448711370141, 0.000000000000000000 ) ) ;
#7189=CARTESIAN_POINT ( 'NONE',  ( -0.07405724077823318263, -0.6820866141194646959, -0.1787899950787401604 ) ) ;
#7191=CARTESIAN_POINT ( 'NONE',  ( -0.06523048226347956391, -1.043799212598425452, 0.1574803149606297803 ) ) ;
#7208=ADVANCED_FACE ( 'NONE', ( #19775 ), #5633, .T. ) ;
#7210=CARTESIAN_POINT ( 'NONE',  ( 0.1574803149606300301, -0.1579724408373548161, 0.06523048226347956391 ) ) ;
#7215=CARTESIAN_POINT ( 'NONE',  ( -0.1561580984082978352, -0.09851383248064074505, 0.06438758770809645260 ) ) ;
#7220=CARTESIAN_POINT ( 'NONE',  ( -0.1787899950787401604, -1.706816881615065951, 0.07405724077823318263 ) ) ;
#7225=CARTESIAN_POINT ( 'NONE',  ( 0.1787899950787401604, -0.9625984251430860228, -0.07405724077823318263 ) ) ;
#7226=CARTESIAN_POINT ( 'NONE',  ( -0.2471922904502822094, -0.05170400041268939650, -0.1201839652816935194 ) ) ;
#7232=CARTESIAN_POINT ( 'NONE',  ( -0.1270800023317771588, -0.1634296363546990094, -0.1270800023317771588 ) ) ;
#7233=CARTESIAN_POINT ( 'NONE',  ( 0.1787899950787401604, -0.1123286926386875273, -0.07405724077823318263 ) ) ;
#7234=CARTESIAN_POINT ( 'NONE',  ( 0.1264236179284866091, -0.06938976372576398377, 0.1264236179284866091 ) ) ;
#7235=FACE_OUTER_BOUND ( 'NONE', #2150, .T. ) ;
#7240=CARTESIAN_POINT ( 'NONE',  ( -0.1787899950787401604, -0.4360236219934807145, -0.07405724077823318263 ) ) ;
#7250=CARTESIAN_POINT ( 'NONE',  ( 0.1264236179284866091, -0.3351377952218271283, -0.1264236179284866091 ) ) ;
#7253=CARTESIAN_POINT ( 'NONE',  ( 0.1264236179284866091, -1.117618110182456714, -0.1264236179284866091 ) ) ;
#7275=CARTESIAN_POINT ( 'NONE',  ( 0.1264236179284866091, -0.05954724404072461036, -0.1264236179284866091 ) ) ;
#7282=CARTESIAN_POINT ( 'NONE',  ( 0.1787899950787401604, -1.332801133583568776, -0.07405724077823318263 ) ) ;
#7284=CARTESIAN_POINT ( 'NONE',  ( -0.1264236179284866091, -0.3499015747493862127, 0.1264236179284866091 ) ) ;
#7291=CARTESIAN_POINT ( 'NONE',  ( -1.094772975963752103E-17, -1.668799212544661348, -0.1787899950787401882 ) ) ;
#7292=CARTESIAN_POINT ( 'NONE',  ( -1.094772975963752103E-17, -1.742618110182456714, -0.1787899950787401882 ) ) ;
#7295=CARTESIAN_POINT ( 'NONE',  ( 0.1797182628040039087, -1.322386329268085525, 0.07444174185955046430 ) ) ;
#7325=CARTESIAN_POINT ( 'NONE',  ( -1.094772975963752103E-17, -0.1284448818360001965, -0.1787899950787401882 ) ) ;
#7333=CARTESIAN_POINT ( 'NONE',  ( -0.1574803149606300301, 0.05856299223351124628, -0.06523048226347956391 ) ) ;
#7344=CARTESIAN_POINT ( 'NONE',  ( 3.284318927891251994E-17, -0.7939231808276635549, 0.1787899950787401882 ) ) ;
#7357=CARTESIAN_POINT ( 'NONE',  ( -0.1270800023317771588, -0.8720910536775334787, -0.1270800023317771588 ) ) ;
#7373=CARTESIAN_POINT ( 'NONE',  ( 3.284318927891251994E-17, -0.8174212597887557941, 0.1787899950787401882 ) ) ;
#7381=CARTESIAN_POINT ( 'NONE',  ( 2.892866454678787531E-17, -1.553149606299212504, 0.1574803149606299191 ) ) ;
#7387=CARTESIAN_POINT ( 'NONE',  ( -0.1113553986120547346, -0.2982283463491657294, -0.1113553986120547346 ) ) ;
#7394=CARTESIAN_POINT ( 'NONE',  ( -0.07405724077823318263, -0.3633129446071917679, 0.1787899950787401604 ) ) ;
#7395=CARTESIAN_POINT ( 'NONE',  ( -0.004819917375885433841, -0.09842519685039370636, 0.1563213176426297146 ) ) ;
#7401=CARTESIAN_POINT ( 'NONE',  ( 0.07405724077823318263, -1.159448818843874074, -0.1787899950787401604 ) ) ;
#7402=CARTESIAN_POINT ( 'NONE',  ( -0.1264236179284866091, -1.334153543253322916, 0.1264236179284866091 ) ) ;
#7406=CARTESIAN_POINT ( 'NONE',  ( -0.06523048226347956391, -0.1924212598425195098, -0.1574803149606300301 ) ) ;
#7419=CARTESIAN_POINT ( 'NONE',  ( 0.1787899950787401604, -1.513779527505292322, -0.07405724077823318263 ) ) ;
#7420=CARTESIAN_POINT ( 'NONE',  ( 0.06523048226347956391, -1.580216535325544402, 0.1574803149606297803 ) ) ;
#7421=CARTESIAN_POINT ( 'NONE',  ( 0.1787899950787401882, -0.7337598424659212970, -2.189545951927503898E-17 ) ) ;
#7423=CARTESIAN_POINT ( 'NONE',  ( 0.1574803149606300301, -1.068405511811023612, -0.06523048226347956391 ) ) ;
#7450=CARTESIAN_POINT ( 'NONE',  ( 0.1787899950787401882, -0.4187992125446614589, -2.189545951927503898E-17 ) ) ;
#7451=CARTESIAN_POINT ( 'NONE',  ( 0.1264236179284866091, -0.8518700786863936392, 0.1264236179284866091 ) ) ;
#7453=CARTESIAN_POINT ( 'NONE',  ( -0.2471920549080087737, -0.08080427097412125337, -0.07167403547431477895 ) ) ;
#7457=CARTESIAN_POINT ( 'NONE',  ( -0.1797182628040039365, -0.2372485339924944592, 0.000000000000000000 ) ) ;
#7458=CARTESIAN_POINT ( 'NONE',  ( 0.07405724077823318263, -0.1221712123237270187, 0.1787899950787401604 ) ) ;
#7464=FILL_AREA_STYLE ('',( #33376 ) ) ;
#7468=CARTESIAN_POINT ( 'NONE',  ( -0.2088134963331629290, -0.06712557525897992761, 0.1648743713630835273 ) ) ;
#7469=EDGE_CURVE ( 'NONE', #36271, #4939, #44619, .T. ) ;
#7471=CARTESIAN_POINT ( 'NONE',  ( 3.284318927891251994E-17, -0.3499015747493862127, 0.1787899950787401882 ) ) ;
#7474=CARTESIAN_POINT ( 'NONE',  ( -0.1787899950787401604, -1.065944881836000224, -0.07405724077823318263 ) ) ;
#7481=CARTESIAN_POINT ( 'NONE',  ( -0.1574803149606297803, -1.196358267609008763, 0.06523048226347956391 ) ) ;
#7493=CARTESIAN_POINT ( 'NONE',  ( -0.1787899950787401882, -0.04478346451316559534, 0.000000000000000000 ) ) ;
#7502=CARTESIAN_POINT ( 'NONE',  ( -0.1264236179284866091, -1.350025543032387976, 0.1264236179284866091 ) ) ;
#7504=CARTESIAN_POINT ( 'NONE',  ( -0.07405724077823318263, -0.2293307086076536994, 0.1787899950787401604 ) ) ;
#7505=CARTESIAN_POINT ( 'NONE',  ( -0.1574803149606300301, 0.01919291349335381161, -0.06523048226347956391 ) ) ;
#7512=CARTESIAN_POINT ( 'NONE',  ( -0.1787899950787401882, -1.619586614119464585, 0.000000000000000000 ) ) ;
#7513=CARTESIAN_POINT ( 'NONE',  ( -0.1787899950787401604, -1.735236220418678643, -0.07405724077823318263 ) ) ;
#7517=CARTESIAN_POINT ( 'NONE',  ( -0.1270800023317771588, -1.492169793835013802, 0.1270800023317771588 ) ) ;
#7524=CARTESIAN_POINT ( 'NONE',  ( 0.05391291923841142614, 0.1299212598425196763, 0.1701573640430796008 ) ) ;
#7527=CARTESIAN_POINT ( 'NONE',  ( -0.1113553986120547346, -0.8100393699712126194, -0.1113553986120547346 ) ) ;
#7539=ORIENTED_EDGE ( 'NONE', *, *, #32770, .T. ) ;
#7548=CARTESIAN_POINT ( 'NONE',  ( -0.07405724077823318263, -0.1259842519147404416, -0.1787899950787401604 ) ) ;
#7552=CARTESIAN_POINT ( 'NONE',  ( -0.1235961452251413406, -0.09842519685039370636, 0.2140748031496062798 ) ) ;
#7555=CARTESIAN_POINT ( 'NONE',  ( -0.1787899950787401882, -1.816437007820251859, 0.000000000000000000 ) ) ;
#7563=CARTESIAN_POINT ( 'NONE',  ( 3.284318927891251994E-17, -0.8332932595678209653, 0.1787899950787401882 ) ) ;
#7564=ORIENTED_EDGE ( 'NONE', *, *, #19593, .T. ) ;
#7575=ADVANCED_FACE ( 'NONE', ( #15673 ), #33191, .F. ) ;
#7579=CARTESIAN_POINT ( 'NONE',  ( -0.1797182628040039087, -0.9483705812365885723, -0.07444174185955065859 ) ) ;
#7588=CARTESIAN_POINT ( 'NONE',  ( -0.06523048226347956391, -0.6550196849318432601, -0.1574803149606300301 ) ) ;
#7592=CARTESIAN_POINT ( 'NONE',  ( 0.1264236179284866091, -0.7731299212060788184, 0.1264236179284866091 ) ) ;
#7597=CARTESIAN_POINT ( 'NONE',  ( -0.1574803149606300301, -1.722933070866142335, -0.06523048226347956391 ) ) ;
#7599=ORIENTED_EDGE ( 'NONE', *, *, #37764, .T. ) ;
#7604=CARTESIAN_POINT ( 'NONE',  ( 0.07405724077823318263, -1.449803149552535642, 0.1787899950787401604 ) ) ;
#7611=CARTESIAN_POINT ( 'NONE',  ( 0.07034821948466062069, 0.08559642391438646025, -0.2448175074096619885 ) ) ;
#7613=CARTESIAN_POINT ( 'NONE',  ( -0.2329120156667235930, -0.08955973368226792519, -0.06010530154842106537 ) ) ;
#7619=AXIS2_PLACEMENT_3D ( 'NONE', #26889, #41446, #8648 ) ;
#7626=CARTESIAN_POINT ( 'NONE',  ( 0.1787899950787401882, -1.324311023568283341, -2.189545951927503898E-17 ) ) ;
#7628=CARTESIAN_POINT ( 'NONE',  ( 0.1264236179284866091, -1.432578740103716664, -0.1264236179284866091 ) ) ;
#7635=CARTESIAN_POINT ( 'NONE',  ( -0.1574803149606299191, -0.2244094488188976555, 0.000000000000000000 ) ) ;
#7639=CARTESIAN_POINT ( 'NONE',  ( -0.1355716054994425268, -0.09355356640806745949, -0.1165615083013312042 ) ) ;
#7642=CARTESIAN_POINT ( 'NONE',  ( 0.1113553986120547346, -0.5049212597349921339, -0.1113553986120547346 ) ) ;
#7644=CARTESIAN_POINT ( 'NONE',  ( -0.1850388559550336376, -0.08126078924477943277, -0.1786007880584631891 ) ) ;
#7647=CARTESIAN_POINT ( 'NONE',  ( 0.1787899950787401604, -1.553149606245448178, -0.07405724077823318263 ) ) ;
#7648=CARTESIAN_POINT ( 'NONE',  ( 0.1113553986120547346, -1.538385826664125711, 0.1113553986120547346 ) ) ;
#7649=CARTESIAN_POINT ( 'NONE',  ( 0.1787899950787401604, -0.8100393700249772788, -0.07405724077823318263 ) ) ;
#7650=CARTESIAN_POINT ( 'NONE',  ( 0.1113553986120547346, -1.233267716535433101, 0.1113553986120547346 ) ) ;
#7652=( BOUNDED_CURVE ( )  B_SPLINE_CURVE ( 2, ( #925, #38311, #41400, #26840, #15823, #37353, #15583, #1396, #19142 ),
 .UNSPECIFIED., .F., .T. ) 
 B_SPLINE_CURVE_WITH_KNOTS ( ( 3, 2, 2, 2, 3 ),
 ( 0.09500000000000000111, 0.09750000000000000333, 0.1000000000000000056, 0.1024999999999999939, 0.1049999999999999961 ),
 .UNSPECIFIED. ) 
 CURVE ( )  GEOMETRIC_REPRESENTATION_ITEM ( )  RATIONAL_B_SPLINE_CURVE ( ( 1.000000000000000000, 0.9238795325112869605, 1.000000000000000000, 0.9238795325112869605, 1.000000000000000000, 0.9238795325112869605, 1.000000000000000000, 0.9238795325112869605, 1.000000000000000000 ) ) 
 REPRESENTATION_ITEM ( '' )  ) ;
#7676=CARTESIAN_POINT ( 'NONE',  ( 0.05548443445031432664, -0.09851382384500374789, 0.1418811546954053260 ) ) ;
#7679=EDGE_CURVE ( 'NONE', #3517, #33652, #31228, .T. ) ;
#7683=CARTESIAN_POINT ( 'NONE',  ( 0.07405724077823318263, -0.9625984251430860228, -0.1787899950787401604 ) ) ;
#7684=CARTESIAN_POINT ( 'NONE',  ( 0.1264236179284866091, -0.4532480314422991929, -0.1264236179284866091 ) ) ;
#7685=CARTESIAN_POINT ( 'NONE',  ( 0.1787899950787401604, -0.9675196849856075865, 0.07405724077823318263 ) ) ;
#7686=ORIENTED_EDGE ( 'NONE', *, *, #39158, .F. ) ;
#7691=CARTESIAN_POINT ( 'NONE',  ( 0.07444174185955065859, -0.1855753056460376360, 0.1797182628040039087 ) ) ;
#7695=CARTESIAN_POINT ( 'NONE',  ( -0.1787899950787401604, -0.1259842519147404416, -0.07405724077823318263 ) ) ;
#7696=CARTESIAN_POINT ( 'NONE',  ( 0.2471914725378836220, -0.08966515697934822338, -0.05042473337714371839 ) ) ;
#7707=CARTESIAN_POINT ( 'NONE',  ( -0.1787899950787401882, -0.2416338582139531399, 0.000000000000000000 ) ) ;
#7710=CARTESIAN_POINT ( 'NONE',  ( 3.284318927891251994E-17, -1.132381889710015743, 0.1787899950787401882 ) ) ;
#7738=CARTESIAN_POINT ( 'NONE',  ( 0.1264236179284866091, -1.448450739882781502, -0.1264236179284866091 ) ) ;
#7742=CARTESIAN_POINT ( 'NONE',  ( 0.07405724077823318263, -0.3425196849856064762, 0.1787899950787401604 ) ) ;
#7750=CARTESIAN_POINT ( 'NONE',  ( 0.1787899950787401604, -1.676181102308441639, -0.07405724077823318263 ) ) ;
#7751=CARTESIAN_POINT ( 'NONE',  ( -1.094772975963752103E-17, -1.703248031442299304, -0.1787899950787401882 ) ) ;
#7752=SHAPE_DEFINITION_REPRESENTATION ( #12849, #45408 ) ;
#7755=CARTESIAN_POINT ( 'NONE',  ( -0.1270800023317771588, -1.383902077299580702, -0.1270800023317771588 ) ) ;
#7764=CYLINDRICAL_SURFACE ( 'NONE', #24401, 0.1574803149606299191 ) ;
#7766=DIRECTION ( 'NONE',  ( 0.000000000000000000, 1.000000000000000000, 0.000000000000000000 ) ) ;
#7777=CARTESIAN_POINT ( 'NONE',  ( -0.1797182628040039365, -0.04039814029170692850, 0.000000000000000000 ) ) ;
#7778=CARTESIAN_POINT ( 'NONE',  ( -0.1574803149606300301, -1.043799212490898132, -0.06523048226347956391 ) ) ;
#7785=CARTESIAN_POINT ( 'NONE',  ( -0.1787899950787401604, -0.1948818897100161873, 0.07405724077823318263 ) ) ;
#7788=CARTESIAN_POINT ( 'NONE',  ( -0.01929052294527481767, -0.05062618494071657177, 0.2742915362215331831 ) ) ;
#7792=CARTESIAN_POINT ( 'NONE',  ( -1.094772975963752103E-17, -1.786909448765134023, -0.1787899950787401882 ) ) ;
#7801=CARTESIAN_POINT ( 'NONE',  ( 0.000000000000000000, 0.0004086818895575684884, 0.000000000000000000 ) ) ;
#7802=CARTESIAN_POINT ( 'NONE',  ( 0.1264236179284866091, -1.054749952481206732, -0.1264236179284866091 ) ) ;
#7804=CARTESIAN_POINT ( 'NONE',  ( 0.1787899950787401604, 0.1397637795813224670, -0.07405724077823318263 ) ) ;
#7811=CARTESIAN_POINT ( 'NONE',  ( -1.094772975963752103E-17, -0.5270669290800944484, -0.1787899950787401882 ) ) ;
#7815=CARTESIAN_POINT ( 'NONE',  ( -0.07444174185955065859, -1.056638297772022339, 0.1797182628040039087 ) ) ;
#7829=CARTESIAN_POINT ( 'NONE',  ( 0.07405724077823318263, -0.8001968503399367050, -0.1787899950787401604 ) ) ;
#7837=CARTESIAN_POINT ( 'NONE',  ( 1.928577636452524610E-17, -0.09842519685039370636, -0.1574803149606299191 ) ) ;
#7838=CARTESIAN_POINT ( 'NONE',  ( 0.1574803149606299191, -1.740157480314960869, -1.928577636452523993E-17 ) ) ;
#7853=CARTESIAN_POINT ( 'NONE',  ( -0.07405724077823318263, -0.4174468028749078186, -0.1787899950787401604 ) ) ;
#7854=CARTESIAN_POINT ( 'NONE',  ( -0.08928429026229449395, -0.08955962610386575262, -0.2342853990049039437 ) ) ;
#7856=CARTESIAN_POINT ( 'NONE',  ( 0.000000000000000000, -0.09842519685039370636, 0.000000000000000000 ) ) ;
#7865=CARTESIAN_POINT ( 'NONE',  ( 0.07405724077823318263, -1.356299212544662014, -0.1787899950787401604 ) ) ;
#7866=CARTESIAN_POINT ( 'NONE',  ( -0.1264236179284866091, -1.501476377898992354, -0.1264236179284866091 ) ) ;
#7875=CARTESIAN_POINT ( 'NONE',  ( 2.892866454678787531E-17, -0.2933070866141732624, 0.1574803149606299191 ) ) ;
#7890=CARTESIAN_POINT ( 'NONE',  ( -0.1787899950787401604, -1.494094488135213394, 0.07405724077823318263 ) ) ;
#7891=CARTESIAN_POINT ( 'NONE',  ( 0.1264236179284866091, -0.6894685038832439883, -0.1264236179284866091 ) ) ;
#7892=CARTESIAN_POINT ( 'NONE',  ( 0.1574803149606300301, -1.270177165354331006, 0.06523048226347956391 ) ) ;
#7918=CARTESIAN_POINT ( 'NONE',  ( -0.2395411720923122101, -0.09842519685039370636, 0.02158160309225409801 ) ) ;
#7924=CARTESIAN_POINT ( 'NONE',  ( -0.1264236179284866091, -0.8764763778989921317, -0.1264236179284866091 ) ) ;
#7925=CARTESIAN_POINT ( 'NONE',  ( 0.1787899950787401882, -0.4581692912848189247, -2.189545951927503898E-17 ) ) ;
#7926=CARTESIAN_POINT ( 'NONE',  ( -0.1264236179284866091, -1.029035433017102319, -0.1264236179284866091 ) ) ;
#7929=CARTESIAN_POINT ( 'NONE',  ( 0.1270800023317771588, -0.3405949906854078280, 0.1270800023317771588 ) ) ;
#7931=CARTESIAN_POINT ( 'NONE',  ( -0.06523048226347956391, 0.1373031496062993018, 0.1574803149606297803 ) ) ;
#7932=CARTESIAN_POINT ( 'NONE',  ( 0.1787899950787401882, -0.06446850388324429360, -2.189545951927503898E-17 ) ) ;
#7934=B_SPLINE_CURVE_WITH_KNOTS ( 'NONE', 3,
 ( #26979, #30579, #13068, #42267 ),
 .UNSPECIFIED., .F., .F.,
 ( 4, 4 ),
 ( 0.000000000000000000, 0.0002204554312150490089 ),
 .UNSPECIFIED. ) ;
#7947=CARTESIAN_POINT ( 'NONE',  ( -0.1787899950787401604, -0.2440944881352131168, -0.07405724077823318263 ) ) ;
#7949=CARTESIAN_POINT ( 'NONE',  ( -0.1787899950787401604, -1.184055118056472455, -0.07405724077823318263 ) ) ;
#7959=EDGE_CURVE ( 'NONE', #22067, #45034, #10053, .T. ) ;
#7960=CARTESIAN_POINT ( 'NONE',  ( -0.07382755323629552890, -0.09842514923570476471, -0.1628384097759718319 ) ) ;
#7972=ORIENTED_EDGE ( 'NONE', *, *, #14716, .T. ) ;
#7974=CARTESIAN_POINT ( 'NONE',  ( 0.1264236179284866091, -1.487820818622939134, -0.1264236179284866091 ) ) ;
#7977=CARTESIAN_POINT ( 'NONE',  ( -0.1264236179284866091, -0.5073818897100158543, 0.1264236179284866091 ) ) ;
#7978=CARTESIAN_POINT ( 'NONE',  ( -0.06523048226347956391, 0.02903543317839319890, 0.1574803149606297803 ) ) ;
#7985=CARTESIAN_POINT ( 'NONE',  ( 0.1264236179284866091, -1.752460629867496067, -0.1264236179284866091 ) ) ;
#7986=CARTESIAN_POINT ( 'NONE',  ( -0.1787899950787401604, -1.695866141678520567, -0.07405724077823318263 ) ) ;
#7991=CARTESIAN_POINT ( 'NONE',  ( 0.06523048226347956391, -0.7878937007874025067, -0.1574803149606300301 ) ) ;
#7992=CARTESIAN_POINT ( 'NONE',  ( 0.1797182628040039365, -1.438035935567297141, -2.200913952912460540E-17 ) ) ;
#7995=CARTESIAN_POINT ( 'NONE',  ( 0.2471922904502826257, 0.09660984127287175482, -0.02629157619858345576 ) ) ;
#8012=CARTESIAN_POINT ( 'NONE',  ( 0.1797182628040039087, -0.06254380958304553428, 0.07444174185955046430 ) ) ;
#8013=CARTESIAN_POINT ( 'NONE',  ( -0.07405724077823318263, -1.233267716481668774, -0.1787899950787401604 ) ) ;
#8020=CARTESIAN_POINT ( 'NONE',  ( 0.1264236179284866091, -0.1333661416785200671, -0.1264236179284866091 ) ) ;
#8027=CARTESIAN_POINT ( 'NONE',  ( -0.1574803149606299191, -0.05708661406570126468, 0.000000000000000000 ) ) ;
#8031=AXIS2_PLACEMENT_3D ( 'NONE', #44265, #15073, #47415 ) ;
#8034=CARTESIAN_POINT ( 'NONE',  ( -0.1264236179284866091, -1.005537354056009969, -0.1264236179284866091 ) ) ;
#8036=CARTESIAN_POINT ( 'NONE',  ( 0.07405724077823318263, 0.05118110241596821736, 0.1787899950787401604 ) ) ;
#8042=CARTESIAN_POINT ( 'NONE',  ( 0.1787899950787401604, -0.5344488188438744070, -0.07405724077823318263 ) ) ;
#8048=CARTESIAN_POINT ( 'NONE',  ( -0.1270800023317771588, -0.9508312111578485215, -0.1270800023317771588 ) ) ;
#8062=CARTESIAN_POINT ( 'NONE',  ( 0.1264236179284866091, -0.6943897637257637756, 0.1264236179284866091 ) ) ;
#8067=AXIS2_PLACEMENT_3D ( 'NONE', #1133, #44266, #44735 ) ;
#8072=CARTESIAN_POINT ( 'NONE',  ( 0.06523048226347956391, -1.629429133858268930, 0.1574803149606297803 ) ) ;
#8079=CARTESIAN_POINT ( 'NONE',  ( 0.07405724077823318263, -1.592519684985606254, -0.1787899950787401604 ) ) ;
#8085=CARTESIAN_POINT ( 'NONE',  ( 0.1345513924870780087, 0.1295369909362752148, -0.09891213622343476841 ) ) ;
#8086=CARTESIAN_POINT ( 'NONE',  ( 0.02442443439252881682, 0.05525422739384140691, -0.2713316170948109063 ) ) ;
#8088=CARTESIAN_POINT ( 'NONE',  ( -0.07405724077823318263, -0.6142971965756950370, -0.1787899950787401604 ) ) ;
#8089=CARTESIAN_POINT ( 'NONE',  ( -0.01779600182615102485, -0.08955987627499310821, 0.2207522308509031472 ) ) ;
#8095=CARTESIAN_POINT ( 'NONE',  ( 0.1787899950787401882, -1.728962550906403495, -2.189545951927503898E-17 ) ) ;
#8102=CARTESIAN_POINT ( 'NONE',  ( 0.1787899950787401882, -1.363681102308440973, -2.189545951927503898E-17 ) ) ;
#8103=CARTESIAN_POINT ( 'NONE',  ( 3.284318927891251994E-17, -1.565452755851747924, 0.1787899950787401882 ) ) ;
#8112=ORIENTED_EDGE ( 'NONE', *, *, #47127, .F. ) ;
#8117=CARTESIAN_POINT ( 'NONE',  ( -0.1649531470039379555, -0.08956211461529646478, 0.02954168907489855556 ) ) ;
#8120=AXIS2_PLACEMENT_3D ( 'NONE', #14672, #3640, #20 ) ;
#8125=CARTESIAN_POINT ( 'NONE',  ( 0.07405724077823318263, -1.523622047190330564, 0.1787899950787401604 ) ) ;
#8126=CARTESIAN_POINT ( 'NONE',  ( 3.284318927891251994E-17, -0.9404527558517480346, 0.1787899950787401882 ) ) ;
#8127=CARTESIAN_POINT ( 'NONE',  ( -0.1113553986120547346, -1.174212598425196985, -0.1113553986120547346 ) ) ;
#8132=ORIENTED_EDGE ( 'NONE', *, *, #31532, .F. ) ;
#8135=CARTESIAN_POINT ( 'NONE',  ( 2.892866454678787531E-17, -1.346456692805858113, 0.1574803149606299191 ) ) ;
#8147=CARTESIAN_POINT ( 'NONE',  ( -0.1299735959408482300, -0.09851383385443740481, 0.1030069632188811007 ) ) ;
#8154=CARTESIAN_POINT ( 'NONE',  ( -0.1787899950787401604, -0.8740157479777336258, -0.07405724077823318263 ) ) ;
#8156=CARTESIAN_POINT ( 'NONE',  ( -1.094772975963752103E-17, -1.073326771599779628, -0.1787899950787401882 ) ) ;
#8158=CARTESIAN_POINT ( 'NONE',  ( 0.1797182628040039365, -0.2963036521027306858, -2.200913952912460540E-17 ) ) ;
#8160=CARTESIAN_POINT ( 'NONE',  ( -0.1574803149606299191, 0.09055118110236221041, 0.000000000000000000 ) ) ;
#8161=CARTESIAN_POINT ( 'NONE',  ( 3.284318927891251994E-17, -0.1924212597887563214, 0.1787899950787401882 ) ) ;
#8166=SURFACE_SIDE_STYLE ('',( #29795 ) ) ;
#8172=CARTESIAN_POINT ( 'NONE',  ( -0.06523048226347956391, -0.9552165353255434033, 0.1574803149606297803 ) ) ;
#8173=CARTESIAN_POINT ( 'NONE',  ( 0.07405724077823318263, -0.3326771653005671237, -0.1787899950787401604 ) ) ;
#8175=CARTESIAN_POINT ( 'NONE',  ( 3.284318927891251994E-17, -1.250492125930488196, 0.1787899950787401882 ) ) ;
#8187=CARTESIAN_POINT ( 'NONE',  ( -0.07818037259012035334, -0.09842482883889538958, -0.1607972800070663622 ) ) ;
#8200=CARTESIAN_POINT ( 'NONE',  ( -0.2160974785307145929, -0.09851385176812245403, -0.1192534063745566836 ) ) ;
#8205=CARTESIAN_POINT ( 'NONE',  ( -0.1264236179284866091, -1.468135779252860207, 0.1264236179284866091 ) ) ;
#8207=CARTESIAN_POINT ( 'NONE',  ( 0.1264236179284866091, -0.4975393700249764461, 0.1264236179284866091 ) ) ;
#8211=DIRECTION ( 'NONE',  ( 0.000000000000000000, 1.000000000000000000, 0.000000000000000000 ) ) ;
#8220=CARTESIAN_POINT ( 'NONE',  ( 0.07405724077823318263, 0.1140492601172180265, 0.1787899950787401604 ) ) ;
#8221=CARTESIAN_POINT ( 'NONE',  ( -0.1787899950787401882, -1.732775590497417362, 0.000000000000000000 ) ) ;
#8225=CARTESIAN_POINT ( 'NONE',  ( 0.1574803149606300301, -0.6796259842519688510, 0.06523048226347956391 ) ) ;
#8227=CARTESIAN_POINT ( 'NONE',  ( 0.1270800023317771588, -1.472484754464935097, -0.1270800023317771588 ) ) ;
#8244=VECTOR ( 'NONE', #3216, 39.37007874015748143 ) ;
#8251=CARTESIAN_POINT ( 'NONE',  ( -0.1797182628040039087, -0.08222884895312435050, -0.07444174185955065859 ) ) ;
#8252=CARTESIAN_POINT ( 'NONE',  ( -0.1787899950787401882, -1.225885826717889815, 0.000000000000000000 ) ) ;
#8257=CARTESIAN_POINT ( 'NONE',  ( -0.1113553986120547346, 0.04625984251968504046, -0.1113553986120547346 ) ) ;
#8265=CARTESIAN_POINT ( 'NONE',  ( 2.892866454678787531E-17, -0.08661417312081949593, 0.1574803149606299191 ) ) ;
#8271=CARTESIAN_POINT ( 'NONE',  ( -0.1787899950787401604, -0.9637066453945932754, -0.07405724077823318263 ) ) ;
#8273=CARTESIAN_POINT ( 'NONE',  ( 0.1264236179284866091, 0.01427165359707059308, 0.1264236179284866091 ) ) ;
#8280=CARTESIAN_POINT ( 'NONE',  ( -0.1787899950787401604, -0.5147637794737950356, 0.07405724077823318263 ) ) ;
#8284=CARTESIAN_POINT ( 'NONE',  ( 0.07444174185955065859, -1.012346959189344808, 0.1797182628040039087 ) ) ;
#8296=CARTESIAN_POINT ( 'NONE',  ( 0.1264236179284866091, -0.7632874015210393548, -0.1264236179284866091 ) ) ;
#8302=CARTESIAN_POINT ( 'NONE',  ( 0.06523048226347956391, -1.708169291338582418, 0.1574803149606297803 ) ) ;
#8306=ORIENTED_EDGE ( 'NONE', *, *, #40190, .F. ) ;
#8311=CARTESIAN_POINT ( 'NONE',  ( -1.094772975963752103E-17, 0.1028543307624250058, -0.1787899950787401882 ) ) ;
#8312=CARTESIAN_POINT ( 'NONE',  ( 0.1113553986120547346, -0.3474409447743626589, -0.1113553986120547346 ) ) ;
#8313=CARTESIAN_POINT ( 'NONE',  ( 0.1264236179284866091, -1.565452755851747924, 0.1264236179284866091 ) ) ;
#8321=CARTESIAN_POINT ( 'NONE',  ( -0.1787899950787401604, -0.6044546768906556844, 0.07405724077823318263 ) ) ;
#8322=CARTESIAN_POINT ( 'NONE',  ( -0.2379558572308452802, -0.08955967549845886277, -0.02966404366025586839 ) ) ;
#8337=CARTESIAN_POINT ( 'NONE',  ( 0.1264236179284866091, -1.319389763725763665, -0.1264236179284866091 ) ) ;
#8338=CARTESIAN_POINT ( 'NONE',  ( -0.1787899950787401882, -1.496555118056472677, 0.000000000000000000 ) ) ;
#8346=CARTESIAN_POINT ( 'NONE',  ( 0.06523048226347956391, -0.2908464566929132578, 0.1574803149606297803 ) ) ;
#8353=CARTESIAN_POINT ( 'NONE',  ( 0.000000000000000000, -0.09842519685039370636, 0.000000000000000000 ) ) ;
#8354=CARTESIAN_POINT ( 'NONE',  ( -0.1574803149606297803, -0.5664370077664889758, 0.06523048226347956391 ) ) ;
#8357=CARTESIAN_POINT ( 'NONE',  ( -0.1697987809117319224, -0.08954398017175399516, -0.008892717904794893158 ) ) ;
#8364=CARTESIAN_POINT ( 'NONE',  ( 0.1264236179284866091, -1.718011810969858333, 0.1264236179284866091 ) ) ;
#8365=CARTESIAN_POINT ( 'NONE',  ( 0.1787899950787401604, -0.8494094487651332459, -0.07405724077823318263 ) ) ;
#8366=CARTESIAN_POINT ( 'NONE',  ( 0.1574803149606300301, -1.191437007874017073, 0.06523048226347956391 ) ) ;
#8379=CARTESIAN_POINT ( 'NONE',  ( 0.09216395708618058125, 0.09383642490574123363, 0.2322221854328543611 ) ) ;
#8386=CARTESIAN_POINT ( 'NONE',  ( -0.1222548325031484334, -0.09842519685039370636, 0.1962412971452039412 ) ) ;
#8396=CARTESIAN_POINT ( 'NONE',  ( -0.1787899950787401604, -0.9478346456155283262, 0.07405724077823318263 ) ) ;
#8397=CARTESIAN_POINT ( 'NONE',  ( -0.07405724077823318263, -1.056102362150961982, 0.1787899950787401604 ) ) ;
#8401=CARTESIAN_POINT ( 'NONE',  ( -0.1113553986120547346, 0.1250000000000000000, -0.1113553986120547346 ) ) ;
#8402=CARTESIAN_POINT ( 'NONE',  ( 0.1264236179284866091, -0.1776574802611972648, -0.1264236179284866091 ) ) ;
#8412=CARTESIAN_POINT ( 'NONE',  ( -0.1264236179284866091, -0.3941929133320630219, 0.1264236179284866091 ) ) ;
#8414=CARTESIAN_POINT ( 'NONE',  ( 3.284318927891251994E-17, -1.211122047190330786, 0.1787899950787401882 ) ) ;
#8425=CARTESIAN_POINT ( 'NONE',  ( 0.02009753640170339889, -0.09839439123163033762, -0.1777236764612983022 ) ) ;
#8443=CARTESIAN_POINT ( 'NONE',  ( 0.07405724077823318263, -1.485360188701679629, -0.1787899950787401604 ) ) ;
#8445=CARTESIAN_POINT ( 'NONE',  ( -0.07405724077823318263, -0.4803149605761579677, -0.1787899950787401604 ) ) ;
#8454=CARTESIAN_POINT ( 'NONE',  ( -0.07405724077823318263, -1.809055118056471123, 0.1787899950787401604 ) ) ;
#8455=CARTESIAN_POINT ( 'NONE',  ( -0.1787899950787401882, 0.1126968504474643862, 0.000000000000000000 ) ) ;
#8459=CARTESIAN_POINT ( 'NONE',  ( -0.06523048226347956391, -0.6894685039370073154, 0.1574803149606297803 ) ) ;
#8461=CARTESIAN_POINT ( 'NONE',  ( 0.07444174185955065859, -1.484787904071234843, 0.1797182628040039087 ) ) ;
#8463=CARTESIAN_POINT ( 'NONE',  ( 0.1574803149606300301, -0.4335629920184572161, 0.06523048226347956391 ) ) ;
#8472=CARTESIAN_POINT ( 'NONE',  ( 0.1787899950787401604, -0.02263779522182706935, -0.07405724077823318263 ) ) ;
#8484=CARTESIAN_POINT ( 'NONE',  ( -0.1270800023317771588, 0.003893198290970204586, 0.1270800023317771588 ) ) ;
#8485=CARTESIAN_POINT ( 'NONE',  ( -0.1264236179284866091, -1.270177165300566902, -0.1264236179284866091 ) ) ;
#8497=CARTESIAN_POINT ( 'NONE',  ( -0.08995663987708611697, -0.09317336072452847562, -0.2334965874938852715 ) ) ;
#8501=CARTESIAN_POINT ( 'NONE',  ( -0.1113553986120547346, -0.09153543296333917223, 0.1113553986120547346 ) ) ;
#8505=( BOUNDED_CURVE ( )  B_SPLINE_CURVE ( 2, ( #37811, #4724, #41596, #11711, #4964, #30189, #19591, #12178, #19348 ),
 .UNSPECIFIED., .F., .T. ) 
 B_SPLINE_CURVE_WITH_KNOTS ( ( 3, 2, 2, 2, 3 ),
 ( 0.04499999999999999833, 0.04750000000000000056, 0.05000000000000000278, 0.05249999999999999806, 0.05500000000000000028 ),
 .UNSPECIFIED. ) 
 CURVE ( )  GEOMETRIC_REPRESENTATION_ITEM ( )  RATIONAL_B_SPLINE_CURVE ( ( 1.000000000000000000, 0.9238795325112869605, 1.000000000000000000, 0.9238795325112869605, 1.000000000000000000, 0.9238795325112869605, 1.000000000000000000, 0.9238795325112869605, 1.000000000000000000 ) ) 
 REPRESENTATION_ITEM ( '' )  ) ;
#8509=CARTESIAN_POINT ( 'NONE',  ( -0.1787899950787401604, -0.9981554642922296772, 0.07405724077823318263 ) ) ;
#8511=CARTESIAN_POINT ( 'NONE',  ( -0.07405724077823318263, 0.03149606304588949135, -0.1787899950787401604 ) ) ;
#8519=CARTESIAN_POINT ( 'NONE',  ( 0.1787899950787401882, -0.6943897637257637756, -2.189545951927503898E-17 ) ) ;
#8523=CARTESIAN_POINT ( 'NONE',  ( -0.07444174185955065859, -0.9385280615515501079, 0.1797182628040039087 ) ) ;
#8532=CARTESIAN_POINT ( 'NONE',  ( -0.07405724077823318263, 0.07086614178604697112, -0.1787899950787401604 ) ) ;
#8536=CARTESIAN_POINT ( 'NONE',  ( -0.07405724077823318263, -0.9773622046706458288, 0.1787899950787401604 ) ) ;
#8538=PLANE ( 'NONE',  #12311 ) ;
#8540=CARTESIAN_POINT ( 'NONE',  ( -0.1574803149606299191, -1.710629921152315047, 0.000000000000000000 ) ) ;
#8545=CARTESIAN_POINT ( 'NONE',  ( -0.06523048226347956391, -1.752460629921259505, 0.1574803149606297803 ) ) ;
#8551=CARTESIAN_POINT ( 'NONE',  ( -0.1787899950787401604, -1.499015747977732627, 0.07405724077823318263 ) ) ;
#8561=CARTESIAN_POINT ( 'NONE',  ( 0.1787899950787401882, -0.5478601887016795180, -2.189545951927503898E-17 ) ) ;
#8562=CARTESIAN_POINT ( 'NONE',  ( -0.03314229022649078926, -0.08955993585198464280, 0.2197241657068637610 ) ) ;
#8565=CYLINDRICAL_SURFACE ( 'NONE', #3501, 0.1574803149606299191 ) ;
#8567=CARTESIAN_POINT ( 'NONE',  ( 0.07405724077823318263, -1.800320818622939356, -0.1787899950787401604 ) ) ;
#8570=CARTESIAN_POINT ( 'NONE',  ( -0.1787899950787401604, -1.346456692859623550, -0.07405724077823318263 ) ) ;
#8572=CARTESIAN_POINT ( 'NONE',  ( -0.1787899950787401604, -1.499015747977732627, -0.07405724077823318263 ) ) ;
#8579=CARTESIAN_POINT ( 'NONE',  ( -0.1113553986120547346, -0.3474409448818897572, -0.1113553986120547346 ) ) ;
#8591=CARTESIAN_POINT ( 'NONE',  ( -0.1330426644874648789, -0.08955887018083319440, 0.09370495055536537388 ) ) ;
#8592=EDGE_LOOP ( 'NONE', ( #585, #35958, #30435 ) ) ;
#8599=CARTESIAN_POINT ( 'NONE',  ( -0.1787899950787401604, -1.735236220418678643, -0.07405724077823318263 ) ) ;
#8600=CARTESIAN_POINT ( 'NONE',  ( 0.07405724077823318263, -0.8444881889226140137, -0.1787899950787401604 ) ) ;
#8601=CARTESIAN_POINT ( 'NONE',  ( -0.1113553986120547346, -1.203740157480315043, 0.1113553986120547346 ) ) ;
#8625=CARTESIAN_POINT ( 'NONE',  ( -0.1150404479467348473, -0.09851383574764233098, 0.1176134116418862258 ) ) ;
#8631=CARTESIAN_POINT ( 'NONE',  ( -0.1787899950787401882, -0.9109251967966299768, 0.000000000000000000 ) ) ;
#8634=CARTESIAN_POINT ( 'NONE',  ( 0.1787899950787401604, -1.001968503883243988, -0.07405724077823318263 ) ) ;
#8636=CARTESIAN_POINT ( 'NONE',  ( -0.1270800023317771588, -0.3504375103704472361, 0.1270800023317771588 ) ) ;
#8648=DIRECTION ( 'NONE',  ( 0.000000000000000000, 0.000000000000000000, 1.000000000000000000 ) ) ;
#8649=CARTESIAN_POINT ( 'NONE',  ( 0.07405724077823318263, -0.4655511810485986057, 0.1787899950787401604 ) ) ;
#8650=CARTESIAN_POINT ( 'NONE',  ( -0.07405724077823318263, -1.213582677111591623, 0.1787899950787401604 ) ) ;
#8661=CARTESIAN_POINT ( 'NONE',  ( 0.06548250281709126763, -0.09842519584946800293, -0.1663669883860420806 ) ) ;
#8681=CARTESIAN_POINT ( 'NONE',  ( -1.094772975963752103E-17, -1.482899558780419458, -0.1787899950787401882 ) ) ;
#8684=CARTESIAN_POINT ( 'NONE',  ( -0.1787899950787401604, -0.3917322834108032947, 0.07405724077823318263 ) ) ;
#8690=CARTESIAN_POINT ( 'NONE',  ( 0.1264236179284866091, -0.2268700786863941110, 0.1264236179284866091 ) ) ;
#8694=CARTESIAN_POINT ( 'NONE',  ( 0.07405724077823318263, -1.764763779473795813, 0.1787899950787401604 ) ) ;
#8700=CARTESIAN_POINT ( 'NONE',  ( -0.1113553986120547346, -0.7017716535433071723, -0.1113553986120547346 ) ) ;
#8702=CARTESIAN_POINT ( 'NONE',  ( 0.1270800023317771588, -1.511854833205092286, -0.1270800023317771588 ) ) ;
#8714=CARTESIAN_POINT ( 'NONE',  ( 0.1787899950787401604, 0.09055118115612580121, 0.07405724077823318263 ) ) ;
#8723=CARTESIAN_POINT ( 'NONE',  ( 0.06523048226347956391, -0.05462598425196848323, 0.1574803149606297803 ) ) ;
#8735=ORIENTED_EDGE ( 'NONE', *, *, #4876, .T. ) ;
#8741=CARTESIAN_POINT ( 'NONE',  ( -0.06523048226347956391, -0.06446850382948084157, -0.1574803149606300301 ) ) ;
#8745=CARTESIAN_POINT ( 'NONE',  ( -0.1787899950787401604, -0.9587853855520737101, 0.07405724077823318263 ) ) ;
#8747=CARTESIAN_POINT ( 'NONE',  ( -0.1787899950787401604, 0.07578740162856664742, -0.07405724077823318263 ) ) ;
#8752=AXIS2_PLACEMENT_3D ( 'NONE', #41547, #41794, #31293 ) ;
#8754=CARTESIAN_POINT ( 'NONE',  ( 0.1264236179284866091, -0.6500984251430865779, -0.1264236179284866091 ) ) ;
#8760=CARTESIAN_POINT ( 'NONE',  ( -0.1797182628040039087, -1.105850896197218658, -0.07444174185955065859 ) ) ;
#8761=CARTESIAN_POINT ( 'NONE',  ( 0.1701422387595818708, 0.1299212598425197041, 0.05395700737448459045 ) ) ;
#8765=EDGE_CURVE ( 'NONE', #24004, #23021, #36381, .T. ) ;
#8770=CARTESIAN_POINT ( 'NONE',  ( 2.892866454678787531E-17, -0.09645669291338582196, 0.1574803149606299191 ) ) ;
#8772=CARTESIAN_POINT ( 'NONE',  ( -1.094772975963752103E-17, 0.06840551186478720236, -0.1787899950787401882 ) ) ;
#8780=CARTESIAN_POINT ( 'NONE',  ( -0.06523048226347956391, -1.703248031388535866, 0.1574803149606297803 ) ) ;
#8786=CARTESIAN_POINT ( 'NONE',  ( 0.07405724077823318263, 0.1446850394238423654, -0.1787899950787401604 ) ) ;
#8792=CARTESIAN_POINT ( 'NONE',  ( 0.06523048226347956391, -0.3449803148531030983, -0.1574803149606300301 ) ) ;
#8793=CARTESIAN_POINT ( 'NONE',  ( 0.07405724077823318263, -1.607283464513165949, 0.1787899950787401604 ) ) ;
#8799=CARTESIAN_POINT ( 'NONE',  ( 0.07405724077823318263, -0.5404782989379000036, -0.1787899950787401604 ) ) ;
#8800=CARTESIAN_POINT ( 'NONE',  ( 0.1203886723041954626, -0.08956011358862403515, 0.1770541383337161656 ) ) ;
#8805=CARTESIAN_POINT ( 'NONE',  ( -1.094772975963752103E-17, -1.797860188701681183, -0.1787899950787401882 ) ) ;
#8810=CARTESIAN_POINT ( 'NONE',  ( -0.1264236179284866091, -1.506397637741511586, -0.1264236179284866091 ) ) ;
#8811=CARTESIAN_POINT ( 'NONE',  ( -0.1545411696117860445, -0.09842519685039370636, -0.08990488994085453489 ) ) ;
#8815=ORIENTED_EDGE ( 'NONE', *, *, #29231, .T. ) ;
#8823=CARTESIAN_POINT ( 'NONE',  ( -0.1574803149606300301, -0.4237204724409446288, -0.06523048226347956391 ) ) ;
#8836=CARTESIAN_POINT ( 'NONE',  ( -0.1066074665795045118, -0.08956136683350990335, 0.1197088631414433141 ) ) ;
#8837=CARTESIAN_POINT ( 'NONE',  ( -0.07405724077823318263, -0.5049212597887556830, 0.1787899950787401604 ) ) ;
#8838=ORIENTED_EDGE ( 'NONE', *, *, #15216, .T. ) ;
#8842=CARTESIAN_POINT ( 'NONE',  ( -0.1235961452251413406, 0.09842519685039370636, -0.2140748031496062798 ) ) ;
#8844=CARTESIAN_POINT ( 'NONE',  ( -0.1787899950787401604, -1.774606299158834277, -0.07405724077823318263 ) ) ;
#8845=CARTESIAN_POINT ( 'NONE',  ( -0.1787899950787401882, -0.8715551180564724554, 0.000000000000000000 ) ) ;
#8846=CARTESIAN_POINT ( 'NONE',  ( -9.642888182262618425E-18, -1.336614173228346525, -0.1574803149606299191 ) ) ;
#8856=CARTESIAN_POINT ( 'NONE',  ( -0.1574803149606300301, -1.398129921152315935, -0.06523048226347956391 ) ) ;
#8860=VECTOR ( 'NONE', #22449, 39.37007874015748143 ) ;
#8867=CARTESIAN_POINT ( 'NONE',  ( -0.2471922904502826812, 0.03219022224904106305, 0.1427165354330708902 ) ) ;
#8870=CARTESIAN_POINT ( 'NONE',  ( 0.05241428596829866143, -0.09842519685039370636, -0.1860699077350574659 ) ) ;
#8878=CARTESIAN_POINT ( 'NONE',  ( -0.1787899950787401882, -0.9896653542769447975, 0.000000000000000000 ) ) ;
#8879=CARTESIAN_POINT ( 'NONE',  ( 0.07405724077823318263, -1.129921259788756682, 0.1787899950787401604 ) ) ;
#8882=CARTESIAN_POINT ( 'NONE',  ( -0.1797182628040039365, -0.3159886914728094465, 0.000000000000000000 ) ) ;
#8884=CARTESIAN_POINT ( 'NONE',  ( 0.1574803149606300301, -0.01033464566929132716, 0.06523048226347956391 ) ) ;
#8895=CARTESIAN_POINT ( 'NONE',  ( -0.1787899950787401882, -0.4778543306548976854, 0.000000000000000000 ) ) ;
#8897=CARTESIAN_POINT ( 'NONE',  ( 0.1787899950787401604, -1.198818897584032150, -0.07405724077823318263 ) ) ;
#8904=CARTESIAN_POINT ( 'NONE',  ( -0.1574803149606297803, -1.235728346349166840, 0.06523048226347956391 ) ) ;
#8907=CARTESIAN_POINT ( 'NONE',  ( 0.05897220410447782252, -0.09842522462652292248, -0.1687951425607464584 ) ) ;
#8912=CARTESIAN_POINT ( 'NONE',  ( -0.1006676817871263313, -0.09658349877441908815, 0.2273124399503319293 ) ) ;
#8913=CARTESIAN_POINT ( 'NONE',  ( -9.642888182262618425E-18, -0.07677165354330708902, -0.1574803149606299191 ) ) ;
#8918=CARTESIAN_POINT ( 'NONE',  ( -0.1275811598217675147, -0.09851385249697934554, -0.2189343593283228084 ) ) ;
#8926=CARTESIAN_POINT ( 'NONE',  ( -0.07405724077823318263, -1.583785385552072489, 0.1787899950787401604 ) ) ;
#8929=CARTESIAN_POINT ( 'NONE',  ( -0.1264236179284866091, -0.4778543306548976854, -0.1264236179284866091 ) ) ;
#8934=CARTESIAN_POINT ( 'NONE',  ( -0.1787899950787401604, -0.2440944881352131168, -0.07405724077823318263 ) ) ;
#8937=CARTESIAN_POINT ( 'NONE',  ( 0.1264236179284866091, 0.1263524097235171340, -0.1264236179284866091 ) ) ;
#8938=CARTESIAN_POINT ( 'NONE',  ( 0.1264236179284866091, -1.796751968450173376, 0.1264236179284866091 ) ) ;
#8940=CARTESIAN_POINT ( 'NONE',  ( 0.1335170321881475330, -0.09842519685039372024, 0.1069600103855054690 ) ) ;
#8945=CARTESIAN_POINT ( 'NONE',  ( -0.1113553986120547346, -0.6919291338582677087, 0.1113553986120547346 ) ) ;
#8947=CARTESIAN_POINT ( 'NONE',  ( 0.07444174185955046430, -1.588134360764147601, -0.1797182628040039087 ) ) ;
#8949=CARTESIAN_POINT ( 'NONE',  ( 0.07405724077823318263, -0.3671259841982050798, -0.1787899950787401604 ) ) ;
#8957=CARTESIAN_POINT ( 'NONE',  ( 0.07405724077823318263, 0.08562992131360593062, 0.1787899950787401604 ) ) ;
#8967=CARTESIAN_POINT ( 'NONE',  ( 0.07405724077823318263, -1.371062992072219489, 0.1787899950787401604 ) ) ;
#8981=CARTESIAN_POINT ( 'NONE',  ( 0.06523048226347956391, -0.06938976367200050399, -0.1574803149606300301 ) ) ;
#8987=CARTESIAN_POINT ( 'NONE',  ( -0.1787899950787401882, -1.118726330433962524, 0.000000000000000000 ) ) ;
#8989=CARTESIAN_POINT ( 'NONE',  ( -0.1264236179284866091, 0.04379921265218866822, 0.1264236179284866091 ) ) ;
#8997=CARTESIAN_POINT ( 'NONE',  ( 0.07405724077823318263, -0.6082677164816695514, -0.1787899950787401604 ) ) ;
#9001=CARTESIAN_POINT ( 'NONE',  ( 3.301370929368692659E-17, -1.132917825331076767, 0.1797182628040039365 ) ) ;
#9002=CARTESIAN_POINT ( 'NONE',  ( 0.1651804164989524593, 0.1299212598425196763, 0.06841997037041555596 ) ) ;
#9009=CARTESIAN_POINT ( 'NONE',  ( 0.1113553986120547346, -0.7116141731208188714, 0.1113553986120547346 ) ) ;
#9019=CARTESIAN_POINT ( 'NONE',  ( -0.06523048226347956391, -1.639271653435778964, -0.1574803149606300301 ) ) ;
#9024=CARTESIAN_POINT ( 'NONE',  ( -0.1787899950787401604, 0.07578740162856664742, -0.07405724077823318263 ) ) ;
#9028=CARTESIAN_POINT ( 'NONE',  ( -0.04076295239693389361, 0.06762482675903896956, 0.2618985693268079396 ) ) ;
#9032=CARTESIAN_POINT ( 'NONE',  ( -0.1113553986120547346, -0.3769685038294807167, -0.1113553986120547346 ) ) ;
#9033=CARTESIAN_POINT ( 'NONE',  ( 0.07405724077823318263, -1.567913385773008095, 0.1787899950787401604 ) ) ;
#9044=CARTESIAN_POINT ( 'NONE',  ( 0.1787899950787401882, -0.5872302674418370394, -2.189545951927503898E-17 ) ) ;
#9045=CARTESIAN_POINT ( 'NONE',  ( 0.1441055234924401574, -0.08955999847834450467, 0.1574950935048799183 ) ) ;
#9053=CARTESIAN_POINT ( 'NONE',  ( 0.2471921406147994105, -0.06698952652786568929, 0.09859233283899719591 ) ) ;
#9055=CARTESIAN_POINT ( 'NONE',  ( 0.1264236179284866091, -1.486712598371433103, 0.1264236179284866091 ) ) ;
#9060=CARTESIAN_POINT ( 'NONE',  ( 0.1797182628040039087, -0.7269138883232022508, -0.07444174185955065859 ) ) ;
#9065=CARTESIAN_POINT ( 'NONE',  ( -0.1113553986120547346, -0.4950787401574803237, 0.1113553986120547346 ) ) ;
#9068=ORIENTED_EDGE ( 'NONE', *, *, #38837, .F. ) ;
#9071=DIRECTION ( 'NONE',  ( 0.000000000000000000, 0.000000000000000000, 1.000000000000000000 ) ) ;
#9073=CARTESIAN_POINT ( 'NONE',  ( -0.1113553986120547346, -0.5738188975302677131, -0.1113553986120547346 ) ) ;
#9078=CARTESIAN_POINT ( 'NONE',  ( 0.1787899950787401604, -0.5344488188438744070, 0.07405724077823318263 ) ) ;
#9085=CARTESIAN_POINT ( 'NONE',  ( 3.284318927891251994E-17, -1.683562992072220599, 0.1787899950787401882 ) ) ;
#9086=CARTESIAN_POINT ( 'NONE',  ( 3.284318927891251994E-17, -0.8617125983714329918, 0.1787899950787401882 ) ) ;
#9087=CARTESIAN_POINT ( 'NONE',  ( 0.1574803149606300301, -1.388287401574803015, 0.06523048226347956391 ) ) ;
#9091=ORIENTED_EDGE ( 'NONE', *, *, #28013, .F. ) ;
#9107=CARTESIAN_POINT ( 'NONE',  ( -7.939671275311751530E-17, -0.03219022224904082713, -0.2854330708661417804 ) ) ;
#9111=CARTESIAN_POINT ( 'NONE',  ( 0.2057643835732720639, -0.09842519685039370636, -0.01601721728994680988 ) ) ;
#9118=CARTESIAN_POINT ( 'NONE',  ( -0.1787899950787401604, -1.026574803095842370, 0.07405724077823318263 ) ) ;
#9120=CARTESIAN_POINT ( 'NONE',  ( 3.284318927891251994E-17, -1.171751968450173154, 0.1787899950787401882 ) ) ;
#9124=CARTESIAN_POINT ( 'NONE',  ( -1.100456976456230270E-17, -0.5226816048586362395, -0.1797182628040039365 ) ) ;
#9126=CARTESIAN_POINT ( 'NONE',  ( 2.892866454678787531E-17, -0.05708661417322834220, 0.1574803149606299191 ) ) ;
#9132=CARTESIAN_POINT ( 'NONE',  ( 0.1264236179284866091, -0.4532480314422991929, -0.1264236179284866091 ) ) ;
#9134=CARTESIAN_POINT ( 'NONE',  ( 3.284318927891251994E-17, -1.407972440891118282, 0.1787899950787401882 ) ) ;
#9149=CARTESIAN_POINT ( 'NONE',  ( 0.1766724065111454356, -0.08549467455806485094, -0.1834299084079261122 ) ) ;
#9155=CARTESIAN_POINT ( 'NONE',  ( -0.1397933335164911473, -0.09851385033795964641, 0.1854247136317299371 ) ) ;
#9162=CARTESIAN_POINT ( 'NONE',  ( 0.1787899950787401604, -1.569021606024515014, -0.07405724077823318263 ) ) ;
#9165=CARTESIAN_POINT ( 'NONE',  ( -0.1264236179284866091, -0.5565944881352126172, -0.1264236179284866091 ) ) ;
#9172=CARTESIAN_POINT ( 'NONE',  ( -0.07405724077823318263, -0.02374601547333323251, -0.1787899950787401604 ) ) ;
#9173=CARTESIAN_POINT ( 'NONE',  ( -1.094772975963752103E-17, -1.781988188922614347, -0.1787899950787401882 ) ) ;
#9180=CARTESIAN_POINT ( 'NONE',  ( 0.1574803149606300301, -0.9158464566929129802, 0.06523048226347956391 ) ) ;
#9182=CARTESIAN_POINT ( 'NONE',  ( -0.1270800023317771588, -1.541382392260210565, -0.1270800023317771588 ) ) ;
#9184=CARTESIAN_POINT ( 'NONE',  ( 0.07405724077823318263, -0.4064960629383624346, -0.1787899950787401604 ) ) ;
#9191=CARTESIAN_POINT ( 'NONE',  ( -0.1787899950787401604, 0.03641732288840918152, 0.07405724077823318263 ) ) ;
#9202=CARTESIAN_POINT ( 'NONE',  ( -0.1574803149606297803, -1.078248031388536754, 0.06523048226347956391 ) ) ;
#9203=CARTESIAN_POINT ( 'NONE',  ( 0.1264236179284866091, -1.398129921206078707, -0.1264236179284866091 ) ) ;
#9215=EDGE_CURVE ( 'NONE', #7112, #44436, #8505, .T. ) ;
#9217=CARTESIAN_POINT ( 'NONE',  ( 3.284318927891251994E-17, 0.1225393701325037388, 0.1787899950787401882 ) ) ;
#9218=CARTESIAN_POINT ( 'NONE',  ( -0.06175619828051706617, -0.08093302715459128882, -0.2497778431879683070 ) ) ;
#9222=CARTESIAN_POINT ( 'NONE',  ( 0.1113553986120547346, -0.1998031494987720369, 0.1113553986120547346 ) ) ;
#9229=CARTESIAN_POINT ( 'NONE',  ( -0.1264236179284866091, -1.163017669016639832, -0.1264236179284866091 ) ) ;
#9231=CARTESIAN_POINT ( 'NONE',  ( 0.1264236179284866091, -0.1727362204186775607, -0.1264236179284866091 ) ) ;
#9237=CARTESIAN_POINT ( 'NONE',  ( -0.07405724077823318263, -0.6673228345919050009, 0.1787899950787401604 ) ) ;
#9242=CARTESIAN_POINT ( 'NONE',  ( -0.1797182628040039087, -1.179669793835013358, 0.07444174185955065859 ) ) ;
#9251=CARTESIAN_POINT ( 'NONE',  ( 0.06523048226347956391, -0.7386811022546784233, -0.1574803149606300301 ) ) ;
#9261=CARTESIAN_POINT ( 'NONE',  ( 0.1574803149606300301, -1.649114173120819649, -0.06523048226347956391 ) ) ;
#9264=CARTESIAN_POINT ( 'NONE',  ( 0.07405724077823318263, -0.09153543301710270752, -0.1787899950787401604 ) ) ;
#9267=CARTESIAN_POINT ( 'NONE',  ( -0.1787899950787401604, 0.08070866147108628208, 0.07405724077823318263 ) ) ;
#9275=CARTESIAN_POINT ( 'NONE',  ( 3.284318927891251994E-17, -1.727854330654897685, 0.1787899950787401882 ) ) ;
#9278=ORIENTED_EDGE ( 'NONE', *, *, #32814, .T. ) ;
#9285=CARTESIAN_POINT ( 'NONE',  ( 0.1787899950787401604, -0.7471712123237258529, 0.07405724077823318263 ) ) ;
#9287=CARTESIAN_POINT ( 'NONE',  ( -0.1531176995717757894, -0.08956120967700866020, -0.08476774985902559012 ) ) ;
#9297=CARTESIAN_POINT ( 'NONE',  ( -1.094772975963752103E-17, -1.432578740103716664, -0.1787899950787401882 ) ) ;
#9300=CARTESIAN_POINT ( 'NONE',  ( -0.1797182628040039087, -0.7465989276932815111, 0.07444174185955065859 ) ) ;
#9303=CARTESIAN_POINT ( 'NONE',  ( 2.892866454678787531E-17, -0.4114173228346456601, 0.1574803149606299191 ) ) ;
#9311=CARTESIAN_POINT ( 'NONE',  ( 0.1574803149606300301, 0.08316929144610965552, -0.06523048226347956391 ) ) ;
#9315=CARTESIAN_POINT ( 'NONE',  ( 0.1113553986120547346, -0.5935039369003465293, 0.1113553986120547346 ) ) ;
#9320=CARTESIAN_POINT ( 'NONE',  ( -1.094772975963752103E-17, -0.6008858267178898149, -0.1787899950787401882 ) ) ;
#9331=CARTESIAN_POINT ( 'NONE',  ( -0.1264236179284866091, -1.737696850339937038, -0.1264236179284866091 ) ) ;
#9332=CARTESIAN_POINT ( 'NONE',  ( 0.1787899950787401604, -1.085629921206079374, -0.07405724077823318263 ) ) ;
#9334=CARTESIAN_POINT ( 'NONE',  ( -9.642888182262618425E-18, -1.375984251968504157, -0.1574803149606299191 ) ) ;
#9341=ORIENTED_EDGE ( 'NONE', *, *, #35036, .T. ) ;
#9351=CARTESIAN_POINT ( 'NONE',  ( -0.1264236179284866091, -0.3264034957882941401, 0.1264236179284866091 ) ) ;
#9353=CARTESIAN_POINT ( 'NONE',  ( 0.03860301396976173471, -0.09842519685039370636, 0.2192022649856606165 ) ) ;
#9360=CARTESIAN_POINT ( 'NONE',  ( 0.07405724077823318263, -1.080708661363559919, -0.1787899950787401604 ) ) ;
#9361=CARTESIAN_POINT ( 'NONE',  ( -0.07405724077823318263, -1.213582677111591623, 0.1787899950787401604 ) ) ;
#9364=CARTESIAN_POINT ( 'NONE',  ( -0.1797182628040039365, -0.4734690064334394211, 0.000000000000000000 ) ) ;
#9365=CARTESIAN_POINT ( 'NONE',  ( -0.06523048226347956391, -1.796751968396409271, -0.1574803149606300301 ) ) ;
#9367=CARTESIAN_POINT ( 'NONE',  ( 0.1574803149606300301, 0.06840551181102358380, 0.06523048226347956391 ) ) ;
#9378=CARTESIAN_POINT ( 'NONE',  ( -0.07405724077823318263, -0.5098425196312756924, 0.1787899950787401604 ) ) ;
#9380=CARTESIAN_POINT ( 'NONE',  ( -0.1264236179284866091, -1.343996062938362268, -0.1264236179284866091 ) ) ;
#9391=CARTESIAN_POINT ( 'NONE',  ( 0.1776925020132069377, -0.09842519685039378963, -0.02072179724286548827 ) ) ;
#9394=B_SPLINE_CURVE_WITH_KNOTS ( 'NONE', 3,
 ( #25534, #34955, #2334, #28007, #40100, #38770, #35187, #77, #35423, #42352, #14725, #2561, #47068, #14259, #29398, #2100, #16730, #31366 ),
 .UNSPECIFIED., .F., .F.,
 ( 4, 2, 2, 2, 2, 2, 2, 2, 4 ),
 ( 0.000000000000000000, 0.1250000000000001110, 0.2500000000000002220, 0.5000000000000004441, 0.5625000000000003331, 0.6250000000000003331, 0.7500000000000002220, 0.8750000000000001110, 1.000000000000000000 ),
 .UNSPECIFIED. ) ;
#9395=CARTESIAN_POINT ( 'NONE',  ( 0.2471922904502826812, -0.03219022224904106305, 0.1427165354330708902 ) ) ;
#9403=CARTESIAN_POINT ( 'NONE',  ( -0.1713386234961888077, -0.09851385174780474818, 0.1582058536542151617 ) ) ;
#9406=CARTESIAN_POINT ( 'NONE',  ( 0.1787899950787401604, -1.608391684764673091, -0.07405724077823318263 ) ) ;
#9409=CARTESIAN_POINT ( 'NONE',  ( 0.07405724077823318263, -0.6427165353793066194, -0.1787899950787401604 ) ) ;
#9415=CARTESIAN_POINT ( 'NONE',  ( -0.1264236179284866091, -0.3646653542769452971, -0.1264236179284866091 ) ) ;
#9416=CARTESIAN_POINT ( 'NONE',  ( 0.07405724077823318263, -0.6968503936470246130, 0.1787899950787401604 ) ) ;
#9423=CARTESIAN_POINT ( 'NONE',  ( -1.094772975963752103E-17, 0.09190359082587953865, -0.1787899950787401882 ) ) ;
#9424=CARTESIAN_POINT ( 'NONE',  ( -0.07405724077823318263, 0.1200787402112438867, 0.1787899950787401604 ) ) ;
#9425=CARTESIAN_POINT ( 'NONE',  ( 0.09212567409445292232, -0.09842519685039373412, 0.1397575628899831168 ) ) ;
#9428=CARTESIAN_POINT ( 'NONE',  ( 0.1574803149606300301, -0.8321850393700797044, -0.06523048226347956391 ) ) ;
#9430=CARTESIAN_POINT ( 'NONE',  ( 0.1270800023317771588, -1.521697352890131638, 0.1270800023317771588 ) ) ;
#9432=CARTESIAN_POINT ( 'NONE',  ( 0.07405724077823318263, -0.3277559054580475584, -0.1787899950787401604 ) ) ;
#9435=CARTESIAN_POINT ( 'NONE',  ( 0.1550283333641064298, 0.09383642490574126138, -0.1959274208663558947 ) ) ;
#9443=CARTESIAN_POINT ( 'NONE',  ( 0.1113553986120547346, -0.8690944880814488460, 0.1113553986120547346 ) ) ;
#9444=CARTESIAN_POINT ( 'NONE',  ( -0.1787899950787401604, 0.07086614178604697112, -0.07405724077823318263 ) ) ;
#9446=CARTESIAN_POINT ( 'NONE',  ( -0.07405724077823318263, -0.9527559054580476694, -0.1787899950787401604 ) ) ;
#9475=CARTESIAN_POINT ( 'NONE',  ( 0.07405724077823318263, -1.091659401300105747, -0.1787899950787401604 ) ) ;
#9477=CARTESIAN_POINT ( 'NONE',  ( -0.1787899950787401604, -0.1948818897100161873, 0.07405724077823318263 ) ) ;
#9484=CARTESIAN_POINT ( 'NONE',  ( 0.07405724077823318263, -0.5836614172690718361, 0.1787899950787401604 ) ) ;
#9487=CARTESIAN_POINT ( 'NONE',  ( 0.07444174185955046430, -1.115693415882259121, -0.1797182628040039087 ) ) ;
#9495=CARTESIAN_POINT ( 'NONE',  ( -9.642888182262618425E-18, -0.7362204723334173639, -0.1574803149606299191 ) ) ;
#9503=CARTESIAN_POINT ( 'NONE',  ( -0.1574803149606297803, -1.708169291231055098, 0.06523048226347956391 ) ) ;
#9507=CARTESIAN_POINT ( 'NONE',  ( 0.09216094027010306167, -0.09383642490574117812, 0.2322237458739927762 ) ) ;
#9509=CARTESIAN_POINT ( 'NONE',  ( -0.07405724077823318263, 0.1102362205262043815, -0.1787899950787401604 ) ) ;
#9513=CARTESIAN_POINT ( 'NONE',  ( -0.08776479879009549401, 0.09247100924357742890, 0.2347620406593067532 ) ) ;
#9517=CARTESIAN_POINT ( 'NONE',  ( -0.1264236179284866091, -1.732775590497417362, 0.1264236179284866091 ) ) ;
#9525=CARTESIAN_POINT ( 'NONE',  ( 0.07405724077823318263, -0.6979586138985296451, -0.1787899950787401604 ) ) ;
#9527=CARTESIAN_POINT ( 'NONE',  ( 0.2038110898043921371, -0.08956021042321613002, 0.02011050427597645823 ) ) ;
#9542=CARTESIAN_POINT ( 'NONE',  ( 0.1797182628040039365, -0.6506343607641476012, -2.200913952912460540E-17 ) ) ;
#9543=CARTESIAN_POINT ( 'NONE',  ( 0.2471922904502826812, 0.07945684066378068400, 0.07439773916327693803 ) ) ;
#9546=CARTESIAN_POINT ( 'NONE',  ( 0.1113553986120547346, -0.3966535433070866312, -0.1113553986120547346 ) ) ;
#9547=CARTESIAN_POINT ( 'NONE',  ( -9.642888182262618425E-18, 0.04133858267716535029, -0.1574803149606299191 ) ) ;
#9550=CARTESIAN_POINT ( 'NONE',  ( 0.1574803149606299191, 0.03149606299212598381, -1.928577636452523993E-17 ) ) ;
#9559=CARTESIAN_POINT ( 'NONE',  ( -0.1264236179284866091, -0.5172244093950552069, -0.1264236179284866091 ) ) ;
#9563=CARTESIAN_POINT ( 'NONE',  ( 0.1651804164989524593, 0.1299212598425196763, 0.06841997037041555596 ) ) ;
#9569=CARTESIAN_POINT ( 'NONE',  ( 3.301370929368692659E-17, 0.08755461561380492586, 0.1797182628040039365 ) ) ;
#9570=CARTESIAN_POINT ( 'NONE',  ( 0.07405724077823318263, -1.001968503883243988, -0.1787899950787401604 ) ) ;
#9571=CARTESIAN_POINT ( 'NONE',  ( 2.892866454678787531E-17, -1.316929133858267820, 0.1574803149606299191 ) ) ;
#9585=CARTESIAN_POINT ( 'NONE',  ( 0.01929052294527547340, -0.05062618494071648156, -0.2742915362215330721 ) ) ;
#9588=CARTESIAN_POINT ( 'NONE',  ( 0.1264236179284866091, -0.2673483776780578580, -0.1264236179284866091 ) ) ;
#9589=CARTESIAN_POINT ( 'NONE',  ( -0.09380120751742244967, -0.09842519685039370636, 0.2089111925752385746 ) ) ;
#9590=CARTESIAN_POINT ( 'NONE',  ( -0.1574803149606300301, 0.009350393700787397108, -0.06523048226347956391 ) ) ;
#9598=CARTESIAN_POINT ( 'NONE',  ( -0.1264236179284866091, -0.9847440944344251212, 0.1264236179284866091 ) ) ;
#9599=CARTESIAN_POINT ( 'NONE',  ( 0.1787899950787401604, -1.164370078686393306, 0.07405724077823318263 ) ) ;
#9602=CARTESIAN_POINT ( 'NONE',  ( 0.1797182628040039365, -0.4537839670633606604, -2.200913952912460540E-17 ) ) ;
#9605=CARTESIAN_POINT ( 'NONE',  ( 0.1574803149606300301, -0.04970472440944883469, 0.06523048226347956391 ) ) ;
#9615=CARTESIAN_POINT ( 'NONE',  ( -0.1574803149606299191, -1.001968503829480328, 0.000000000000000000 ) ) ;
#9616=CARTESIAN_POINT ( 'NONE',  ( -0.1264236179284866091, -0.5615157479777322935, -0.1264236179284866091 ) ) ;
#9617=CARTESIAN_POINT ( 'NONE',  ( -0.1787899950787401882, -1.457185039316315045, 0.000000000000000000 ) ) ;
#9625=CARTESIAN_POINT ( 'NONE',  ( -0.1574803149606299191, -1.238188976270425012, 0.000000000000000000 ) ) ;
#9631=CARTESIAN_POINT ( 'NONE',  ( 0.2090839795229337272, -0.06563552548666866382, 0.1647146447861778384 ) ) ;
#9637=CARTESIAN_POINT ( 'NONE',  ( 0.2072130438524933116, -0.09851384797483406230, -0.0004152610389529299054 ) ) ;
#9642=CARTESIAN_POINT ( 'NONE',  ( 0.1264236179284866091, -1.537033417048135897, 0.1264236179284866091 ) ) ;
#9645=CARTESIAN_POINT ( 'NONE',  ( -1.094772975963752103E-17, -0.6008858267178898149, -0.1787899950787401882 ) ) ;
#9646=ADVANCED_FACE ( 'NONE', ( #757 ), #19693, .T. ) ;
#9651=CARTESIAN_POINT ( 'NONE',  ( -0.1787899950787401604, -0.3179133857730082058, 0.07405724077823318263 ) ) ;
#9652=CARTESIAN_POINT ( 'NONE',  ( -0.1787899950787401882, -0.7091535432533228045, 0.000000000000000000 ) ) ;
#9656=CARTESIAN_POINT ( 'NONE',  ( -0.07405724077823318263, 0.09436422074713922414, -0.1787899950787401604 ) ) ;
#9657=CARTESIAN_POINT ( 'NONE',  ( -0.07405724077823318263, 0.04133858273092887170, 0.1787899950787401604 ) ) ;
#9663=CARTESIAN_POINT ( 'NONE',  ( 0.1113553986120547346, -0.8789370078740158521, 0.1113553986120547346 ) ) ;
#9665=CARTESIAN_POINT ( 'NONE',  ( 3.301370929368692659E-17, -1.526618612732651314, 0.1797182628040039365 ) ) ;
#9667=CARTESIAN_POINT ( 'NONE',  ( -0.07405724077823318263, -0.4015748030958427028, -0.1787899950787401604 ) ) ;
#9669=CARTESIAN_POINT ( 'NONE',  ( 0.1292751490962095184, 0.09842519685039370636, -0.2107960287359162133 ) ) ;
#9676=CARTESIAN_POINT ( 'NONE',  ( 0.1787899950787401604, -0.1062992125446616531, 0.07405724077823318263 ) ) ;
#9677=CARTESIAN_POINT ( 'NONE',  ( 3.284318927891251994E-17, -0.06938976372576398377, 0.1787899950787401882 ) ) ;
#9679=CARTESIAN_POINT ( 'NONE',  ( -0.07405724077823318263, -0.9133858267178897039, -0.1787899950787401604 ) ) ;
#9686=CARTESIAN_POINT ( 'NONE',  ( -0.1264236179284866091, -1.339074803095842592, 0.1264236179284866091 ) ) ;
#9688=DIRECTION ( 'NONE',  ( 0.000000000000000000, 1.000000000000000000, 0.000000000000000000 ) ) ;
#9703=B_SPLINE_CURVE_WITH_KNOTS ( 'NONE', 3,
 ( #6155, #36120, #31362, #13152, #31825, #46412, #24620, #27786, #35876, #42347, #17660, #32058, #9543, #24388, #32309, #39220, #14075, #6632, #28228 ),
 .UNSPECIFIED., .F., .F.,
 ( 4, 1, 1, 1, 2, 2, 1, 1, 1, 1, 2, 2, 4 ),
 ( 0.000000000000000000, 0.1250000000000007494, 0.1875000000000011102, 0.2187500000000013045, 0.2343750000000013600, 0.2500000000000013878, 0.3750000000000005551, 0.4375000000000001110, 0.4687500000000000000, 0.4843749999999998890, 0.4921874999999998335, 0.4999999999999997780, 1.000000000000000000 ),
 .UNSPECIFIED. ) ;
#9706=CARTESIAN_POINT ( 'NONE',  ( -0.1787899950787401604, -1.155635779252861983, 0.07405724077823318263 ) ) ;
#9708=CARTESIAN_POINT ( 'NONE',  ( 0.07405724077823318263, -0.1309055117572600901, -0.1787899950787401604 ) ) ;
#9711=EDGE_LOOP ( 'NONE', ( #39011, #25189, #17501, #7564, #28436, #3615, #21717 ) ) ;
#9712=EDGE_CURVE ( 'NONE', #45034, #36603, #36082, .T. ) ;
#9716=CARTESIAN_POINT ( 'NONE',  ( 0.1787899950787401882, -0.7337598424659212970, -2.189545951927503898E-17 ) ) ;
#9719=CARTESIAN_POINT ( 'NONE',  ( -0.1797182628040039087, -1.184591053677534811, -0.07444174185955065859 ) ) ;
#9739=CARTESIAN_POINT ( 'NONE',  ( 4.681852760415787419E-17, -0.03219022224904102836, 0.2854330708661417804 ) ) ;
#9741=CARTESIAN_POINT ( 'NONE',  ( -0.1264236179284866091, 0.08316929139234625901, 0.1264236179284866091 ) ) ;
#9745=CARTESIAN_POINT ( 'NONE',  ( 0.1916154494608395820, 0.07733267719194271417, 0.1748038395390349997 ) ) ;
#9750=CARTESIAN_POINT ( 'NONE',  ( -0.1787899950787401882, -1.619586614119464585, 0.000000000000000000 ) ) ;
#9758=CARTESIAN_POINT ( 'NONE',  ( 0.1498865323622342038, 0.1262053965888239315, -0.06565210875279572922 ) ) ;
#9760=CARTESIAN_POINT ( 'NONE',  ( 0.1787899950787401882, -0.7053405036623090485, -2.189545951927503898E-17 ) ) ;
#9762=CARTESIAN_POINT ( 'NONE',  ( -0.02921664450966929283, -0.08956076947073877970, -0.1825412823646976601 ) ) ;
#9776=CARTESIAN_POINT ( 'NONE',  ( 0.1797182628040039087, -0.6481737308428884292, -0.07444174185955065859 ) ) ;
#9780=CARTESIAN_POINT ( 'NONE',  ( 0.1113553986120547346, -0.3671259842519685179, 0.1113553986120547346 ) ) ;
#9788=CARTESIAN_POINT ( 'NONE',  ( -0.1113553986120547346, -0.6033464565853857708, 0.1113553986120547346 ) ) ;
#9792=CARTESIAN_POINT ( 'NONE',  ( -0.1607166238174611572, -0.08956082419875868728, -0.06572622029918266662 ) ) ;
#9793=CARTESIAN_POINT ( 'NONE',  ( 0.1787899950787401604, -0.6525590550643474153, 0.07405724077823318263 ) ) ;
#9801=CARTESIAN_POINT ( 'NONE',  ( -0.07444174185955065859, 0.03096012742482846455, -0.1797182628040039087 ) ) ;
#9802=CARTESIAN_POINT ( 'NONE',  ( -0.1264236179284866091, -1.063484251914740275, 0.1264236179284866091 ) ) ;
#9803=CARTESIAN_POINT ( 'NONE',  ( 0.1574803149606299191, -1.385826771653543510, -1.928577636452523993E-17 ) ) ;
#9804=B_SPLINE_CURVE_WITH_KNOTS ( 'NONE', 3,
 ( #6048, #13964, #24987, #24289, #42930, #24749, #39583, #20674, #21140, #31957, #6762, #40460, #7644, #22259, #36894, #46776, #38884, #39344, #28614, #35316, #2455, #17081, #46311 ),
 .UNSPECIFIED., .F., .F.,
 ( 4, 2, 2, 1, 1, 1, 2, 2, 2, 1, 1, 2, 2, 4 ),
 ( 0.000000000000000000, 0.2500000000000052736, 0.3750000000000077161, 0.4375000000000087153, 0.4687500000000093814, 0.4843750000000096589, 0.4921875000000093814, 0.5000000000000091038, 0.6250000000000042188, 0.6875000000000016653, 0.7187500000000007772, 0.7343750000000004441, 0.7500000000000000000, 1.000000000000000000 ),
 .UNSPECIFIED. ) ;
#9820=CARTESIAN_POINT ( 'NONE',  ( -0.1588215770322243259, 0.09266989036297293425, -0.1937373906134662316 ) ) ;
#9825=CARTESIAN_POINT ( 'NONE',  ( 0.07405724077823318263, -0.2255176690166402764, -0.1787899950787401604 ) ) ;
#9826=CARTESIAN_POINT ( 'NONE',  ( -0.002278514610727500403, -0.09842519685039370636, 0.2245093560007807021 ) ) ;
#9827=CARTESIAN_POINT ( 'NONE',  ( 2.892866454678787531E-17, 0.02165354330708661734, 0.1574803149606299191 ) ) ;
#9831=CARTESIAN_POINT ( 'NONE',  ( 0.07405724077823318263, -1.272637795221826629, -0.1787899950787401604 ) ) ;
#9832=AXIS2_PLACEMENT_3D ( 'NONE', #8353, #37587, #11029 ) ;
#9834=CARTESIAN_POINT ( 'NONE',  ( -0.1797182628040039365, -0.5128390851735968869, 0.000000000000000000 ) ) ;
#9837=CARTESIAN_POINT ( 'NONE',  ( -0.1574803149606297803, 0.05364173228346464511, 0.06523048226347956391 ) ) ;
#9845=FACE_OUTER_BOUND ( 'NONE', #19297, .T. ) ;
#9847=CARTESIAN_POINT ( 'NONE',  ( -0.1787899950787401604, -0.5935039369541101895, 0.07405724077823318263 ) ) ;
#9848=CARTESIAN_POINT ( 'NONE',  ( -0.07405724077823318263, -1.371062992072219489, 0.1787899950787401604 ) ) ;
#9860=CARTESIAN_POINT ( 'NONE',  ( 0.1338895052746215397, -0.09842531827051598237, -0.1184899159207936509 ) ) ;
#9872=CARTESIAN_POINT ( 'NONE',  ( -0.2395769297574236179, -0.09851385218651377562, 0.02158642379462074462 ) ) ;
#9877=CARTESIAN_POINT ( 'NONE',  ( 0.1264236179284866091, -1.615773574528450940, 0.1264236179284866091 ) ) ;
#9879=CARTESIAN_POINT ( 'NONE',  ( 3.284318927891251994E-17, -0.5812007873478111097, 0.1787899950787401882 ) ) ;
#9881=ORIENTED_EDGE ( 'NONE', *, *, #33255, .F. ) ;
#9882=CARTESIAN_POINT ( 'NONE',  ( -0.1787899950787401604, -0.3228346456155278266, -0.07405724077823318263 ) ) ;
#9884=CARTESIAN_POINT ( 'NONE',  ( -0.2471922904502826812, -0.09842519685039372024, -0.006644306898575463166 ) ) ;
#9885=DIRECTION ( 'NONE',  ( 0.000000000000000000, 1.000000000000000000, 0.000000000000000000 ) ) ;
#9887=CARTESIAN_POINT ( 'NONE',  ( -1.094772975963752103E-17, -0.02620664539459307413, -0.1787899950787401882 ) ) ;
#9888=CARTESIAN_POINT ( 'NONE',  ( 0.07405724077823318263, 0.006889763833291078637, 0.1787899950787401604 ) ) ;
#9893=CARTESIAN_POINT ( 'NONE',  ( 0.1574803149606299191, -0.8346456692913386544, -1.928577636452523993E-17 ) ) ;
#9895=CARTESIAN_POINT ( 'NONE',  ( -1.100456976456230270E-17, -1.703783967063360105, -0.1797182628040039365 ) ) ;
#9897=CARTESIAN_POINT ( 'NONE',  ( -0.07405724077823318263, -0.3228346456155278266, -0.1787899950787401604 ) ) ;
#9902=ORIENTED_EDGE ( 'NONE', *, *, #2794, .F. ) ;
#9907=CARTESIAN_POINT ( 'NONE',  ( 0.1787899950787401604, -0.1801181101824570474, -0.07405724077823318263 ) ) ;
#9931=CARTESIAN_POINT ( 'NONE',  ( -0.1264236179284866091, 0.1077755906049446960, -0.1264236179284866091 ) ) ;
#9935=CARTESIAN_POINT ( 'NONE',  ( -0.2471922904502826812, 0.09842519685039370636, -0.006585516632646069672 ) ) ;
#9938=CARTESIAN_POINT ( 'NONE',  ( -0.1787899950787401604, -1.160557039095381437, -0.07405724077823318263 ) ) ;
#9940=CARTESIAN_POINT ( 'NONE',  ( -0.1264236179284866091, -0.08415354325332302654, -0.1264236179284866091 ) ) ;
#9941=ORIENTED_EDGE ( 'NONE', *, *, #19582, .F. ) ;
#9945=CARTESIAN_POINT ( 'NONE',  ( -0.1270800023317771588, -0.1929571954098172892, 0.1270800023317771588 ) ) ;
#9946=CARTESIAN_POINT ( 'NONE',  ( -0.1787899950787401604, -0.7559055117572593963, -0.07405724077823318263 ) ) ;
#9948=CARTESIAN_POINT ( 'NONE',  ( -0.1270800023317771588, -1.334689478874383717, 0.1270800023317771588 ) ) ;
#9957=DIRECTION ( 'NONE',  ( 0.000000000000000000, -0.8660254037844383745, 0.5000000000000003331 ) ) ;
#9975=CARTESIAN_POINT ( 'NONE',  ( -0.07405724077823318263, 0.03149606304588949135, -0.1787899950787401604 ) ) ;
#9979=CARTESIAN_POINT ( 'NONE',  ( 4.801428276353606495E-17, 0.03219022224904102836, 0.2854330708661417804 ) ) ;
#9983=CARTESIAN_POINT ( 'NONE',  ( -0.06523048226347956391, -0.4187992124908984093, -0.1574803149606300301 ) ) ;
#9984=CARTESIAN_POINT ( 'NONE',  ( -0.1264236179284866091, -1.654035433017102319, 0.1264236179284866091 ) ) ;
#9989=CARTESIAN_POINT ( 'NONE',  ( 2.700008691033534577E-17, 0.09842519685039370636, 0.2204724409448818867 ) ) ;
#9991=CARTESIAN_POINT ( 'NONE',  ( 0.1264236179284866091, -0.7102617635048287248, 0.1264236179284866091 ) ) ;
#9993=CARTESIAN_POINT ( 'NONE',  ( 0.09519241326698858752, -0.08956226547226790735, 0.1092664699140651619 ) ) ;
#10006=CARTESIAN_POINT ( 'NONE',  ( 0.1797182628040039087, -0.7318351481657215940, 0.07444174185955046430 ) ) ;
#10010=CARTESIAN_POINT ( 'NONE',  ( -0.1574803149606299191, -0.5787401574803149318, 0.000000000000000000 ) ) ;
#10011=CARTESIAN_POINT ( 'NONE',  ( -0.1574205454495407608, 0.1252972266898419451, -0.04195140859584962911 ) ) ;
#10021=EDGE_LOOP ( 'NONE', ( #45602, #31757, #42780, #40812 ) ) ;
#10024=EDGE_CURVE ( 'NONE', #4670, #36616, #7652, .T. ) ;
#10027=CARTESIAN_POINT ( 'NONE',  ( -1.100456976456230270E-17, 0.1466097337240411524, -0.1797182628040039365 ) ) ;
#10028=CARTESIAN_POINT ( 'NONE',  ( -0.1264236179284866091, -0.9847440944344251212, 0.1264236179284866091 ) ) ;
#10029=CARTESIAN_POINT ( 'NONE',  ( 0.1113553986120547346, -1.577755905511811108, -0.1113553986120547346 ) ) ;
#10033=ORIENTED_EDGE ( 'NONE', *, *, #35938, .F. ) ;
#10037=CARTESIAN_POINT ( 'NONE',  ( -9.642888182262618425E-18, -1.444881889656252083, -0.1574803149606299191 ) ) ;
#10045=CARTESIAN_POINT ( 'NONE',  ( -0.1674339218907005267, 0.08959396230939166428, -0.1887650509910711871 ) ) ;
#10048=CARTESIAN_POINT ( 'NONE',  ( 0.1787899950787401604, -0.3091790863394751065, -0.07405724077823318263 ) ) ;
#10049=CARTESIAN_POINT ( 'NONE',  ( -0.02050543330604039441, -0.09842519685039370636, 0.1561122773925366081 ) ) ;
#10053=( BOUNDED_CURVE ( )  B_SPLINE_CURVE ( 2, ( #45491, #41888, #19875, #16533, #13410, #1408, #5253, #27104, #20348 ),
 .UNSPECIFIED., .F., .T. ) 
 B_SPLINE_CURVE_WITH_KNOTS ( ( 3, 2, 2, 2, 3 ),
 ( 0.06500000000000000222, 0.06750000000000000444, 0.07000000000000000666, 0.07249999999999999500, 0.07499999999999999722 ),
 .UNSPECIFIED. ) 
 CURVE ( )  GEOMETRIC_REPRESENTATION_ITEM ( )  RATIONAL_B_SPLINE_CURVE ( ( 1.000000000000000000, 0.9238795325112869605, 1.000000000000000000, 0.9238795325112869605, 1.000000000000000000, 0.9238795325112869605, 1.000000000000000000, 0.9238795325112869605, 1.000000000000000000 ) ) 
 REPRESENTATION_ITEM ( '' )  ) ;
#10058=CARTESIAN_POINT ( 'NONE',  ( -0.1787899950787401604, -1.302165354276944242, -0.07405724077823318263 ) ) ;
#10060=CARTESIAN_POINT ( 'NONE',  ( -0.1270800023317771588, -0.4685477465909196892, 0.1270800023317771588 ) ) ;
#10063=CARTESIAN_POINT ( 'NONE',  ( 0.1574803149606300301, -0.2022637795275592509, -0.06523048226347956391 ) ) ;
#10070=CARTESIAN_POINT ( 'NONE',  ( -0.1574803149606300301, -0.06938976377952764396, -0.06523048226347956391 ) ) ;
#10081=CARTESIAN_POINT ( 'NONE',  ( -0.1787899950787401604, -0.6328740156942683770, 0.07405724077823318263 ) ) ;
#10082=CARTESIAN_POINT ( 'NONE',  ( -0.07405724077823318263, -1.425196850339937482, -0.1787899950787401604 ) ) ;
#10090=CARTESIAN_POINT ( 'NONE',  ( 0.09110444530572323063, -0.09842520415008684798, -0.1538371768615053592 ) ) ;
#10098=CARTESIAN_POINT ( 'NONE',  ( -0.06523048226347956391, -0.1284448817822367028, 0.1574803149606297803 ) ) ;
#10103=CARTESIAN_POINT ( 'NONE',  ( 0.1762355013749781762, -0.09851384352596320726, -0.09845540268461337730 ) ) ;
#10108=ORIENTED_EDGE ( 'NONE', *, *, #41904, .T. ) ;
#10109=CARTESIAN_POINT ( 'NONE',  ( 0.1264236179284866091, -1.684671212323726630, -0.1264236179284866091 ) ) ;
#10111=CARTESIAN_POINT ( 'NONE',  ( -0.1264236179284866091, -0.5861220471903307860, 0.1264236179284866091 ) ) ;
#10115=CARTESIAN_POINT ( 'NONE',  ( 0.1264236179284866091, -0.3449803149068665364, 0.1264236179284866091 ) ) ;
#10116=CARTESIAN_POINT ( 'NONE',  ( -1.094772975963752103E-17, -0.7189960629383621571, -0.1787899950787401882 ) ) ;
#10123=CARTESIAN_POINT ( 'NONE',  ( -0.1787899950787401604, -0.01882475563081354580, -0.07405724077823318263 ) ) ;
#10131=CARTESIAN_POINT ( 'NONE',  ( 2.892866454678787531E-17, -0.8838582677165355284, 0.1574803149606299191 ) ) ;
#10133=CARTESIAN_POINT ( 'NONE',  ( -0.1270800023317771588, -1.738232785960998061, -0.1270800023317771588 ) ) ;
#10143=CARTESIAN_POINT ( 'NONE',  ( 0.1787899950787401604, -0.06200787396198446239, -0.07405724077823318263 ) ) ;
#10145=CARTESIAN_POINT ( 'NONE',  ( 3.284318927891251994E-17, -0.8567913385289133155, 0.1787899950787401882 ) ) ;
#10165=CARTESIAN_POINT ( 'NONE',  ( -0.1787899950787401882, 0.03395669296714932950, 0.000000000000000000 ) ) ;
#10169=CARTESIAN_POINT ( 'NONE',  ( 0.1787899950787401604, -1.474409448765133801, -0.07405724077823318263 ) ) ;
#10174=CARTESIAN_POINT ( 'NONE',  ( 0.1787899950787401882, -1.256521606024513904, -2.189545951927503898E-17 ) ) ;
#10176=CARTESIAN_POINT ( 'NONE',  ( -0.07405724077823318263, -0.1112204723871813017, 0.1787899950787401604 ) ) ;
#10184=CARTESIAN_POINT ( 'NONE',  ( -0.07405724077823318263, -1.415354330654897019, 0.1787899950787401604 ) ) ;
#10185=CARTESIAN_POINT ( 'NONE',  ( -1.094772975963752103E-17, -0.7632874015210393548, -0.1787899950787401882 ) ) ;
#10188=CARTESIAN_POINT ( 'NONE',  ( 0.07444174185955046430, -1.273173730842887208, -0.1797182628040039087 ) ) ;
#10197=CARTESIAN_POINT ( 'NONE',  ( 0.07405724077823318263, 0.02657480320336980464, -0.1787899950787401604 ) ) ;
#10214=CARTESIAN_POINT ( 'NONE',  ( 0.07405724077823318263, 0.05118110241596821736, 0.1787899950787401604 ) ) ;
#10218=CARTESIAN_POINT ( 'NONE',  ( 0.1235961452251413406, 0.09842519685039370636, 0.2140748031496062798 ) ) ;
#10223=CARTESIAN_POINT ( 'NONE',  ( 0.07405724077823318263, -1.710629921206078041, -0.1787899950787401604 ) ) ;
#10231=CARTESIAN_POINT ( 'NONE',  ( -1.094772975963752103E-17, -0.7348680627174272173, -0.1787899950787401882 ) ) ;
#10234=CARTESIAN_POINT ( 'NONE',  ( 2.892866454678787531E-17, -0.08661417312081949593, 0.1574803149606299191 ) ) ;
#10240=CARTESIAN_POINT ( 'NONE',  ( 0.1574803149606300301, 0.06840551181102358380, 0.06523048226347956391 ) ) ;
#10250=CARTESIAN_POINT ( 'NONE',  ( -0.1797182628040039087, -0.8253390851735974421, 0.07444174185955065859 ) ) ;
#10254=CARTESIAN_POINT ( 'NONE',  ( 2.892866454678787531E-17, -0.5295275590551181688, 0.1574803149606299191 ) ) ;
#10255=CARTESIAN_POINT ( 'NONE',  ( -0.03350953465935899850, 0.1209034135645020575, -0.1556370229766415314 ) ) ;
#10271=CARTESIAN_POINT ( 'NONE',  ( -0.1797182628040039365, 0.1564522534090805050, 0.000000000000000000 ) ) ;
#10272=CARTESIAN_POINT ( 'NONE',  ( 0.1264236179284866091, -1.053641732229700700, 0.1264236179284866091 ) ) ;
#10273=CARTESIAN_POINT ( 'NONE',  ( 0.1113553986120547346, -1.459645669291338432, -0.1113553986120547346 ) ) ;
#10281=CARTESIAN_POINT ( 'NONE',  ( -0.1574803149606297803, -1.432578740049952781, 0.06523048226347956391 ) ) ;
#10288=CARTESIAN_POINT ( 'NONE',  ( -0.2471922904502825702, 0.07695608958885592765, 0.07926021241888449309 ) ) ;
#10293=CARTESIAN_POINT ( 'NONE',  ( -1.094772975963752103E-17, -0.2230570390953807158, -0.1787899950787401882 ) ) ;
#10303=CARTESIAN_POINT ( 'NONE',  ( -0.1264236179284866091, -1.152066929080094448, -0.1264236179284866091 ) ) ;
#10304=CARTESIAN_POINT ( 'NONE',  ( -0.1787899950787401882, -1.457185039316315045, 0.000000000000000000 ) ) ;
#10309=CARTESIAN_POINT ( 'NONE',  ( 0.1113553986120547346, -0.08169291338582677919, -0.1113553986120547346 ) ) ;
#10316=CARTESIAN_POINT ( 'NONE',  ( -0.06523048226347956391, -0.05954724409448820810, 0.1574803149606297803 ) ) ;
#10323=CARTESIAN_POINT ( 'NONE',  ( -9.642888182262618425E-18, -1.523622047136566682, -0.1574803149606299191 ) ) ;
#10324=CARTESIAN_POINT ( 'NONE',  ( 0.1787899950787401882, -0.6156496062454488438, -2.189545951927503898E-17 ) ) ;
#10325=CARTESIAN_POINT ( 'NONE',  ( 0.1113553986120547346, -1.065944881889763662, -0.1113553986120547346 ) ) ;
#10343=CARTESIAN_POINT ( 'NONE',  ( 0.06523048226347956391, -0.2268700786326303398, -0.1574803149606300301 ) ) ;
#10348=CARTESIAN_POINT ( 'NONE',  ( -0.05992402829640944978, -0.09851383910125414978, -0.1770211755185344404 ) ) ;
#10354=CARTESIAN_POINT ( 'NONE',  ( 0.07405724077823318263, -1.736344440670183120, 0.1787899950787401604 ) ) ;
#10356=CARTESIAN_POINT ( 'NONE',  ( 0.1787899950787401882, -0.6894685038832439883, -2.189545951927503898E-17 ) ) ;
#10361=CARTESIAN_POINT ( 'NONE',  ( -0.1264236179284866091, -0.3252952755367877757, -0.1264236179284866091 ) ) ;
#10362=CARTESIAN_POINT ( 'NONE',  ( -0.1264236179284866091, -0.8321850393163149340, -0.1264236179284866091 ) ) ;
#10368=CARTESIAN_POINT ( 'NONE',  ( -0.07405724077823318263, -0.06311609421349069493, -0.1787899950787401604 ) ) ;
#10374=CARTESIAN_POINT ( 'NONE',  ( 3.301370929368692659E-17, -1.802209163913756296, 0.1797182628040039365 ) ) ;
#10382=VERTEX_POINT ( 'NONE', #46431 ) ;
#10385=CARTESIAN_POINT ( 'NONE',  ( 3.284318927891251994E-17, -0.1924212597887563214, 0.1787899950787401882 ) ) ;
#10387=ADVANCED_FACE ( 'NONE', ( #13399 ), #46667, .F. ) ;
#10388=CARTESIAN_POINT ( 'NONE',  ( 0.1264236179284866091, -1.009350393647023614, 0.1264236179284866091 ) ) ;
#10409=CARTESIAN_POINT ( 'NONE',  ( 0.07405724077823318263, 0.006889763833291078637, 0.1787899950787401604 ) ) ;
#10418=CARTESIAN_POINT ( 'NONE',  ( 0.07405724077823318263, -1.367249952481208064, -0.1787899950787401604 ) ) ;
#10420=CARTESIAN_POINT ( 'NONE',  ( 0.07405724077823318263, -0.2244094487651340231, 0.1787899950787401604 ) ) ;
#10427=CARTESIAN_POINT ( 'NONE',  ( -0.07405724077823318263, -1.548228346402928723, -0.1787899950787401604 ) ) ;
#10428=CARTESIAN_POINT ( 'NONE',  ( -0.1787899950787401604, -0.7952755904974174728, -0.07405724077823318263 ) ) ;
#10430=CARTESIAN_POINT ( 'NONE',  ( -0.1270800023317771588, -1.305161919819265659, -0.1270800023317771588 ) ) ;
#10438=CARTESIAN_POINT ( 'NONE',  ( -0.1574803149606300301, -0.7682086613097959260, -0.06523048226347956391 ) ) ;
#10440=CARTESIAN_POINT ( 'NONE',  ( -0.1264236179284866091, 0.03395669296714932950, -0.1264236179284866091 ) ) ;
#10455=CARTESIAN_POINT ( 'NONE',  ( -0.1264236179284866091, -0.005413385773008149403, -0.1264236179284866091 ) ) ;
#10467=CARTESIAN_POINT ( 'NONE',  ( -0.1264236179284866091, -1.781988188922614347, -0.1264236179284866091 ) ) ;
#10476=CARTESIAN_POINT ( 'NONE',  ( 0.1787899950787401604, -0.7865412910638841515, 0.07405724077823318263 ) ) ;
#10477=ORIENTED_EDGE ( 'NONE', *, *, #35036, .F. ) ;
#10491=CARTESIAN_POINT ( 'NONE',  ( 0.1797182628040039087, -0.8056540458035184038, -0.07444174185955065859 ) ) ;
#10495=CARTESIAN_POINT ( 'NONE',  ( -0.1113553986120547346, -0.5836614173228346081, -0.1113553986120547346 ) ) ;
#10496=CARTESIAN_POINT ( 'NONE',  ( -0.1527835536277865613, 0.1279265601668728991, 0.06534438871128525617 ) ) ;
#10506=CARTESIAN_POINT ( 'NONE',  ( -0.1787899950787401882, -0.6697834645131652831, 0.000000000000000000 ) ) ;
#10514=CARTESIAN_POINT ( 'NONE',  ( 0.07444174185955065859, 0.05064516679490722179, 0.1797182628040039087 ) ) ;
#10515=CARTESIAN_POINT ( 'NONE',  ( 0.07405724077823318263, -1.174212598371433769, 0.1787899950787401604 ) ) ;
#10516=CARTESIAN_POINT ( 'NONE',  ( 0.1574803149606300301, -1.545767716535432879, 0.06523048226347956391 ) ) ;
#10531=CARTESIAN_POINT ( 'NONE',  ( 0.08774906724789779955, -0.09246610911303654312, -0.2347711071351356593 ) ) ;
#10534=CARTESIAN_POINT ( 'NONE',  ( 0.1264236179284866091, -0.3953011335835693307, 0.1264236179284866091 ) ) ;
#10543=CARTESIAN_POINT ( 'NONE',  ( 0.1264236179284866091, -1.240649606245448622, -0.1264236179284866091 ) ) ;
#10544=CARTESIAN_POINT ( 'NONE',  ( -0.1264236179284866091, -1.304625984198204636, -0.1264236179284866091 ) ) ;
#10546=( NAMED_UNIT ( * ) SI_UNIT ( $, .STERADIAN. ) SOLID_ANGLE_UNIT ( ) ) ;
#10552=CARTESIAN_POINT ( 'NONE',  ( -0.1574803149606297803, -0.1038385826771653780, 0.06523048226347956391 ) ) ;
#10563=CARTESIAN_POINT ( 'NONE',  ( -0.1264236179284866091, -0.03494094482812625663, 0.1264236179284866091 ) ) ;
#10567=CARTESIAN_POINT ( 'NONE',  ( 0.1574803149606300301, -1.496555118002708795, 0.06523048226347956391 ) ) ;
#10568=CARTESIAN_POINT ( 'NONE',  ( -0.1787899950787401604, -0.5984251967966303098, -0.07405724077823318263 ) ) ;
#10569=CARTESIAN_POINT ( 'NONE',  ( 0.1113553986120547346, -1.036417322834645827, 0.1113553986120547346 ) ) ;
#10579=EDGE_LOOP ( 'NONE', ( #8735, #5384, #25391, #35500, #31388, #43849, #20696 ) ) ;
#10590=CARTESIAN_POINT ( 'NONE',  ( -0.1574803149606297803, -0.2121062991050713942, 0.06523048226347956391 ) ) ;
#10595=CARTESIAN_POINT ( 'NONE',  ( -0.02491398756834440828, -0.09851384158024625859, -0.1871469785078783421 ) ) ;
#10599=CARTESIAN_POINT ( 'NONE',  ( -1.094772975963752103E-17, -1.679749952481206954, -0.1787899950787401882 ) ) ;
#10605=CARTESIAN_POINT ( 'NONE',  ( -0.1787899950787401882, -0.9847440944344251212, 0.000000000000000000 ) ) ;
#10608=CARTESIAN_POINT ( 'NONE',  ( -0.1787899950787401604, -0.1369349918512859643, -0.07405724077823318263 ) ) ;
#10609=CARTESIAN_POINT ( 'NONE',  ( 0.1264236179284866091, 0.009350393754550925460, 0.1264236179284866091 ) ) ;
#10616=CARTESIAN_POINT ( 'NONE',  ( -0.1797182628040039365, -1.733311526118478385, 0.000000000000000000 ) ) ;
#10619=CARTESIAN_POINT ( 'NONE',  ( -0.1478661631957976508, -0.09575019180979005284, 0.2000608872904859059 ) ) ;
#10624=CARTESIAN_POINT ( 'NONE',  ( 0.1787899950787401604, -0.1407480314422995815, -0.07405724077823318263 ) ) ;
#10626=CARTESIAN_POINT ( 'NONE',  ( 3.284318927891251994E-17, -1.053641732229700700, 0.1787899950787401882 ) ) ;
#10635=LINE ( 'NONE', #39827, #23210 ) ;
#10645=CARTESIAN_POINT ( 'NONE',  ( 0.1787899950787401604, -0.02263779522182706588, -0.07405724077823318263 ) ) ;
#10652=CARTESIAN_POINT ( 'NONE',  ( -0.1787899950787401604, -1.278667275315853002, -0.07405724077823318263 ) ) ;
#10654=CARTESIAN_POINT ( 'NONE',  ( -0.1264236179284866091, -0.2022637794737956740, -0.1264236179284866091 ) ) ;
#10663=CARTESIAN_POINT ( 'NONE',  ( 0.07405724077823318263, -1.592519684985606254, -0.1787899950787401604 ) ) ;
#10664=CARTESIAN_POINT ( 'NONE',  ( -0.1787899950787401882, -0.7140748030958424808, 0.000000000000000000 ) ) ;
#10674=CARTESIAN_POINT ( 'NONE',  ( -0.1026092249587055166, 0.1299212598425196763, 0.1321676130798911386 ) ) ;
#10677=CARTESIAN_POINT ( 'NONE',  ( 0.1574803149606299191, -0.7854330707586142379, -1.928577636452523993E-17 ) ) ;
#10698=CARTESIAN_POINT ( 'NONE',  ( 0.1264236179284866091, -0.05462598419820496182, -0.1264236179284866091 ) ) ;
#10704=CARTESIAN_POINT ( 'NONE',  ( 0.1572356565281126384, -0.09317336072454235341, -0.1946530291195974205 ) ) ;
#10709=CARTESIAN_POINT ( 'NONE',  ( 2.892866454678787531E-17, 0.1102362205799679168, 0.1574803149606299191 ) ) ;
#10717=CARTESIAN_POINT ( 'NONE',  ( 0.1264236179284866091, -0.8677420784654585884, 0.1264236179284866091 ) ) ;
#10735=CARTESIAN_POINT ( 'NONE',  ( -0.1270800023317771588, -0.8622485339924941261, 0.1270800023317771588 ) ) ;
#10740=CARTESIAN_POINT ( 'NONE',  ( 0.06523048226347956391, -0.5123031496062991907, -0.1574803149606300301 ) ) ;
#10742=CARTESIAN_POINT ( 'NONE',  ( -0.1157464095645248381, 0.1295232178076358986, 0.1214645533880106126 ) ) ;
#10753=CARTESIAN_POINT ( 'NONE',  ( 3.284318927891251994E-17, -0.6205708660879685201, 0.1787899950787401882 ) ) ;
#10754=CYLINDRICAL_SURFACE ( 'NONE', #10870, 0.2204724409448818867 ) ;
#10759=CARTESIAN_POINT ( 'NONE',  ( 3.284318927891251994E-17, -1.176673228292692830, 0.1787899950787401882 ) ) ;
#10760=CARTESIAN_POINT ( 'NONE',  ( -0.1574803149606299191, -1.562992125984252079, 0.000000000000000000 ) ) ;
#10766=ORIENTED_EDGE ( 'NONE', *, *, #26845, .T. ) ;
#10775=CARTESIAN_POINT ( 'NONE',  ( 0.1787899950787401604, -0.4715806611426248129, 0.07405724077823318263 ) ) ;
#10776=CARTESIAN_POINT ( 'NONE',  ( -0.01524090226806027598, -0.09842519685039370636, 0.1563540702671338822 ) ) ;
#10786=CARTESIAN_POINT ( 'NONE',  ( 0.07405724077823318263, -1.134842519631275914, 0.1787899950787401604 ) ) ;
#10787=CARTESIAN_POINT ( 'NONE',  ( 0.07405724077823318263, -1.405511810969858999, 0.1787899950787401604 ) ) ;
#10791=CARTESIAN_POINT ( 'NONE',  ( 0.07444174185955065859, -0.6186461717877695943, 0.1797182628040039087 ) ) ;
#10795=CARTESIAN_POINT ( 'NONE',  ( -0.1113553986120547346, -0.1801181102362204856, 0.1113553986120547346 ) ) ;
#10800=CYLINDRICAL_SURFACE ( 'NONE', #24101, 0.1574803149606299191 ) ;
#10808=CARTESIAN_POINT ( 'NONE',  ( 0.06523048226347956391, -1.501476377845230248, 0.1574803149606297803 ) ) ;
#10809=CARTESIAN_POINT ( 'NONE',  ( -0.1264236179284866091, -0.7485236219934803259, 0.1264236179284866091 ) ) ;
#10812=CARTESIAN_POINT ( 'NONE',  ( 0.1574803149606300301, -1.033956692913387210, 0.06523048226347956391 ) ) ;
#10819=CARTESIAN_POINT ( 'NONE',  ( 0.06523048226347956391, -1.289862204616882169, -0.1574803149606300301 ) ) ;
#10825=CARTESIAN_POINT ( 'NONE',  ( 0.1113553986120547346, -0.2785433069790869687, 0.1113553986120547346 ) ) ;
#10835=DIRECTION ( 'NONE',  ( 1.000000000000000000, 0.000000000000000000, 0.000000000000000000 ) ) ;
#10843=CARTESIAN_POINT ( 'NONE',  ( 0.1264236179284866091, -0.8813976377415118080, -0.1264236179284866091 ) ) ;
#10848=CARTESIAN_POINT ( 'NONE',  ( -0.1797182628040039087, -0.1609690064334393378, -0.07444174185955065859 ) ) ;
#10850=CARTESIAN_POINT ( 'NONE',  ( -0.07405724077823318263, -0.1664625509064040221, 0.1787899950787401604 ) ) ;
#10851=CARTESIAN_POINT ( 'NONE',  ( 0.1787899950787401882, -0.2563976377415121966, -2.189545951927503898E-17 ) ) ;
#10852=CARTESIAN_POINT ( 'NONE',  ( -0.1787899950787401604, -0.007874015694267972806, -0.07405724077823318263 ) ) ;
#10858=CARTESIAN_POINT ( 'NONE',  ( -0.1797182628040039087, -1.691480817457061914, 0.07444174185955065859 ) ) ;
#10860=FACE_OUTER_BOUND ( 'NONE', #8592, .T. ) ;
#10864=CARTESIAN_POINT ( 'NONE',  ( -0.1787899950787401604, -0.3228346456155278266, -0.07405724077823318263 ) ) ;
#10867=CARTESIAN_POINT ( 'NONE',  ( 0.1787899950787401604, -1.080708661363559919, -0.07405724077823318263 ) ) ;
#10870=AXIS2_PLACEMENT_3D ( 'NONE', #3766, #39697, #6881 ) ;
#10888=CARTESIAN_POINT ( 'NONE',  ( -0.1787899950787401604, -0.08169291333206318839, 0.07405724077823318263 ) ) ;
#10894=CARTESIAN_POINT ( 'NONE',  ( -0.1264236179284866091, -1.231915306811915523, 0.1264236179284866091 ) ) ;
#10896=CARTESIAN_POINT ( 'NONE',  ( -0.1264236179284866091, -0.3105314960092286913, 0.1264236179284866091 ) ) ;
#10902=CARTESIAN_POINT ( 'NONE',  ( -0.2471922904502827645, -0.09842519685039372024, 0.01321092903694667461 ) ) ;
#10908=CARTESIAN_POINT ( 'NONE',  ( 0.07405724077823318263, -1.671259842465922407, -0.1787899950787401604 ) ) ;
#10918=CARTESIAN_POINT ( 'NONE',  ( 0.1113553986120547346, -0.7805118109160945616, -0.1113553986120547346 ) ) ;
#10935=CARTESIAN_POINT ( 'NONE',  ( -0.1787899950787401604, -0.07677165348954355373, 0.07405724077823318263 ) ) ;
#10941=CARTESIAN_POINT ( 'NONE',  ( -0.1121631700669266513, 0.09842519685039372024, 0.2206756344348398957 ) ) ;
#10945=CARTESIAN_POINT ( 'NONE',  ( -0.06523048226347956391, 0.06840551191855072377, 0.1574803149606297803 ) ) ;
#10951=CARTESIAN_POINT ( 'NONE',  ( 0.07405724077823318263, -0.8308326296465612382, 0.1787899950787401604 ) ) ;
#10954=CARTESIAN_POINT ( 'NONE',  ( -0.09235291751817698014, -0.08956172857085197003, 0.1299824129084523605 ) ) ;
#10958=CARTESIAN_POINT ( 'NONE',  ( 0.000000000000000000, -0.09842519685039370636, 0.000000000000000000 ) ) ;
#10967=CARTESIAN_POINT ( 'NONE',  ( -0.1797182628040039365, -0.8671697938350138024, 0.000000000000000000 ) ) ;
#10983=CARTESIAN_POINT ( 'NONE',  ( 0.1787899950787401604, -0.8100393700249772788, 0.07405724077823318263 ) ) ;
#10985=LINE ( 'NONE', #43305, #13074 ) ;
#10989=CARTESIAN_POINT ( 'NONE',  ( 0.1113553986120547346, -1.508858267716535417, 0.1113553986120547346 ) ) ;
#10994=CARTESIAN_POINT ( 'NONE',  ( 0.1113553986120547346, 0.1053149606299212532, 0.1113553986120547346 ) ) ;
#11004=CARTESIAN_POINT ( 'NONE',  ( 0.07405724077823318263, -0.4371318422449868013, 0.1787899950787401604 ) ) ;
#11005=CARTESIAN_POINT ( 'NONE',  ( -0.1516314384195220633, -0.09842519685039370636, -0.09561409171430847176 ) ) ;
#11009=CARTESIAN_POINT ( 'NONE',  ( 0.2471902767489403685, -0.09658829859166323528, 0.02317992046427707481 ) ) ;
#11014=CARTESIAN_POINT ( 'NONE',  ( 0.1787899950787401604, -1.248031496009228913, 0.07405724077823318263 ) ) ;
#11015=CARTESIAN_POINT ( 'NONE',  ( 0.07405724077823318263, -1.326771653489542402, 0.1787899950787401604 ) ) ;
#11019=CARTESIAN_POINT ( 'NONE',  ( -0.1797182628040039087, -0.6334099513153290673, -0.07444174185955065859 ) ) ;
#11022=CARTESIAN_POINT ( 'NONE',  ( 0.06523048226347956391, -0.1727362204724408601, 0.1574803149606297803 ) ) ;
#11026=CARTESIAN_POINT ( 'NONE',  ( -0.1264236179284866091, -0.1973425196312759700, 0.1264236179284866091 ) ) ;
#11029=DIRECTION ( 'NONE',  ( 0.000000000000000000, 0.000000000000000000, 1.000000000000000000 ) ) ;
#11039=CARTESIAN_POINT ( 'NONE',  ( 0.1787899950787401882, -1.555610236166708571, -2.189545951927503898E-17 ) ) ;
#11040=CARTESIAN_POINT ( 'NONE',  ( -0.1574803149606297803, -1.550688976270427011, 0.06523048226347956391 ) ) ;
#11041=CARTESIAN_POINT ( 'NONE',  ( -0.07405724077823318263, -0.7608267715997808489, -0.1787899950787401604 ) ) ;
#11043=CARTESIAN_POINT ( 'NONE',  ( -9.642888182262618425E-18, -1.021653543307086576, -0.1574803149606299191 ) ) ;
#11070=CARTESIAN_POINT ( 'NONE',  ( -0.1264236179284866091, -0.6747047243556849594, -0.1264236179284866091 ) ) ;
#11076=CARTESIAN_POINT ( 'NONE',  ( -0.07405724077823318263, -0.8740157479777336258, -0.1787899950787401604 ) ) ;
#11080=CARTESIAN_POINT ( 'NONE',  ( 0.1797182628040039087, -0.1757327859609983112, -0.07444174185955065859 ) ) ;
#11081=CARTESIAN_POINT ( 'NONE',  ( 0.1787899950787401882, -0.1541594013001049146, -2.189545951927503898E-17 ) ) ;
#11082=CARTESIAN_POINT ( 'NONE',  ( 0.1787899950787401882, -0.1038385826234017734, -2.189545951927503898E-17 ) ) ;
#11083=CARTESIAN_POINT ( 'NONE',  ( 0.2471922904502826812, -0.09842519685039370636, -5.914624404477007554E-17 ) ) ;
#11091=CARTESIAN_POINT ( 'NONE',  ( -0.1888229765468985855, -0.07899262986810677567, 0.1764160547656800637 ) ) ;
#11093=CARTESIAN_POINT ( 'NONE',  ( -9.642888182262618425E-18, -0.9330708660342048599, -0.1574803149606299191 ) ) ;
#11094=CARTESIAN_POINT ( 'NONE',  ( -1.094772975963752103E-17, -0.2514763778989925203, -0.1787899950787401882 ) ) ;
#11097=CARTESIAN_POINT ( 'NONE',  ( -0.07405724077823318263, -1.134842519631275914, 0.1787899950787401604 ) ) ;
#11106=AXIS2_PLACEMENT_3D ( 'NONE', #47428, #38287, #27302 ) ;
#11119=CARTESIAN_POINT ( 'NONE',  ( -0.1787899950787401882, 0.07332677170730689253, 0.000000000000000000 ) ) ;
#11127=CARTESIAN_POINT ( 'NONE',  ( 0.07405724077823318263, -1.263903495788293307, 0.1787899950787401604 ) ) ;
#11129=CARTESIAN_POINT ( 'NONE',  ( 0.07405724077823318263, -0.2096456692375751329, -0.1787899950787401604 ) ) ;
#11133=CARTESIAN_POINT ( 'NONE',  ( -0.2471904733176818747, -0.07069887449061568185, 0.09042980707098648152 ) ) ;
#11138=CARTESIAN_POINT ( 'NONE',  ( 0.07405724077823318263, -1.681102362150960650, 0.1787899950787401604 ) ) ;
#11141=CARTESIAN_POINT ( 'NONE',  ( -0.07444174185955065859, -1.489709163913754075, 0.1797182628040039087 ) ) ;
#11171=CARTESIAN_POINT ( 'NONE',  ( 0.1264236179284866091, -0.2219488188438744347, 0.1264236179284866091 ) ) ;
#11181=CARTESIAN_POINT ( 'NONE',  ( -0.07405724077823318263, -1.809055118056471123, 0.1787899950787401604 ) ) ;
#11191=CARTESIAN_POINT ( 'NONE',  ( -0.07405724077823318263, -0.8111475902764821999, -0.1787899950787401604 ) ) ;
#11199=CARTESIAN_POINT ( 'NONE',  ( -0.1787899950787401882, -0.4778543306548976854, 0.000000000000000000 ) ) ;
#11201=CARTESIAN_POINT ( 'NONE',  ( 0.1270800023317771588, -0.9213036521027303527, -0.1270800023317771588 ) ) ;
#11211=CARTESIAN_POINT ( 'NONE',  ( -0.1113553986120547346, -0.6525590550105826448, -0.1113553986120547346 ) ) ;
#11214=CARTESIAN_POINT ( 'NONE',  ( -0.07405724077823318263, -0.8346456692375755493, -0.1787899950787401604 ) ) ;
#11219=CARTESIAN_POINT ( 'NONE',  ( -0.1574803149606299191, -1.641732283464567121, 0.000000000000000000 ) ) ;
#11227=CARTESIAN_POINT ( 'NONE',  ( -0.1574803149606299191, -0.2933070865066460531, 0.000000000000000000 ) ) ;
#11228=CARTESIAN_POINT ( 'NONE',  ( 0.1787899950787401882, -1.442421259788756016, -2.189545951927503898E-17 ) ) ;
#11235=CARTESIAN_POINT ( 'NONE',  ( 0.05473164110560585494, 0.07681961335491396814, -0.2538337431406301747 ) ) ;
#11237=CARTESIAN_POINT ( 'NONE',  ( -0.1787899950787401604, -0.4076042831898689656, 0.07405724077823318263 ) ) ;
#11238=CARTESIAN_POINT ( 'NONE',  ( -0.1791659572252606303, -0.08955948998496260360, -0.1686289933158019450 ) ) ;
#11247=CARTESIAN_POINT ( 'NONE',  ( 0.1787899950787401882, -1.403051181048598384, -2.189545951927503898E-17 ) ) ;
#11249=CARTESIAN_POINT ( 'NONE',  ( 0.1264236179284866091, -1.442421259788756016, 0.1264236179284866091 ) ) ;
#11252=CARTESIAN_POINT ( 'NONE',  ( 0.1797182628040039365, -0.6112642820239901909, -2.200913952912460540E-17 ) ) ;
#11256=CARTESIAN_POINT ( 'NONE',  ( -9.642888182262618425E-18, -0.2342519685039370358, -0.1574803149606299191 ) ) ;
#11259=CARTESIAN_POINT ( 'NONE',  ( -0.07405724077823318263, -0.1948818897100161873, 0.1787899950787401604 ) ) ;
#11270=CARTESIAN_POINT ( 'NONE',  ( 0.07405724077823318263, -1.602362204670647161, 0.1787899950787401604 ) ) ;
#11271=CARTESIAN_POINT ( 'NONE',  ( -0.1574803149606300301, -1.516240157372787944, -0.06523048226347956391 ) ) ;
#11272=CARTESIAN_POINT ( 'NONE',  ( -9.642888182262618425E-18, -1.139763779527559029, -0.1574803149606299191 ) ) ;
#11283=CARTESIAN_POINT ( 'NONE',  ( 0.1113553986120547346, -1.341535432963338437, 0.1113553986120547346 ) ) ;
#11289=CARTESIAN_POINT ( 'NONE',  ( 0.05769625742918475797, 0.07859832706092276244, 0.2521221211081680624 ) ) ;
#11300=CARTESIAN_POINT ( 'NONE',  ( -0.1787899950787401604, -0.6722440944344262315, -0.07405724077823318263 ) ) ;
#11302=CARTESIAN_POINT ( 'NONE',  ( -0.07405724077823318263, -0.9429133857730090940, 0.1787899950787401604 ) ) ;
#11304=CARTESIAN_POINT ( 'NONE',  ( -0.1264236179284866091, -0.4434055117572598959, -0.1264236179284866091 ) ) ;
#11305=CARTESIAN_POINT ( 'NONE',  ( 0.1787899950787401882, -0.9650590550643465271, -2.189545951927503898E-17 ) ) ;
#11308=CARTESIAN_POINT ( 'NONE',  ( 0.1270800023317771588, -0.1437445969846202765, 0.1270800023317771588 ) ) ;
#11309=CARTESIAN_POINT ( 'NONE',  ( -0.1574803149606300301, 0.1668307086614173873, -0.06523048226347956391 ) ) ;
#11310=CARTESIAN_POINT ( 'NONE',  ( 0.1264236179284866091, -0.1087598424659214497, 0.1264236179284866091 ) ) ;
#11311=CARTESIAN_POINT ( 'NONE',  ( 0.2471922763370229259, -0.09254788073173002283, -0.04110581524678511012 ) ) ;
#11326=CARTESIAN_POINT ( 'NONE',  ( 0.1264236179284866091, -0.3056102361667090705, 0.1264236179284866091 ) ) ;
#11328=CARTESIAN_POINT ( 'NONE',  ( -0.1264236179284866091, -1.147145669237574772, -0.1264236179284866091 ) ) ;
#11356=CARTESIAN_POINT ( 'NONE',  ( 0.07405724077823318263, -1.524730267441837483, -0.1787899950787401604 ) ) ;
#11358=CARTESIAN_POINT ( 'NONE',  ( 0.07405724077823318263, -0.3277559054580475584, -0.1787899950787401604 ) ) ;
#11366=CARTESIAN_POINT ( 'NONE',  ( -1.094772975963752103E-17, -1.590059055064346305, -0.1787899950787401882 ) ) ;
#11371=CARTESIAN_POINT ( 'NONE',  ( 0.1270800023317771588, -1.354374518244462422, -0.1270800023317771588 ) ) ;
#11377=CARTESIAN_POINT ( 'NONE',  ( -0.07810294628632777347, 0.1299212598425197041, 0.1504079689250619467 ) ) ;
#11393=CARTESIAN_POINT ( 'NONE',  ( -0.07444174185955065859, -0.008409951315329022153, -0.1797182628040039087 ) ) ;
#11398=CARTESIAN_POINT ( 'NONE',  ( 0.1264236179284866091, -0.1727362204186775607, -0.1264236179284866091 ) ) ;
#11402=CARTESIAN_POINT ( 'NONE',  ( 0.1888229765471286237, -0.07899262986800696662, -0.1764160547655181654 ) ) ;
#11405=CARTESIAN_POINT ( 'NONE',  ( 0.1113553986120547346, 0.03641732294217271682, 0.1113553986120547346 ) ) ;
#11413=CARTESIAN_POINT ( 'NONE',  ( 0.07405724077823318263, -0.8160688501190034305, -0.1787899950787401604 ) ) ;
#11423=CARTESIAN_POINT ( 'NONE',  ( -0.1264236179284866091, -0.4827755904974173617, -0.1264236179284866091 ) ) ;
#11425=( BOUNDED_SURFACE ( )  B_SPLINE_SURFACE ( 1, 2, ( 
 ( #30718, #11309, #1207, #44571, #37888, #12258, #11542, #25923, #44810, #37166, #4551, #37644, #40505, #7931, #36938, #22549, #4088, #41195, #8401, #18711, #11790, #26407, #23029, #33370, #19184, #4312, #26880, #41441, #19666, #34308, #33606, #719, #8160, #22788, #33843, #23741, #34529, #27607, #1685, #46232, #35251, #9367, #35480, #27844, #42159, #2620, #42629, #9837, #35011, #17022, #2159, #2386, #38347, #41915, #17253, #45290, #16556, #12969, #23991, #41679, #31659, #27129, #13437, #46002, #12506, #5523, #20137, #34783, #5282, #31185, #38590, #16786, #28066, #8884, #1924, #31425, #16332, #24447, #13210, #39046, #6212, #19898, #30954, #5766, #23519, #20607, #38823, #12742, #20371, #9605, #38122, #42406, #9126, #24227, #20841, #45520, #5986, #27373, #45759, #25405, #17950, #32608, #10309, #21071, #14139, #35708, #32840, #21799, #43348, #22022, #14376, #10552, #36648, #29275, #43823, #3344, #18200, #47196, #36424, #24922, #28536, #3808, #31891, #3094, #46947, #25151, #28292, #47436, #13654, #14604, #29023, #46470, #39514, #6688, #21306, #39279, #17719, #39741, #43581, #11022, #42854, #35934, #10795, #17481, #25640, #39983, #40215, #7406, #6453, #32115, #6928, #10063, #7174, #24682, #46702, #43103, #32369, #34022, #438, #4257, #7635, #44986, #663, #1146, #11256, #29970, #15091, #906, #37831, #29738, #44280, #33790, #33315, #11483, #22972, #33547, #22251, #15804, #18892, #26105, #15317, #37338, #40678, #30432, #44517, #23218, #37109, #8346, #7875, #22490, #15569, #26353, #22733, #4488, #36882, #18424, #33073, #37579, #30208, #12196, #4740, #4038, #200, #44752, #11970, #19367, #26823, #14847, #41379, #29511, #8579, #25867, #44059, #40449, #42571, #38294, #35186, #1864, #9780, #23683, #42351, #19843, #34472, #34954, #1622, #5215, #16500, #23458, #24390, #4989, #9546, #5463, #2333, #24167, #38060, #19609, #9303, #45461, #31130, #31365, #34248, #8823, #1378, #16271, #45224, #5701, #2099, #16036, #20078, #34725, #16729, #12446, #12916, #12686, #45944, #38769, #20547, #13155, #27068, #30664, #27788, #38533, #20315, #27311, #41616, #45697, #41861, #5930, #16959, #27546, #9065, #31599, #42098, #23926, #46180, #13378, #28006, #10740, #28726, #43525, #32061, #35656, #11610, #38989, #10254, #6635, #3032, #35422, #25348, #20780, #39931, #39684, #29854, #46649, #13834, #28477, #46415, #24859, #21255, #43295, #7118, #44395, #17424, #25093, #10010, #21742, #10495, #36373, #3529, #13593, #24623, #17663, #2560, #14323, #32551, #6398, #18142, #35879, #32785, #21010, #39459, #28231, #47380, #32311, #14552, #31829, #46890, #2795, #21491, #6159, #43047, #14080, #6870, #39223, #36123, #17193, #3278, #42794, #47138, #28968, #33907, #41259, #45106, #4614, #41741, #8225, #12081, #15441, #5332, #8459, #8945, #19003, #37707, #22851, #8700, #45575, #37466, #19248, #26940, #26469, #41031, #30782, #23089, #30095, #23565, #26705, #1028, #4860, #12324, #15684, #38169, #19486, #31006, #44869, #16151, #30321, #34134, #23336, #1264, #15917, #30544, #44627, #26232, #40798, #45349, #41494, #19952, #12562, #11842, #7991, #37949, #5097, #19721, #34359, #22616, #1496, #37228, #27187, #33666, #34592, #1742, #16387, #4373, #27896, #24506, #5583, #20663, #9428, #9893, #31946, #28350, #20900, #34840, #17544, #6274, #46298, #13489, #38648, #1985, #42458, #16615, #13714, #2679, #24279, #2908, #42680, #9663, #32181, #10131, #24739, #2444, #46532, #17072, #17310, #5823, #24048, #12797, #27431, #31475, #38874, #6039, #9180, #42919, #41972, #39336, #28120, #23796, #20431, #35065, #2216, #20189, #46059, #35307, #31713, #6514, #38412, #16835, #39101, #31242, #21133, #35539, #35768, #45819, #13028, #27665, #42226, #13267, #47452, #18216, #39530, #43842, #6947, #13906, #21322, #6467, #17970, #3825, #14625, #36444, #17497, #29294, #3111, #21085, #14391, #11043, #24693, #32858, #43362, #21568, #10812, #10569, #21816, #43121, #7191, #3596, #35953, #25659, #29041, #40235, #22041, #25171, #32624, #10325, #7423, #47211, #36667, #18446, #33095, #14866, #39755, #17734, #36206, #29525, #24937, #32384, #216, #44076, #6709, #39294, #35725, #2860, #3358, #46965, #32128, #14154, #46720, #28798, #43600, #25424, #39998, #18672, #15338, #11272, #928, #11751, #41162, #34042, #29991, #4057, #26372, #44535, #15108, #40931, #41404, #37854, #29753, #8127, #26610, #44771, #45007, #44301, #12220, #23241, #8366, #4275, #5009, #16059, #18909, #8601, #22750, #30224, #15586, #15826, #22267, #11504, #1167, #22992, #37356, #11987, #33812, #7650, #33332, #36903, #455, #19391, #26126, #26843, #19145, #683, #19628, #30451, #40696, #33565, #25885, #37604, #7892, #34269, #4764, #40467, #30686, #1399, #22510, #37126, #16524, #42373, #27091, #12938, #35213, #17221, #13402, #20572, #28032, #38314, #31153, #9571, #41642, #27571, #2351, #45250, #42591, #34493, #41881, #8846, #38559, #24412, #16984, #24190, #38084, #31623, #23707, #23483, #34978, #46203, #12470, #38792, #45722, #42119, #31393, #9334, #5949, #1648, #27813, #9803, #9087, #39016, #2123, #6180, #20804, #23953, #5724, #30922, #35445, #20340, #2583, #5241, #19868, #16292, #16752, #5488, #45962, #45483, #12711, #20102, #27336, #34748, #1889, #13176, #18162, #7139, #32332, #21034, #13614, #10273, #31856, #29240, #39480, #28988, #36396, #39243, #35899, #46434, #21509, #46912, #14342, #3550, #3052, #24649, #14102, #17681, #35679, #28748, #14571, #10989, #2816, #43312, #47158, #17920, #32802, #17447, #47397, #43791, #43546, #24883, #25606, #36613, #6657, #40180, #10516, #3301, #36147, #7381, #42817, #32081, #21991, #10760, #25114, #32573, #6891, #28254, #6417, #10029, #46670, #3772, #13856, #28503, #39703, #21274, #43069, #25367, #3998, #11449, #33037, #11692, #40410, #4704, #33509, #164, #37795, #25833, #22450, #18395, #8072, #18851, #866, #41110, #37071, #11219, #621, #4224, #22212, #15281, #1109, #44951, #36842, #29931, #33756, #4449, #19334, #18619, #33983, #30401, #15526, #26066, #12161, #23179, #40635, #15770, #44476, #37298, #22694, #22933, #29472, #33279, #8302, #30169, #26317, #19084, #40873, #14811, #7597, #44017, #404, #26551, #15054, #26785, #44709, #7838, #41344, #37543, #44246, #11931, #8545, #45659, #27032, #38735, #20042, #19575, #24357, #27752, #35151, #45429, #23647, #2067, #34220, #34681, #42317, #1347, #20516, #41584, #1583, #16003 ),
 ( #24132, #1827, #2293, #34437, #38258, #8786, #31565, #16462, #16923, #23422, #31099, #16235, #34922, #30625, #30868, #12648, #5667, #5184, #19805, #9509, #12878, #38024, #46146, #5422, #27273, #27511, #23886, #41822, #13343, #42063, #9741, #9267, #5902, #9024, #16698, #27972, #38495, #20274, #31326, #45903, #13119, #42537, #14285, #10214, #31799, #6599, #24818, #42755, #39419, #21703, #18105, #9975, #21213, #6830, #25055, #25304, #24587, #39894, #3489, #21450, #32023, #32747, #43732, #46613, #36337, #2992, #10455, #28686, #43490, #17157, #39184, #28927, #36080, #35843, #43255, #14039, #35387, #13561, #46382, #28197, #47092, #6357, #7078, #43005, #28442, #47345, #10698, #20972, #17626, #6119, #32270, #35617, #14517, #46850, #20744, #10935, #29184, #38955, #39649, #3236, #17866, #2760, #32509, #17384, #41062, #4408, #109, #25787, #40126, #40592, #15476, #26264, #29882, #3722, #40826, #7548, #7325, #37028, #8020, #25555, #22651, #29658, #26016, #15238, #44198, #11642, #43969, #37256, #19037, #36795, #33704, #18805, #812, #44659, #11398, #4179, #40357, #30123, #33462, #44427, #11876, #26503, #21942, #7785, #3948, #22400, #36562, #22158, #33229, #18343, #32985, #18572, #14754, #29425, #11171, #356, #579, #15006, #46762, #20895, #18254, #17538, #35760, #14194, #14, #43640, #32663, #2901, #10851, #43159, #32173, #21613, #25464, #35534, #14431, #39568, #47001, #36247, #6745, #18009, #24973, #3398, #47249, #21364, #29083, #40038, #36479, #32896, #35991, #43398, #3632, #14663, #29337, #43880, #25701, #9897, #13717, #9432, #20193, #42229, #28354, #41977, #45823, #20667, #38878, #12801, #39105, #6279, #20902, #38654, #45579, #38175, #13033, #8949, #35543, #27669, #2448, #2685, #16392, #5827, #23569, #46064, #27900, #17313, #31951, #42463, #1749, #9667, #24283, #9184, #5337, #19958, #34598, #23800, #31013, #38416, #25472, #18490, #46770, #268, #32185, #7240, #36002, #13956, #39576, #17786, #32433, #3406, #21861, #3641, #21, #14205, #18022, #32905, #20330, #41873, #12929, #45713, #19619, #45238, #34259, #30677, #31382, #1390, #24181, #27325, #12700, #16974, #45955, #8837, #16283, #37843, #16515, #12462, #9559, #5478, #5001, #42581, #13167, #5939, #30914, #9078, #34968, #16049, #20093, #27801, #23231, #38783, #27080, #20560, #41630, #35202, #2343, #38549, #45473, #31613, #28021, #23697, #46194, #34739, #42111, #27562, #42365, #23472, #38074, #13392, #2112, #31144, #9320, #23942, #5229, #19857, #34484, #1637, #5713, #16743, #10753, #13845, #43058, #3543, #17911, #42807, #17437, #6173, #32322, #32071, #43536, #24869, #2572, #9793, #32562, #21753, #14091, #28736, #21500, #17208, #10506, #47150, #25104, #18154, #3291, #14334, #28979, #32794, #47390, #19077, #8062, #36606, #33749, #22206, #25600, #33502, #858, #43781, #37292, #15047, #26060, #29925, #29697, #40866, #155, #26310, #22688, #40404, #4443, #615, #15517, #41102, #44238, #4217, #29465, #30160, #18846, #44701, #8296, #11919, #33976, #11443, #7592, #40630, #1102, #14806, #36838, #26542, #22923, #44010, #37536, #4695, #19327, #7829, #33029, #40171, #3990, #10983, #15760, #18612, #7373, #21984, #3765, #396, #18387, #15274, #22444, #11214, #25827, #37065, #33272, #44470, #11685, #34209, #2232, #13728, #10145, #1337, #46077, #46319, #17088, #20914, #42474, #21145, #13503, #27911, #35780, #28366, #42935, #20681, #2697, #35321, #35553, #24062, #27680, #2922, #30393, #16851, #13278, #9679, #26778, #17324, #12154, #31960, #31726, #44942, #38669, #5838, #20446, #37785, #31493, #24294, #2461, #46545, #41337, #9446, #28135, #15993, #24754, #42692, #39350, #6531, #4937, #30616, #38892, #8536, #23168, #24519, #45180, #19563, #6055, #12401, #42243, #39117, #35084, #44130, #47269, #33158, #10388, #29104, #14218, #34, #36953, #28859, #43418, #18272, #17798, #32445, #22093, #32680, #21386, #279, #3417, #25229, #14448, #36495, #10626, #14924, #43659, #22325, #36267, #7474, #47023, #39817, #14683, #7006, #21633, #10867, #36011, #17557, #32195, #36720, #18034, #29589, #3882, #3168, #46782, #21875, #25487, #40053, #43898, #13969, #7253, #28619, #3651, #24993, #32915, #29356, #7710, #11097, #25720, #40289, #39588, #18501, #11328, #25940, #6769, #40520, #43179, #41208, #26661, #503, #26185, #15162, #11561, #12272, #29806, #5059, #37901, #7949, #19676, #16109, #19439, #44585, #30733, #8897, #11803, #1450, #15637, #23042, #8414, #8650, #15397, #34318, #40753, #15870, #22801, #37660, #4816, #44353, #22568, #37183, #4327, #26893, #18960, #45302, #8175, #40990, #12520, #41450, #33620, #26422, #18729, #44826, #735, #41695, #19201, #33389, #23529, #23288, #4110, #37409, #4567, #1219, #30041, #33860, #979, #30274, #12038, #34089, #30498, #45058, #31433, #17268, #13447, #2400, #30964, #28076, #16567, #19912, #27854, #42637, #38132, #31670, #9380, #20380, #24236, #24001, #35266, #41928, #20617, #17033, #34793, #46248, #42413, #9848, #35495, #38600, #46014, #23751, #24458, #13219, #39060, #2634, #6228, #28302, #5774, #1933, #35020, #42869, #9134, #31197, #20852, #31904, #38362, #46485, #13666, #10082, #2169, #27384, #34542, #45770, #5292, #1694, #12980, #16343, #45531, #12754, #42172, #5533, #9617, #16792, #20148, #27619, #38833, #5997, #6560, #10169, #46570, #21168, #6312, #2947, #40230, #36901, #37125, #7890, #40464, #4055, #26123, #37354, #11985, #213, #22508, #7419, #26370, #40694, #22748, #8125, #29290, #22037, #453, #18212, #44533, #15336, #36663, #40929, #18670, #4507, #3821, #7647, #11039, #926, #33330, #19143, #14620, #15106, #18441, #18907, #41160, #33092, #14863, #33563, #29522, #44073, #33809, #29751, #25654, #15584, #22264, #11270, #44299, #681, #25882, #30222, #11502, #26608, #29988, #11749, #44769, #21812, #36440, #3592, #32854, #47448, #43838, #13174, #27811, #45720, #27089, #5722, #27569, #26841, #22990, #12709, #34267, #34491, #34746, #37601, #12218, #4762, #41401, #1165, #9085, #5485, #45960, #41640, #23481, #20100, #15824, #16290, #5007, #19388, #34040, #31391, #1397, #30449, #8364, #1887, #41879, #23705, #16057, #45005, #38082, #8599, #9331, #12936, #19866, #23239, #38312, #5239, #30684, #20338, #34976, #45481, #42117, #27334, #23951, #45247, #12468, #8844, #1645, #30920, #16522, #31151, #38557, #2121, #16750, #14100, #43067, #33223, #35443, #17219, #31854, #2349, #46432 ),
 ( #10271, #39478, #349, #28252, #10027, #6655, #35211, #2814, #39014, #24188, #20570, #18567, #6178, #16982, #14998, #35897, #28501, #24881, #20802, #31621, #24647, #46201, #43310, #32330, #6415, #42371, #21272, #39241, #9569, #39701, #6889, #32079, #28746, #46668, #46910, #2581, #13612, #38790, #5947, #42815, #21032, #35677, #13400, #10514, #28030, #25112, #3050, #42589, #17445, #13854, #17679, #9801, #21507, #36145, #3299, #24410, #15943, #11634, #22877, #18797, #12106, #41053, #8484, #41284, #22394, #33454, #30116, #11393, #30344, #15709, #15227, #26731, #803, #23119, #29874, #4398, #37020, #19510, #15468, #37732, #7777, #44648, #44416, #19272, #45130, #26253, #40815, #37489, #570, #8012, #4887, #33693, #22641, #34159, #19027, #37246, #11866, #8251, #26491, #1288, #4643, #30568, #33928, #29649, #1051, #44190, #26006, #40585, #44893, #4173, #14661, #29567, #18006, #21611, #44337, #24328, #43638, #40035, #36477, #20715, #44114, #6089, #11308, #25699, #15144, #32661, #47247, #14429, #31767, #10848, #7232, #29334, #40504, #29791, #3396, #11080, #42730, #25922, #43878, #7691, #22307, #46350, #9945, #3630, #35355, #258, #18484, #39794, #36937, #21851, #4087, #6987, #25462, #13534, #18709, #18252, #33369, #17125, #32894, #36244, #7457, #38927, #29081, #12, #40271, #24550, #22078, #488, #36703, #28169, #2502, #3864, #33132, #14906, #30482, #37395, #41677, #23028, #16328, #30261, #1433, #26406, #40970, #41440, #8158, #11789, #37642, #30027, #30953, #11541, #16094, #44809, #8882, #30715, #44570, #26166, #15859, #4550, #4796, #37886, #40735, #15378, #7929, #22787, #4311, #12257, #8636, #1682, #12021, #26646, #23270, #18944, #19424, #19183, #22548, #37164, #34526, #33842, #33605, #718, #5044, #45042, #26879, #963, #15621, #41194, #34077, #12504, #45288, #1205, #19664, #34306, #27127, #23517, #38120, #5280, #19895, #23987, #28287, #42401, #2842, #16783, #35476, #12965, #27606, #28063, #42156, #45756, #9602, #31182, #17478, #45518, #2615, #31421, #10060, #17250, #9364, #12740, #2382, #38586, #24223, #24442, #27370, #1921, #41912, #5763, #38344, #46228, #42625, #35704, #13207, #27841, #9834, #5520, #5982, #20368, #9124, #23740, #21067, #35007, #20135, #34781, #39042, #31655, #13432, #2155, #38820, #20602, #35247, #46466, #31887, #17018, #6208, #20837, #13650, #24679, #39275, #6450, #36420, #18421, #3578, #33069, #25146, #6923, #4032, #32112, #3341, #47192, #43577, #28531, #14842, #39510, #11252, #32836, #22246, #10791, #25401, #39978, #6684, #7171, #18196, #11019, #36878, #46698, #21302, #17714, #23679, #9776, #9542, #35419, #38986, #12679, #5458, #31361, #1617, #28003, #42568, #34720, #24387, #34951, #17192, #1859, #38529, #41856, #31824, #2095, #46411, #45456, #16725, #16497, #35183, #5211, #31127, #45693, #2329, #12913, #27543, #13590, #20310, #9060, #28227, #10006, #19839, #5698, #42096, #45941, #34467, #9300, #23921, #16267, #30900, #13151, #27306, #27785, #42346, #24164, #38766, #21007, #17659, #39219, #36594, #46886, #36369, #43765, #46645, #43291, #6395, #28964, #39679, #21737, #14547, #10491, #32057, #6866, #25089, #43043, #21487, #21969, #18374, #10250, #36119, #7114, #25343, #25585, #24856, #40158, #3751, #3524, #32308, #33016, #43999, #14074, #138, #3274, #10735, #43521, #10967, #3028, #7357, #28473, #18136, #17898, #39927, #32781, #35653, #13832, #2791, #39455, #47375, #17420, #14791, #32546, #28722, #29452, #29217, #6631, #47134, #21250, #11201, #35875, #12140, #40853, #40390, #45165, #1086, #8523, #18834, #44459, #22910, #7579, #8048, #15745, #25814, #41321, #15035, #22431, #22192, #19064, #4925, #30379, #37524, #18597, #44925, #4205, #36828, #15503, #26764, #3979, #19310, #11672, #22676, #11904, #26296, #4680, #29684, #8284, #33963, #37051, #23153, #30148, #37768, #19548, #37277, #33733, #11430, #34195, #843, #1323, #15980, #30601, #4432, #33259, #40621, #7815, #383, #33489, #26048, #44687, #44226, #605, #15262, #29909, #26527, #41087, #31539, #30844, #27008, #16673, #38235, #38472, #38713, #41552, #16213, #8760, #45411, #5162, #13093, #9487, #2506, #45637, #27489, #24106, #19781, #20253, #9001, #23397, #38001, #35361, #23625, #34415, #17130, #5883, #45881, #27726, #5393, #1558, #42040, #12624, #13318, #2274, #23860, #31772, #42288, #9242, #12387, #9719, #24333, #2040, #46120, #31301, #16899, #20016, #34655, #27247, #41801, #31073, #5642, #34899, #1805, #27949, #16444, #42516, #20490, #12856, #35128, #38931, #6093, #20718, #32242, #14012, #32486, #14489, #36537, #24795, #43462, #42979, #3464, #25275, #47315, #32723, #20949, #10188, #21425, #42733, #21678, #39863, #21185, #18075, #43225, #29148, #35818, #46824, #35593, #40101, #10430, #43704, #2732, #7053, #2965, #36309, #18318, #7295, #21915, #46354, #13538, #28172, #9948, #24557, #36765, #1030, #18779, #40565, #548, #4375, #11371, #15686, #29856, #25982, #33668, #33202, #324, #37468, #15205, #3924, #30323, #33433, #7755, #44396, #19005, #22373, #44871, #11612, #37708, #4153, #22852, #14974, #29630, #15443, #44169, #36997, #26233, #18546, #4862, #32956, #4616, #40799, #12083, #19250, #7992, #78, #37230, #22618, #781, #11844, #14726, #30097, #29399, #44629, #25761, #26471, #41033, #23090, #8227, #33909, #26707, #40330, #41261, #8461, #43943, #11141, #7517, #22138, #41496, #24281, #13031, #5585, #20191, #45351, #8702, #1744, #23338, #20433, #9430, #31008, #9665, #1987, #16389, #38876, #16837, #31477, #9182, #38650, #23797, #24050, #12564, #16153, #19488, #34136, #38171, #34594, #45577, #15919, #5825, #1266, #35067, #34842, #30546, #27189, #41743, #8947, #26942, #5334, #12799, #38414, #2218, #45108, #23567, #16617, #37951, #46061, #31244, #13269, #27898, #5099, #19723, #27433, #12326, #42228, #27667, #34360, #42460, #41974, #1498, #30784, #19954, #45821, #32668, #35769, #21621, #46300, #17546, #2681, #36001, #25471, #17312, #18018, #43406, #43649, #6516, #31948, #39338, #10858, #24508, #46534, #3159, #17784, #9895, #39806, #6994, #28845, #21135, #42682, #35309, #13716, #6041, #3405, #28351, #32432, #10616, #13491, #10133, #20665, #43169, #2910, #47010, #25215, #24741, #28122, #32183, #46769, #39103, #13955, #36254, #47257, #6276, #28606, #21375, #39575, #14437, #20901, #29090, #2446, #14202, #42921, #17074, #31715, #10374, #35541, #24981, #6753, #29796 ) ),
 .UNSPECIFIED., .F., .F., .T. ) 
 B_SPLINE_SURFACE_WITH_KNOTS ( ( 2, 1, 2 ),
 ( 3, 2, 2, 2, 2, 2, 2, 2, 2, 2, 2, 2, 2, 2, 2, 2, 2, 2, 2, 2, 2, 2, 2, 2, 2, 2, 2, 2, 2, 2, 2, 2, 2, 2, 2, 2, 2, 2, 2, 2, 2, 2, 2, 2, 2, 2, 2, 2, 2, 2, 2, 2, 2, 2, 2, 2, 2, 2, 2, 2, 2, 2, 2, 2, 2, 2, 2, 2, 2, 2, 2, 2, 2, 2, 2, 2, 2, 2, 2, 2, 2, 2, 2, 2, 2, 2, 2, 2, 2, 2, 2, 2, 2, 2, 2, 2, 2, 2, 2, 2, 2, 2, 2, 2, 2, 2, 2, 2, 2, 2, 2, 2, 2, 2, 2, 2, 2, 2, 2, 2, 2, 2, 2, 2, 2, 2, 2, 2, 2, 2, 2, 2, 2, 2, 2, 2, 2, 2, 2, 2, 2, 2, 2, 2, 2, 2, 2, 2, 2, 2, 2, 2, 2, 2, 2, 2, 2, 2, 2, 2, 2, 2, 2, 2, 2, 2, 2, 2, 2, 2, 2, 2, 2, 2, 2, 2, 2, 2, 2, 2, 2, 2, 2, 2, 2, 2, 2, 2, 2, 2, 2, 2, 2, 2, 2, 2, 2, 2, 2, 2, 2, 2, 2, 2, 2, 2, 2, 2, 2, 2, 2, 2, 2, 2, 2, 2, 2, 2, 2, 2, 2, 2, 2, 2, 2, 2, 2, 2, 2, 2, 2, 2, 2, 2, 2, 2, 2, 2, 2, 2, 2, 2, 2, 2, 2, 2, 2, 2, 2, 2, 2, 2, 2, 2, 2, 2, 2, 2, 2, 2, 2, 2, 2, 2, 2, 2, 2, 2, 2, 2, 2, 2, 2, 2, 2, 2, 2, 2, 2, 2, 2, 2, 2, 2, 2, 2, 2, 2, 2, 2, 2, 2, 2, 2, 2, 2, 2, 2, 2, 2, 2, 2, 2, 2, 2, 2, 2, 2, 2, 2, 2, 2, 2, 2, 2, 2, 2, 2, 2, 2, 2, 2, 2, 2, 2, 2, 2, 2, 2, 2, 2, 2, 2, 2, 2, 2, 2, 2, 2, 2, 2, 2, 2, 2, 2, 2, 2, 2, 2, 2, 2, 2, 2, 2, 2, 2, 2, 2, 2, 2, 2, 2, 2, 2, 2, 2, 2, 2, 2, 2, 2, 2, 2, 2, 2, 2, 2, 2, 2, 2, 2, 2, 2, 2, 2, 2, 2, 2, 2, 2, 2, 2, 2, 2, 2, 2, 2, 2, 2, 2, 3 ),
 ( 0.000000000000000000, 1.000000000000000000, 1.043560847470196062 ),
 ( 0.000000000000000000, 0.002500000000000000052, 0.005000000000000000104, 0.007499999999999999722, 0.01000000000000000021, 0.01250000000000000069, 0.01499999999999999944, 0.01750000000000000167, 0.02000000000000000042, 0.02249999999999999917, 0.02500000000000000139, 0.02750000000000000014, 0.02999999999999999889, 0.03250000000000000111, 0.03500000000000000333, 0.03749999999999999861, 0.04000000000000000083, 0.04250000000000000305, 0.04499999999999999833, 0.04750000000000000056, 0.05000000000000000278, 0.05249999999999999806, 0.05500000000000000028, 0.05750000000000000250, 0.05999999999999999778, 0.06250000000000000000, 0.06500000000000000222, 0.06750000000000000444, 0.07000000000000000666, 0.07249999999999999500, 0.07499999999999999722, 0.07749999999999999944, 0.08000000000000000167, 0.08250000000000000389, 0.08500000000000000611, 0.08749999999999999445, 0.08999999999999999667, 0.09249999999999999889, 0.09500000000000000111, 0.09750000000000000333, 0.1000000000000000056, 0.1024999999999999939, 0.1049999999999999961, 0.1074999999999999983, 0.1100000000000000006, 0.1125000000000000028, 0.1150000000000000050, 0.1174999999999999933, 0.1199999999999999956, 0.1224999999999999978, 0.1250000000000000000, 0.1275000000000000022, 0.1300000000000000044, 0.1325000000000000067, 0.1350000000000000089, 0.1375000000000000111, 0.1400000000000000133, 0.1424999999999999878, 0.1449999999999999900, 0.1474999999999999922, 0.1499999999999999944, 0.1524999999999999967, 0.1549999999999999989, 0.1575000000000000011, 0.1600000000000000033, 0.1625000000000000056, 0.1650000000000000078, 0.1675000000000000100, 0.1700000000000000122, 0.1724999999999999867, 0.1749999999999999889, 0.1774999999999999911, 0.1799999999999999933, 0.1824999999999999956, 0.1849999999999999978, 0.1875000000000000000, 0.1900000000000000022, 0.1925000000000000044, 0.1950000000000000067, 0.1975000000000000089, 0.2000000000000000111, 0.2025000000000000133, 0.2049999999999999878, 0.2074999999999999900, 0.2099999999999999922, 0.2124999999999999944, 0.2149999999999999967, 0.2174999999999999989, 0.2200000000000000011, 0.2225000000000000033, 0.2250000000000000056, 0.2275000000000000078, 0.2300000000000000100, 0.2325000000000000122, 0.2349999999999999867, 0.2374999999999999889, 0.2399999999999999911, 0.2424999999999999933, 0.2449999999999999956, 0.2474999999999999978, 0.2500000000000000000, 0.2525000000000000022, 0.2550000000000000044, 0.2575000000000000067, 0.2600000000000000089, 0.2625000000000000111, 0.2650000000000000133, 0.2675000000000000155, 0.2700000000000000178, 0.2725000000000000200, 0.2750000000000000222, 0.2775000000000000244, 0.2800000000000000266, 0.2824999999999999734, 0.2849999999999999756, 0.2874999999999999778, 0.2899999999999999800, 0.2924999999999999822, 0.2949999999999999845, 0.2974999999999999867, 0.2999999999999999889, 0.3024999999999999911, 0.3049999999999999933, 0.3074999999999999956, 0.3099999999999999978, 0.3125000000000000000, 0.3150000000000000022, 0.3175000000000000044, 0.3200000000000000067, 0.3225000000000000089, 0.3250000000000000111, 0.3275000000000000133, 0.3300000000000000155, 0.3325000000000000178, 0.3350000000000000200, 0.3375000000000000222, 0.3400000000000000244, 0.3425000000000000266, 0.3449999999999999734, 0.3474999999999999756, 0.3499999999999999778, 0.3524999999999999800, 0.3549999999999999822, 0.3574999999999999845, 0.3599999999999999867, 0.3624999999999999889, 0.3649999999999999911, 0.3674999999999999933, 0.3699999999999999956, 0.3724999999999999978, 0.3750000000000000000, 0.3775000000000000022, 0.3800000000000000044, 0.3825000000000000067, 0.3850000000000000089, 0.3875000000000000111, 0.3900000000000000133, 0.3925000000000000155, 0.3950000000000000178, 0.3975000000000000200, 0.4000000000000000222, 0.4025000000000000244, 0.4050000000000000266, 0.4074999999999999734, 0.4099999999999999756, 0.4124999999999999778, 0.4149999999999999800, 0.4174999999999999822, 0.4199999999999999845, 0.4224999999999999867, 0.4249999999999999889, 0.4274999999999999911, 0.4299999999999999933, 0.4324999999999999956, 0.4349999999999999978, 0.4375000000000000000, 0.4400000000000000022, 0.4425000000000000044, 0.4450000000000000067, 0.4475000000000000089, 0.4500000000000000111, 0.4525000000000000133, 0.4550000000000000155, 0.4575000000000000178, 0.4600000000000000200, 0.4625000000000000222, 0.4650000000000000244, 0.4675000000000000266, 0.4699999999999999734, 0.4724999999999999756, 0.4749999999999999778, 0.4774999999999999800, 0.4799999999999999822, 0.4824999999999999845, 0.4849999999999999867, 0.4874999999999999889, 0.4899999999999999911, 0.4924999999999999933, 0.4949999999999999956, 0.4974999999999999978, 0.5000000000000000000, 0.5024999999999999467, 0.5050000000000000044, 0.5074999999999999512, 0.5100000000000000089, 0.5124999999999999556, 0.5150000000000000133, 0.5174999999999999600, 0.5200000000000000178, 0.5224999999999999645, 0.5250000000000000222, 0.5274999999999999689, 0.5300000000000000266, 0.5324999999999999734, 0.5350000000000000311, 0.5374999999999999778, 0.5400000000000000355, 0.5424999999999999822, 0.5450000000000000400, 0.5474999999999999867, 0.5500000000000000444, 0.5524999999999999911, 0.5550000000000000488, 0.5574999999999999956, 0.5600000000000000533, 0.5625000000000000000, 0.5649999999999999467, 0.5675000000000000044, 0.5699999999999999512, 0.5725000000000000089, 0.5749999999999999556, 0.5775000000000000133, 0.5799999999999999600, 0.5825000000000000178, 0.5849999999999999645, 0.5875000000000000222, 0.5899999999999999689, 0.5925000000000000266, 0.5949999999999999734, 0.5975000000000000311, 0.5999999999999999778, 0.6025000000000000355, 0.6049999999999999822, 0.6075000000000000400, 0.6099999999999999867, 0.6125000000000000444, 0.6149999999999999911, 0.6175000000000000488, 0.6199999999999999956, 0.6225000000000000533, 0.6250000000000000000, 0.6274999999999999467, 0.6300000000000000044, 0.6324999999999999512, 0.6350000000000000089, 0.6374999999999999556, 0.6400000000000000133, 0.6424999999999999600, 0.6450000000000000178, 0.6474999999999999645, 0.6500000000000000222, 0.6524999999999999689, 0.6550000000000000266, 0.6574999999999999734, 0.6600000000000000311, 0.6624999999999999778, 0.6650000000000000355, 0.6674999999999999822, 0.6700000000000000400, 0.6724999999999999867, 0.6750000000000000444, 0.6774999999999999911, 0.6800000000000000488, 0.6824999999999999956, 0.6850000000000000533, 0.6875000000000000000, 0.6899999999999999467, 0.6925000000000000044, 0.6949999999999999512, 0.6975000000000000089, 0.6999999999999999556, 0.7025000000000000133, 0.7049999999999999600, 0.7075000000000000178, 0.7099999999999999645, 0.7125000000000000222, 0.7149999999999999689, 0.7175000000000000266, 0.7199999999999999734, 0.7225000000000000311, 0.7249999999999999778, 0.7275000000000000355, 0.7299999999999999822, 0.7325000000000000400, 0.7349999999999999867, 0.7375000000000000444, 0.7399999999999999911, 0.7425000000000000488, 0.7449999999999999956, 0.7475000000000000533, 0.7500000000000000000, 0.7524999999999999467, 0.7550000000000000044, 0.7574999999999999512, 0.7600000000000000089, 0.7624999999999999556, 0.7650000000000000133, 0.7674999999999999600, 0.7700000000000000178, 0.7724999999999999645, 0.7750000000000000222, 0.7774999999999999689, 0.7800000000000000266, 0.7824999999999999734, 0.7850000000000000311, 0.7874999999999999778, 0.7900000000000000355, 0.7924999999999999822, 0.7950000000000000400, 0.7974999999999999867, 0.8000000000000000444, 0.8024999999999999911, 0.8050000000000000488, 0.8074999999999999956, 0.8100000000000000533, 0.8125000000000000000, 0.8149999999999999467, 0.8175000000000000044, 0.8199999999999999512, 0.8225000000000000089, 0.8249999999999999556, 0.8275000000000000133, 0.8299999999999999600, 0.8325000000000000178, 0.8349999999999999645, 0.8375000000000000222, 0.8399999999999999689, 0.8425000000000000266, 0.8449999999999999734, 0.8475000000000000311, 0.8499999999999999778, 0.8525000000000000355, 0.8549999999999999822, 0.8575000000000000400, 0.8599999999999999867, 0.8625000000000000444, 0.8649999999999999911, 0.8675000000000000488, 0.8699999999999999956, 0.8725000000000000533, 0.8750000000000000000, 0.8774999999999999467, 0.8800000000000000044, 0.8824999999999999512, 0.8850000000000000089, 0.8874999999999999556, 0.8900000000000000133, 0.8924999999999999600, 0.8950000000000000178, 0.8974999999999999645, 0.9000000000000000222, 0.9024999999999999689, 0.9050000000000000266, 0.9074999999999999734, 0.9100000000000000311, 0.9124999999999999778, 0.9150000000000000355, 0.9174999999999999822, 0.9200000000000000400, 0.9224999999999999867, 0.9250000000000000444, 0.9274999999999999911, 0.9300000000000000488, 0.9324999999999999956, 0.9350000000000000533, 0.9375000000000000000, 0.9399999999999999467, 0.9425000000000000044, 0.9449999999999999512, 0.9475000000000000089, 0.9499999999999999556, 0.9525000000000000133, 0.9549999999999999600, 0.9575000000000000178, 0.9599999999999999645, 0.9625000000000000222, 0.9649999999999999689, 0.9675000000000000266, 0.9699999999999999734, 0.9725000000000000311, 0.9749999999999999778, 0.9775000000000000355, 0.9799999999999999822, 0.9825000000000000400, 0.9849999999999999867, 0.9875000000000000444, 0.9899999999999999911, 0.9925000000000000488, 0.9949999999999999956, 0.9975000000000000533, 1.000000000000000000 ),
 .UNSPECIFIED. ) 
 GEOMETRIC_REPRESENTATION_ITEM ( )  RATIONAL_B_SPLINE_SURFACE ( (
 ( 1.000000000000000000, 0.9238795325112869605, 1.000000000000000000, 0.9238795325112869605, 1.000000000000000000, 0.9238795325112869605, 1.000000000000000000, 0.9238795325112869605, 1.000000000000000000, 0.9238795325112869605, 1.000000000000000000, 0.9238795325112869605, 1.000000000000000000, 0.9238795325112869605, 1.000000000000000000, 0.9238795325112869605, 1.000000000000000000, 0.9238795325112869605, 1.000000000000000000, 0.9238795325112869605, 1.000000000000000000, 0.9238795325112869605, 1.000000000000000000, 0.9238795325112869605, 1.000000000000000000, 0.9238795325112869605, 1.000000000000000000, 0.9238795325112869605, 1.000000000000000000, 0.9238795325112869605, 1.000000000000000000, 0.9238795325112869605, 1.000000000000000000, 0.9238795325112869605, 1.000000000000000000, 0.9238795325112869605, 1.000000000000000000, 0.9238795325112869605, 1.000000000000000000, 0.9238795325112869605, 1.000000000000000000, 0.9238795325112869605, 1.000000000000000000, 0.9238795325112869605, 1.000000000000000000, 0.9238795325112869605, 1.000000000000000000, 0.9238795325112869605, 1.000000000000000000, 0.9238795325112869605, 1.000000000000000000, 0.9238795325112869605, 1.000000000000000000, 0.9238795325112869605, 1.000000000000000000, 0.9238795325112869605, 1.000000000000000000, 0.9238795325112869605, 1.000000000000000000, 0.9238795325112869605, 1.000000000000000000, 0.9238795325112869605, 1.000000000000000000, 0.9238795325112869605, 1.000000000000000000, 0.9238795325112869605, 1.000000000000000000, 0.9238795325112869605, 1.000000000000000000, 0.9238795325112869605, 1.000000000000000000, 0.9238795325112869605, 1.000000000000000000, 0.9238795325112869605, 1.000000000000000000, 0.9238795325112869605, 1.000000000000000000, 0.9238795325112869605, 1.000000000000000000, 0.9238795325112869605, 1.000000000000000000, 0.9238795325112869605, 1.000000000000000000, 0.9238795325112869605, 1.000000000000000000, 0.9238795325112869605, 1.000000000000000000, 0.9238795325112869605, 1.000000000000000000, 0.9238795325112869605, 1.000000000000000000, 0.9238795325112869605, 1.000000000000000000, 0.9238795325112869605, 1.000000000000000000, 0.9238795325112869605, 1.000000000000000000, 0.9238795325112869605, 1.000000000000000000, 0.9238795325112869605, 1.000000000000000000, 0.9238795325112869605, 1.000000000000000000, 0.9238795325112869605, 1.000000000000000000, 0.9238795325112869605, 1.000000000000000000, 0.9238795325112869605, 1.000000000000000000, 0.9238795325112869605, 1.000000000000000000, 0.9238795325112869605, 1.000000000000000000, 0.9238795325112869605, 1.000000000000000000, 0.9238795325112869605, 1.000000000000000000, 0.9238795325112869605, 1.000000000000000000, 0.9238795325112869605, 1.000000000000000000, 0.9238795325112869605, 1.000000000000000000, 0.9238795325112869605, 1.000000000000000000, 0.9238795325112869605, 1.000000000000000000, 0.9238795325112869605, 1.000000000000000000, 0.9238795325112869605, 1.000000000000000000, 0.9238795325112869605, 1.000000000000000000, 0.9238795325112869605, 1.000000000000000000, 0.9238795325112869605, 1.000000000000000000, 0.9238795325112869605, 1.000000000000000000, 0.9238795325112869605, 1.000000000000000000, 0.9238795325112869605, 1.000000000000000000, 0.9238795325112869605, 1.000000000000000000, 0.9238795325112869605, 1.000000000000000000, 0.9238795325112869605, 1.000000000000000000, 0.9238795325112869605, 1.000000000000000000, 0.9238795325112869605, 1.000000000000000000, 0.9238795325112869605, 1.000000000000000000, 0.9238795325112869605, 1.000000000000000000, 0.9238795325112869605, 1.000000000000000000, 0.9238795325112869605, 1.000000000000000000, 0.9238795325112869605, 1.000000000000000000, 0.9238795325112869605, 1.000000000000000000, 0.9238795325112869605, 1.000000000000000000, 0.9238795325112869605, 1.000000000000000000, 0.9238795325112869605, 1.000000000000000000, 0.9238795325112869605, 1.000000000000000000, 0.9238795325112869605, 1.000000000000000000, 0.9238795325112869605, 1.000000000000000000, 0.9238795325112869605, 1.000000000000000000, 0.9238795325112869605, 1.000000000000000000, 0.9238795325112869605, 1.000000000000000000, 0.9238795325112869605, 1.000000000000000000, 0.9238795325112869605, 1.000000000000000000, 0.9238795325112869605, 1.000000000000000000, 0.9238795325112869605, 1.000000000000000000, 0.9238795325112869605, 1.000000000000000000, 0.9238795325112869605, 1.000000000000000000, 0.9238795325112869605, 1.000000000000000000, 0.9238795325112869605, 1.000000000000000000, 0.9238795325112869605, 1.000000000000000000, 0.9238795325112869605, 1.000000000000000000, 0.9238795325112869605, 1.000000000000000000, 0.9238795325112869605, 1.000000000000000000, 0.9238795325112869605, 1.000000000000000000, 0.9238795325112869605, 1.000000000000000000, 0.9238795325112869605, 1.000000000000000000, 0.9238795325112869605, 1.000000000000000000, 0.9238795325112869605, 1.000000000000000000, 0.9238795325112869605, 1.000000000000000000, 0.9238795325112869605, 1.000000000000000000, 0.9238795325112869605, 1.000000000000000000, 0.9238795325112869605, 1.000000000000000000, 0.9238795325112869605, 1.000000000000000000, 0.9238795325112869605, 1.000000000000000000, 0.9238795325112869605, 1.000000000000000000, 0.9238795325112869605, 1.000000000000000000, 0.9238795325112869605, 1.000000000000000000, 0.9238795325112869605, 1.000000000000000000, 0.9238795325112869605, 1.000000000000000000, 0.9238795325112869605, 1.000000000000000000, 0.9238795325112869605, 1.000000000000000000, 0.9238795325112869605, 1.000000000000000000, 0.9238795325112869605, 1.000000000000000000, 0.9238795325112869605, 1.000000000000000000, 0.9238795325112869605, 1.000000000000000000, 0.9238795325112869605, 1.000000000000000000, 0.9238795325112869605, 1.000000000000000000, 0.9238795325112869605, 1.000000000000000000, 0.9238795325112869605, 1.000000000000000000, 0.9238795325112869605, 1.000000000000000000, 0.9238795325112869605, 1.000000000000000000, 0.9238795325112869605, 1.000000000000000000, 0.9238795325112869605, 1.000000000000000000, 0.9238795325112869605, 1.000000000000000000, 0.9238795325112869605, 1.000000000000000000, 0.9238795325112869605, 1.000000000000000000, 0.9238795325112869605, 1.000000000000000000, 0.9238795325112869605, 1.000000000000000000, 0.9238795325112869605, 1.000000000000000000, 0.9238795325112869605, 1.000000000000000000, 0.9238795325112869605, 1.000000000000000000, 0.9238795325112869605, 1.000000000000000000, 0.9238795325112869605, 1.000000000000000000, 0.9238795325112869605, 1.000000000000000000, 0.9238795325112869605, 1.000000000000000000, 0.9238795325112869605, 1.000000000000000000, 0.9238795325112869605, 1.000000000000000000, 0.9238795325112869605, 1.000000000000000000, 0.9238795325112869605, 1.000000000000000000, 0.9238795325112869605, 1.000000000000000000, 0.9238795325112869605, 1.000000000000000000, 0.9238795325112869605, 1.000000000000000000, 0.9238795325112869605, 1.000000000000000000, 0.9238795325112869605, 1.000000000000000000, 0.9238795325112869605, 1.000000000000000000, 0.9238795325112869605, 1.000000000000000000, 0.9238795325112869605, 1.000000000000000000, 0.9238795325112869605, 1.000000000000000000, 0.9238795325112869605, 1.000000000000000000, 0.9238795325112869605, 1.000000000000000000, 0.9238795325112869605, 1.000000000000000000, 0.9238795325112869605, 1.000000000000000000, 0.9238795325112869605, 1.000000000000000000, 0.9238795325112869605, 1.000000000000000000, 0.9238795325112869605, 1.000000000000000000, 0.9238795325112869605, 1.000000000000000000, 0.9238795325112869605, 1.000000000000000000, 0.9238795325112869605, 1.000000000000000000, 0.9238795325112869605, 1.000000000000000000, 0.9238795325112869605, 1.000000000000000000, 0.9238795325112869605, 1.000000000000000000, 0.9238795325112869605, 1.000000000000000000, 0.9238795325112869605, 1.000000000000000000, 0.9238795325112869605, 1.000000000000000000, 0.9238795325112869605, 1.000000000000000000, 0.9238795325112869605, 1.000000000000000000, 0.9238795325112869605, 1.000000000000000000, 0.9238795325112869605, 1.000000000000000000, 0.9238795325112869605, 1.000000000000000000, 0.9238795325112869605, 1.000000000000000000, 0.9238795325112869605, 1.000000000000000000, 0.9238795325112869605, 1.000000000000000000, 0.9238795325112869605, 1.000000000000000000, 0.9238795325112869605, 1.000000000000000000, 0.9238795325112869605, 1.000000000000000000, 0.9238795325112869605, 1.000000000000000000, 0.9238795325112869605, 1.000000000000000000, 0.9238795325112869605, 1.000000000000000000, 0.9238795325112869605, 1.000000000000000000, 0.9238795325112869605, 1.000000000000000000, 0.9238795325112869605, 1.000000000000000000, 0.9238795325112869605, 1.000000000000000000, 0.9238795325112869605, 1.000000000000000000, 0.9238795325112869605, 1.000000000000000000, 0.9238795325112869605, 1.000000000000000000, 0.9238795325112869605, 1.000000000000000000, 0.9238795325112869605, 1.000000000000000000, 0.9238795325112869605, 1.000000000000000000, 0.9238795325112869605, 1.000000000000000000, 0.9238795325112869605, 1.000000000000000000, 0.9238795325112869605, 1.000000000000000000, 0.9238795325112869605, 1.000000000000000000, 0.9238795325112869605, 1.000000000000000000, 0.9238795325112869605, 1.000000000000000000, 0.9238795325112869605, 1.000000000000000000, 0.9238795325112869605, 1.000000000000000000, 0.9238795325112869605, 1.000000000000000000, 0.9238795325112869605, 1.000000000000000000, 0.9238795325112869605, 1.000000000000000000, 0.9238795325112869605, 1.000000000000000000, 0.9238795325112869605, 1.000000000000000000, 0.9238795325112869605, 1.000000000000000000, 0.9238795325112869605, 1.000000000000000000, 0.9238795325112869605, 1.000000000000000000, 0.9238795325112869605, 1.000000000000000000, 0.9238795325112869605, 1.000000000000000000, 0.9238795325112869605, 1.000000000000000000, 0.9238795325112869605, 1.000000000000000000, 0.9238795325112869605, 1.000000000000000000, 0.9238795325112869605, 1.000000000000000000, 0.9238795325112869605, 1.000000000000000000, 0.9238795325112869605, 1.000000000000000000, 0.9238795325112869605, 1.000000000000000000, 0.9238795325112869605, 1.000000000000000000, 0.9238795325112869605, 1.000000000000000000, 0.9238795325112869605, 1.000000000000000000, 0.9238795325112869605, 1.000000000000000000, 0.9238795325112869605, 1.000000000000000000, 0.9238795325112869605, 1.000000000000000000, 0.9238795325112869605, 1.000000000000000000, 0.9238795325112869605, 1.000000000000000000, 0.9238795325112869605, 1.000000000000000000, 0.9238795325112869605, 1.000000000000000000, 0.9238795325112869605, 1.000000000000000000, 0.9238795325112869605, 1.000000000000000000, 0.9238795325112869605, 1.000000000000000000, 0.9238795325112869605, 1.000000000000000000, 0.9238795325112869605, 1.000000000000000000, 0.9238795325112869605, 1.000000000000000000, 0.9238795325112869605, 1.000000000000000000, 0.9238795325112869605, 1.000000000000000000, 0.9238795325112869605, 1.000000000000000000, 0.9238795325112869605, 1.000000000000000000, 0.9238795325112869605, 1.000000000000000000, 0.9238795325112869605, 1.000000000000000000, 0.9238795325112869605, 1.000000000000000000, 0.9238795325112869605, 1.000000000000000000, 0.9238795325112869605, 1.000000000000000000, 0.9238795325112869605, 1.000000000000000000, 0.9238795325112869605, 1.000000000000000000, 0.9238795325112869605, 1.000000000000000000, 0.9238795325112869605, 1.000000000000000000, 0.9238795325112869605, 1.000000000000000000, 0.9238795325112869605, 1.000000000000000000, 0.9238795325112869605, 1.000000000000000000, 0.9238795325112869605, 1.000000000000000000, 0.9238795325112869605, 1.000000000000000000, 0.9238795325112869605, 1.000000000000000000, 0.9238795325112869605, 1.000000000000000000, 0.9238795325112869605, 1.000000000000000000, 0.9238795325112869605, 1.000000000000000000, 0.9238795325112869605, 1.000000000000000000, 0.9238795325112869605, 1.000000000000000000, 0.9238795325112869605, 1.000000000000000000, 0.9238795325112869605, 1.000000000000000000, 0.9238795325112869605, 1.000000000000000000, 0.9238795325112869605, 1.000000000000000000, 0.9238795325112869605, 1.000000000000000000, 0.9238795325112869605, 1.000000000000000000, 0.9238795325112869605, 1.000000000000000000, 0.9238795325112869605, 1.000000000000000000, 0.9238795325112869605, 1.000000000000000000, 0.9238795325112869605, 1.000000000000000000, 0.9238795325112869605, 1.000000000000000000, 0.9238795325112869605, 1.000000000000000000, 0.9238795325112869605, 1.000000000000000000, 0.9238795325112869605, 1.000000000000000000, 0.9238795325112869605, 1.000000000000000000, 0.9238795325112869605, 1.000000000000000000, 0.9238795325112869605, 1.000000000000000000, 0.9238795325112869605, 1.000000000000000000, 0.9238795325112869605, 1.000000000000000000, 0.9238795325112869605, 1.000000000000000000, 0.9238795325112869605, 1.000000000000000000, 0.9238795325112869605, 1.000000000000000000, 0.9238795325112869605, 1.000000000000000000, 0.9238795325112869605, 1.000000000000000000, 0.9238795325112869605, 1.000000000000000000, 0.9238795325112869605, 1.000000000000000000, 0.9238795325112869605, 1.000000000000000000, 0.9238795325112869605, 1.000000000000000000, 0.9238795325112869605, 1.000000000000000000, 0.9238795325112869605, 1.000000000000000000, 0.9238795325112869605, 1.000000000000000000, 0.9238795325112869605, 1.000000000000000000, 0.9238795325112869605, 1.000000000000000000, 0.9238795325112869605, 1.000000000000000000, 0.9238795325112869605, 1.000000000000000000, 0.9238795325112869605, 1.000000000000000000, 0.9238795325112869605, 1.000000000000000000, 0.9238795325112869605, 1.000000000000000000, 0.9238795325112869605, 1.000000000000000000, 0.9238795325112869605, 1.000000000000000000, 0.9238795325112869605, 1.000000000000000000, 0.9238795325112869605, 1.000000000000000000, 0.9238795325112869605, 1.000000000000000000, 0.9238795325112869605, 1.000000000000000000, 0.9238795325112869605, 1.000000000000000000, 0.9238795325112869605, 1.000000000000000000, 0.9238795325112869605, 1.000000000000000000, 0.9238795325112869605, 1.000000000000000000, 0.9238795325112869605, 1.000000000000000000, 0.9238795325112869605, 1.000000000000000000, 0.9238795325112869605, 1.000000000000000000, 0.9238795325112869605, 1.000000000000000000, 0.9238795325112869605, 1.000000000000000000, 0.9238795325112869605, 1.000000000000000000, 0.9238795325112869605, 1.000000000000000000, 0.9238795325112869605, 1.000000000000000000, 0.9238795325112869605, 1.000000000000000000, 0.9238795325112869605, 1.000000000000000000, 0.9238795325112869605, 1.000000000000000000, 0.9238795325112869605, 1.000000000000000000, 0.9238795325112869605, 1.000000000000000000, 0.9238795325112869605, 1.000000000000000000, 0.9238795325112869605, 1.000000000000000000, 0.9238795325112869605, 1.000000000000000000, 0.9238795325112869605, 1.000000000000000000, 0.9238795325112869605, 1.000000000000000000, 0.9238795325112869605, 1.000000000000000000, 0.9238795325112869605, 1.000000000000000000, 0.9238795325112869605, 1.000000000000000000, 0.9238795325112869605, 1.000000000000000000, 0.9238795325112869605, 1.000000000000000000, 0.9238795325112869605, 1.000000000000000000, 0.9238795325112869605, 1.000000000000000000, 0.9238795325112869605, 1.000000000000000000, 0.9238795325112869605, 1.000000000000000000, 0.9238795325112869605, 1.000000000000000000, 0.9238795325112869605, 1.000000000000000000, 0.9238795325112869605, 1.000000000000000000, 0.9238795325112869605, 1.000000000000000000, 0.9238795325112869605, 1.000000000000000000, 0.9238795325112869605, 1.000000000000000000, 0.9238795325112869605, 1.000000000000000000, 0.9238795325112869605, 1.000000000000000000, 0.9238795325112869605, 1.000000000000000000, 0.9238795325112869605, 1.000000000000000000, 0.9238795325112869605, 1.000000000000000000, 0.9238795325112869605, 1.000000000000000000, 0.9238795325112869605, 1.000000000000000000, 0.9238795325112869605, 1.000000000000000000, 0.9238795325112869605, 1.000000000000000000, 0.9238795325112869605, 1.000000000000000000, 0.9238795325112869605, 1.000000000000000000, 0.9238795325112869605, 1.000000000000000000, 0.9238795325112869605, 1.000000000000000000, 0.9238795325112869605, 1.000000000000000000, 0.9238795325112869605, 1.000000000000000000, 0.9238795325112869605, 1.000000000000000000, 0.9238795325112869605, 1.000000000000000000, 0.9238795325112869605, 1.000000000000000000, 0.9238795325112869605, 1.000000000000000000, 0.9238795325112869605, 1.000000000000000000, 0.9238795325112869605, 1.000000000000000000, 0.9238795325112869605, 1.000000000000000000, 0.9238795325112869605, 1.000000000000000000, 0.9238795325112869605, 1.000000000000000000, 0.9238795325112869605, 1.000000000000000000, 0.9238795325112869605, 1.000000000000000000, 0.9238795325112869605, 1.000000000000000000, 0.9238795325112869605, 1.000000000000000000, 0.9238795325112869605, 1.000000000000000000, 0.9238795325112869605, 1.000000000000000000, 0.9238795325112869605, 1.000000000000000000, 0.9238795325112869605, 1.000000000000000000, 0.9238795325112869605, 1.000000000000000000, 0.9238795325112869605, 1.000000000000000000, 0.9238795325112869605, 1.000000000000000000, 0.9238795325112869605, 1.000000000000000000, 0.9238795325112869605, 1.000000000000000000, 0.9238795325112869605, 1.000000000000000000, 0.9238795325112869605, 1.000000000000000000, 0.9238795325112869605, 1.000000000000000000, 0.9238795325112869605, 1.000000000000000000, 0.9238795325112869605, 1.000000000000000000, 0.9238795325112869605, 1.000000000000000000, 0.9238795325112869605, 1.000000000000000000, 0.9238795325112869605, 1.000000000000000000, 0.9238795325112869605, 1.000000000000000000, 0.9238795325112869605, 1.000000000000000000, 0.9238795325112869605, 1.000000000000000000, 0.9238795325112869605, 1.000000000000000000, 0.9238795325112869605, 1.000000000000000000, 0.9238795325112869605, 1.000000000000000000, 0.9238795325112869605, 1.000000000000000000, 0.9238795325112869605, 1.000000000000000000, 0.9238795325112869605, 1.000000000000000000, 0.9238795325112869605, 1.000000000000000000, 0.9238795325112869605, 1.000000000000000000),
 ( 1.000000000000000000, 0.9238795325112869605, 1.000000000000000000, 0.9238795325112869605, 1.000000000000000000, 0.9238795325112869605, 1.000000000000000000, 0.9238795325112869605, 1.000000000000000000, 0.9238795325112869605, 1.000000000000000000, 0.9238795325112869605, 1.000000000000000000, 0.9238795325112869605, 1.000000000000000000, 0.9238795325112869605, 1.000000000000000000, 0.9238795325112869605, 1.000000000000000000, 0.9238795325112869605, 1.000000000000000000, 0.9238795325112869605, 1.000000000000000000, 0.9238795325112869605, 1.000000000000000000, 0.9238795325112869605, 1.000000000000000000, 0.9238795325112869605, 1.000000000000000000, 0.9238795325112869605, 1.000000000000000000, 0.9238795325112869605, 1.000000000000000000, 0.9238795325112869605, 1.000000000000000000, 0.9238795325112869605, 1.000000000000000000, 0.9238795325112869605, 1.000000000000000000, 0.9238795325112869605, 1.000000000000000000, 0.9238795325112869605, 1.000000000000000000, 0.9238795325112869605, 1.000000000000000000, 0.9238795325112869605, 1.000000000000000000, 0.9238795325112869605, 1.000000000000000000, 0.9238795325112869605, 1.000000000000000000, 0.9238795325112869605, 1.000000000000000000, 0.9238795325112869605, 1.000000000000000000, 0.9238795325112869605, 1.000000000000000000, 0.9238795325112869605, 1.000000000000000000, 0.9238795325112869605, 1.000000000000000000, 0.9238795325112869605, 1.000000000000000000, 0.9238795325112869605, 1.000000000000000000, 0.9238795325112869605, 1.000000000000000000, 0.9238795325112869605, 1.000000000000000000, 0.9238795325112869605, 1.000000000000000000, 0.9238795325112869605, 1.000000000000000000, 0.9238795325112869605, 1.000000000000000000, 0.9238795325112869605, 1.000000000000000000, 0.9238795325112869605, 1.000000000000000000, 0.9238795325112869605, 1.000000000000000000, 0.9238795325112869605, 1.000000000000000000, 0.9238795325112869605, 1.000000000000000000, 0.9238795325112869605, 1.000000000000000000, 0.9238795325112869605, 1.000000000000000000, 0.9238795325112869605, 1.000000000000000000, 0.9238795325112869605, 1.000000000000000000, 0.9238795325112869605, 1.000000000000000000, 0.9238795325112869605, 1.000000000000000000, 0.9238795325112869605, 1.000000000000000000, 0.9238795325112869605, 1.000000000000000000, 0.9238795325112869605, 1.000000000000000000, 0.9238795325112869605, 1.000000000000000000, 0.9238795325112869605, 1.000000000000000000, 0.9238795325112869605, 1.000000000000000000, 0.9238795325112869605, 1.000000000000000000, 0.9238795325112869605, 1.000000000000000000, 0.9238795325112869605, 1.000000000000000000, 0.9238795325112869605, 1.000000000000000000, 0.9238795325112869605, 1.000000000000000000, 0.9238795325112869605, 1.000000000000000000, 0.9238795325112869605, 1.000000000000000000, 0.9238795325112869605, 1.000000000000000000, 0.9238795325112869605, 1.000000000000000000, 0.9238795325112869605, 1.000000000000000000, 0.9238795325112869605, 1.000000000000000000, 0.9238795325112869605, 1.000000000000000000, 0.9238795325112869605, 1.000000000000000000, 0.9238795325112869605, 1.000000000000000000, 0.9238795325112869605, 1.000000000000000000, 0.9238795325112869605, 1.000000000000000000, 0.9238795325112869605, 1.000000000000000000, 0.9238795325112869605, 1.000000000000000000, 0.9238795325112869605, 1.000000000000000000, 0.9238795325112869605, 1.000000000000000000, 0.9238795325112869605, 1.000000000000000000, 0.9238795325112869605, 1.000000000000000000, 0.9238795325112869605, 1.000000000000000000, 0.9238795325112869605, 1.000000000000000000, 0.9238795325112869605, 1.000000000000000000, 0.9238795325112869605, 1.000000000000000000, 0.9238795325112869605, 1.000000000000000000, 0.9238795325112869605, 1.000000000000000000, 0.9238795325112869605, 1.000000000000000000, 0.9238795325112869605, 1.000000000000000000, 0.9238795325112869605, 1.000000000000000000, 0.9238795325112869605, 1.000000000000000000, 0.9238795325112869605, 1.000000000000000000, 0.9238795325112869605, 1.000000000000000000, 0.9238795325112869605, 1.000000000000000000, 0.9238795325112869605, 1.000000000000000000, 0.9238795325112869605, 1.000000000000000000, 0.9238795325112869605, 1.000000000000000000, 0.9238795325112869605, 1.000000000000000000, 0.9238795325112869605, 1.000000000000000000, 0.9238795325112869605, 1.000000000000000000, 0.9238795325112869605, 1.000000000000000000, 0.9238795325112869605, 1.000000000000000000, 0.9238795325112869605, 1.000000000000000000, 0.9238795325112869605, 1.000000000000000000, 0.9238795325112869605, 1.000000000000000000, 0.9238795325112869605, 1.000000000000000000, 0.9238795325112869605, 1.000000000000000000, 0.9238795325112869605, 1.000000000000000000, 0.9238795325112869605, 1.000000000000000000, 0.9238795325112869605, 1.000000000000000000, 0.9238795325112869605, 1.000000000000000000, 0.9238795325112869605, 1.000000000000000000, 0.9238795325112869605, 1.000000000000000000, 0.9238795325112869605, 1.000000000000000000, 0.9238795325112869605, 1.000000000000000000, 0.9238795325112869605, 1.000000000000000000, 0.9238795325112869605, 1.000000000000000000, 0.9238795325112869605, 1.000000000000000000, 0.9238795325112869605, 1.000000000000000000, 0.9238795325112869605, 1.000000000000000000, 0.9238795325112869605, 1.000000000000000000, 0.9238795325112869605, 1.000000000000000000, 0.9238795325112869605, 1.000000000000000000, 0.9238795325112869605, 1.000000000000000000, 0.9238795325112869605, 1.000000000000000000, 0.9238795325112869605, 1.000000000000000000, 0.9238795325112869605, 1.000000000000000000, 0.9238795325112869605, 1.000000000000000000, 0.9238795325112869605, 1.000000000000000000, 0.9238795325112869605, 1.000000000000000000, 0.9238795325112869605, 1.000000000000000000, 0.9238795325112869605, 1.000000000000000000, 0.9238795325112869605, 1.000000000000000000, 0.9238795325112869605, 1.000000000000000000, 0.9238795325112869605, 1.000000000000000000, 0.9238795325112869605, 1.000000000000000000, 0.9238795325112869605, 1.000000000000000000, 0.9238795325112869605, 1.000000000000000000, 0.9238795325112869605, 1.000000000000000000, 0.9238795325112869605, 1.000000000000000000, 0.9238795325112869605, 1.000000000000000000, 0.9238795325112869605, 1.000000000000000000, 0.9238795325112869605, 1.000000000000000000, 0.9238795325112869605, 1.000000000000000000, 0.9238795325112869605, 1.000000000000000000, 0.9238795325112869605, 1.000000000000000000, 0.9238795325112869605, 1.000000000000000000, 0.9238795325112869605, 1.000000000000000000, 0.9238795325112869605, 1.000000000000000000, 0.9238795325112869605, 1.000000000000000000, 0.9238795325112869605, 1.000000000000000000, 0.9238795325112869605, 1.000000000000000000, 0.9238795325112869605, 1.000000000000000000, 0.9238795325112869605, 1.000000000000000000, 0.9238795325112869605, 1.000000000000000000, 0.9238795325112869605, 1.000000000000000000, 0.9238795325112869605, 1.000000000000000000, 0.9238795325112869605, 1.000000000000000000, 0.9238795325112869605, 1.000000000000000000, 0.9238795325112869605, 1.000000000000000000, 0.9238795325112869605, 1.000000000000000000, 0.9238795325112869605, 1.000000000000000000, 0.9238795325112869605, 1.000000000000000000, 0.9238795325112869605, 1.000000000000000000, 0.9238795325112869605, 1.000000000000000000, 0.9238795325112869605, 1.000000000000000000, 0.9238795325112869605, 1.000000000000000000, 0.9238795325112869605, 1.000000000000000000, 0.9238795325112869605, 1.000000000000000000, 0.9238795325112869605, 1.000000000000000000, 0.9238795325112869605, 1.000000000000000000, 0.9238795325112869605, 1.000000000000000000, 0.9238795325112869605, 1.000000000000000000, 0.9238795325112869605, 1.000000000000000000, 0.9238795325112869605, 1.000000000000000000, 0.9238795325112869605, 1.000000000000000000, 0.9238795325112869605, 1.000000000000000000, 0.9238795325112869605, 1.000000000000000000, 0.9238795325112869605, 1.000000000000000000, 0.9238795325112869605, 1.000000000000000000, 0.9238795325112869605, 1.000000000000000000, 0.9238795325112869605, 1.000000000000000000, 0.9238795325112869605, 1.000000000000000000, 0.9238795325112869605, 1.000000000000000000, 0.9238795325112869605, 1.000000000000000000, 0.9238795325112869605, 1.000000000000000000, 0.9238795325112869605, 1.000000000000000000, 0.9238795325112869605, 1.000000000000000000, 0.9238795325112869605, 1.000000000000000000, 0.9238795325112869605, 1.000000000000000000, 0.9238795325112869605, 1.000000000000000000, 0.9238795325112869605, 1.000000000000000000, 0.9238795325112869605, 1.000000000000000000, 0.9238795325112869605, 1.000000000000000000, 0.9238795325112869605, 1.000000000000000000, 0.9238795325112869605, 1.000000000000000000, 0.9238795325112869605, 1.000000000000000000, 0.9238795325112869605, 1.000000000000000000, 0.9238795325112869605, 1.000000000000000000, 0.9238795325112869605, 1.000000000000000000, 0.9238795325112869605, 1.000000000000000000, 0.9238795325112869605, 1.000000000000000000, 0.9238795325112869605, 1.000000000000000000, 0.9238795325112869605, 1.000000000000000000, 0.9238795325112869605, 1.000000000000000000, 0.9238795325112869605, 1.000000000000000000, 0.9238795325112869605, 1.000000000000000000, 0.9238795325112869605, 1.000000000000000000, 0.9238795325112869605, 1.000000000000000000, 0.9238795325112869605, 1.000000000000000000, 0.9238795325112869605, 1.000000000000000000, 0.9238795325112869605, 1.000000000000000000, 0.9238795325112869605, 1.000000000000000000, 0.9238795325112869605, 1.000000000000000000, 0.9238795325112869605, 1.000000000000000000, 0.9238795325112869605, 1.000000000000000000, 0.9238795325112869605, 1.000000000000000000, 0.9238795325112869605, 1.000000000000000000, 0.9238795325112869605, 1.000000000000000000, 0.9238795325112869605, 1.000000000000000000, 0.9238795325112869605, 1.000000000000000000, 0.9238795325112869605, 1.000000000000000000, 0.9238795325112869605, 1.000000000000000000, 0.9238795325112869605, 1.000000000000000000, 0.9238795325112869605, 1.000000000000000000, 0.9238795325112869605, 1.000000000000000000, 0.9238795325112869605, 1.000000000000000000, 0.9238795325112869605, 1.000000000000000000, 0.9238795325112869605, 1.000000000000000000, 0.9238795325112869605, 1.000000000000000000, 0.9238795325112869605, 1.000000000000000000, 0.9238795325112869605, 1.000000000000000000, 0.9238795325112869605, 1.000000000000000000, 0.9238795325112869605, 1.000000000000000000, 0.9238795325112869605, 1.000000000000000000, 0.9238795325112869605, 1.000000000000000000, 0.9238795325112869605, 1.000000000000000000, 0.9238795325112869605, 1.000000000000000000, 0.9238795325112869605, 1.000000000000000000, 0.9238795325112869605, 1.000000000000000000, 0.9238795325112869605, 1.000000000000000000, 0.9238795325112869605, 1.000000000000000000, 0.9238795325112869605, 1.000000000000000000, 0.9238795325112869605, 1.000000000000000000, 0.9238795325112869605, 1.000000000000000000, 0.9238795325112869605, 1.000000000000000000, 0.9238795325112869605, 1.000000000000000000, 0.9238795325112869605, 1.000000000000000000, 0.9238795325112869605, 1.000000000000000000, 0.9238795325112869605, 1.000000000000000000, 0.9238795325112869605, 1.000000000000000000, 0.9238795325112869605, 1.000000000000000000, 0.9238795325112869605, 1.000000000000000000, 0.9238795325112869605, 1.000000000000000000, 0.9238795325112869605, 1.000000000000000000, 0.9238795325112869605, 1.000000000000000000, 0.9238795325112869605, 1.000000000000000000, 0.9238795325112869605, 1.000000000000000000, 0.9238795325112869605, 1.000000000000000000, 0.9238795325112869605, 1.000000000000000000, 0.9238795325112869605, 1.000000000000000000, 0.9238795325112869605, 1.000000000000000000, 0.9238795325112869605, 1.000000000000000000, 0.9238795325112869605, 1.000000000000000000, 0.9238795325112869605, 1.000000000000000000, 0.9238795325112869605, 1.000000000000000000, 0.9238795325112869605, 1.000000000000000000, 0.9238795325112869605, 1.000000000000000000, 0.9238795325112869605, 1.000000000000000000, 0.9238795325112869605, 1.000000000000000000, 0.9238795325112869605, 1.000000000000000000, 0.9238795325112869605, 1.000000000000000000, 0.9238795325112869605, 1.000000000000000000, 0.9238795325112869605, 1.000000000000000000, 0.9238795325112869605, 1.000000000000000000, 0.9238795325112869605, 1.000000000000000000, 0.9238795325112869605, 1.000000000000000000, 0.9238795325112869605, 1.000000000000000000, 0.9238795325112869605, 1.000000000000000000, 0.9238795325112869605, 1.000000000000000000, 0.9238795325112869605, 1.000000000000000000, 0.9238795325112869605, 1.000000000000000000, 0.9238795325112869605, 1.000000000000000000, 0.9238795325112869605, 1.000000000000000000, 0.9238795325112869605, 1.000000000000000000, 0.9238795325112869605, 1.000000000000000000, 0.9238795325112869605, 1.000000000000000000, 0.9238795325112869605, 1.000000000000000000, 0.9238795325112869605, 1.000000000000000000, 0.9238795325112869605, 1.000000000000000000, 0.9238795325112869605, 1.000000000000000000, 0.9238795325112869605, 1.000000000000000000, 0.9238795325112869605, 1.000000000000000000, 0.9238795325112869605, 1.000000000000000000, 0.9238795325112869605, 1.000000000000000000, 0.9238795325112869605, 1.000000000000000000, 0.9238795325112869605, 1.000000000000000000, 0.9238795325112869605, 1.000000000000000000, 0.9238795325112869605, 1.000000000000000000, 0.9238795325112869605, 1.000000000000000000, 0.9238795325112869605, 1.000000000000000000, 0.9238795325112869605, 1.000000000000000000, 0.9238795325112869605, 1.000000000000000000, 0.9238795325112869605, 1.000000000000000000, 0.9238795325112869605, 1.000000000000000000, 0.9238795325112869605, 1.000000000000000000, 0.9238795325112869605, 1.000000000000000000, 0.9238795325112869605, 1.000000000000000000, 0.9238795325112869605, 1.000000000000000000, 0.9238795325112869605, 1.000000000000000000, 0.9238795325112869605, 1.000000000000000000, 0.9238795325112869605, 1.000000000000000000, 0.9238795325112869605, 1.000000000000000000, 0.9238795325112869605, 1.000000000000000000, 0.9238795325112869605, 1.000000000000000000, 0.9238795325112869605, 1.000000000000000000, 0.9238795325112869605, 1.000000000000000000, 0.9238795325112869605, 1.000000000000000000, 0.9238795325112869605, 1.000000000000000000, 0.9238795325112869605, 1.000000000000000000, 0.9238795325112869605, 1.000000000000000000, 0.9238795325112869605, 1.000000000000000000, 0.9238795325112869605, 1.000000000000000000, 0.9238795325112869605, 1.000000000000000000, 0.9238795325112869605, 1.000000000000000000, 0.9238795325112869605, 1.000000000000000000, 0.9238795325112869605, 1.000000000000000000, 0.9238795325112869605, 1.000000000000000000, 0.9238795325112869605, 1.000000000000000000, 0.9238795325112869605, 1.000000000000000000, 0.9238795325112869605, 1.000000000000000000, 0.9238795325112869605, 1.000000000000000000, 0.9238795325112869605, 1.000000000000000000, 0.9238795325112869605, 1.000000000000000000, 0.9238795325112869605, 1.000000000000000000, 0.9238795325112869605, 1.000000000000000000, 0.9238795325112869605, 1.000000000000000000, 0.9238795325112869605, 1.000000000000000000, 0.9238795325112869605, 1.000000000000000000, 0.9238795325112869605, 1.000000000000000000, 0.9238795325112869605, 1.000000000000000000, 0.9238795325112869605, 1.000000000000000000, 0.9238795325112869605, 1.000000000000000000, 0.9238795325112869605, 1.000000000000000000, 0.9238795325112869605, 1.000000000000000000, 0.9238795325112869605, 1.000000000000000000, 0.9238795325112869605, 1.000000000000000000, 0.9238795325112869605, 1.000000000000000000, 0.9238795325112869605, 1.000000000000000000, 0.9238795325112869605, 1.000000000000000000, 0.9238795325112869605, 1.000000000000000000, 0.9238795325112869605, 1.000000000000000000, 0.9238795325112869605, 1.000000000000000000, 0.9238795325112869605, 1.000000000000000000, 0.9238795325112869605, 1.000000000000000000, 0.9238795325112869605, 1.000000000000000000, 0.9238795325112869605, 1.000000000000000000, 0.9238795325112869605, 1.000000000000000000, 0.9238795325112869605, 1.000000000000000000, 0.9238795325112869605, 1.000000000000000000, 0.9238795325112869605, 1.000000000000000000, 0.9238795325112869605, 1.000000000000000000, 0.9238795325112869605, 1.000000000000000000, 0.9238795325112869605, 1.000000000000000000, 0.9238795325112869605, 1.000000000000000000, 0.9238795325112869605, 1.000000000000000000, 0.9238795325112869605, 1.000000000000000000, 0.9238795325112869605, 1.000000000000000000, 0.9238795325112869605, 1.000000000000000000, 0.9238795325112869605, 1.000000000000000000, 0.9238795325112869605, 1.000000000000000000, 0.9238795325112869605, 1.000000000000000000, 0.9238795325112869605, 1.000000000000000000, 0.9238795325112869605, 1.000000000000000000, 0.9238795325112869605, 1.000000000000000000, 0.9238795325112869605, 1.000000000000000000, 0.9238795325112869605, 1.000000000000000000, 0.9238795325112869605, 1.000000000000000000, 0.9238795325112869605, 1.000000000000000000, 0.9238795325112869605, 1.000000000000000000, 0.9238795325112869605, 1.000000000000000000, 0.9238795325112869605, 1.000000000000000000, 0.9238795325112869605, 1.000000000000000000, 0.9238795325112869605, 1.000000000000000000, 0.9238795325112869605, 1.000000000000000000, 0.9238795325112869605, 1.000000000000000000, 0.9238795325112869605, 1.000000000000000000, 0.9238795325112869605, 1.000000000000000000, 0.9238795325112869605, 1.000000000000000000, 0.9238795325112869605, 1.000000000000000000, 0.9238795325112869605, 1.000000000000000000, 0.9238795325112869605, 1.000000000000000000, 0.9238795325112869605, 1.000000000000000000, 0.9238795325112869605, 1.000000000000000000, 0.9238795325112869605, 1.000000000000000000, 0.9238795325112869605, 1.000000000000000000, 0.9238795325112869605, 1.000000000000000000, 0.9238795325112869605, 1.000000000000000000, 0.9238795325112869605, 1.000000000000000000, 0.9238795325112869605, 1.000000000000000000, 0.9238795325112869605, 1.000000000000000000, 0.9238795325112869605, 1.000000000000000000, 0.9238795325112869605, 1.000000000000000000, 0.9238795325112869605, 1.000000000000000000, 0.9238795325112869605, 1.000000000000000000),
 ( 1.000000000000000000, 0.9238795325112869605, 1.000000000000000000, 0.9238795325112869605, 1.000000000000000000, 0.9238795325112869605, 1.000000000000000000, 0.9238795325112869605, 1.000000000000000000, 0.9238795325112869605, 1.000000000000000000, 0.9238795325112869605, 1.000000000000000000, 0.9238795325112869605, 1.000000000000000000, 0.9238795325112869605, 1.000000000000000000, 0.9238795325112869605, 1.000000000000000000, 0.9238795325112869605, 1.000000000000000000, 0.9238795325112869605, 1.000000000000000000, 0.9238795325112869605, 1.000000000000000000, 0.9238795325112869605, 1.000000000000000000, 0.9238795325112869605, 1.000000000000000000, 0.9238795325112869605, 1.000000000000000000, 0.9238795325112869605, 1.000000000000000000, 0.9238795325112869605, 1.000000000000000000, 0.9238795325112869605, 1.000000000000000000, 0.9238795325112869605, 1.000000000000000000, 0.9238795325112869605, 1.000000000000000000, 0.9238795325112869605, 1.000000000000000000, 0.9238795325112869605, 1.000000000000000000, 0.9238795325112869605, 1.000000000000000000, 0.9238795325112869605, 1.000000000000000000, 0.9238795325112869605, 1.000000000000000000, 0.9238795325112869605, 1.000000000000000000, 0.9238795325112869605, 1.000000000000000000, 0.9238795325112869605, 1.000000000000000000, 0.9238795325112869605, 1.000000000000000000, 0.9238795325112869605, 1.000000000000000000, 0.9238795325112869605, 1.000000000000000000, 0.9238795325112869605, 1.000000000000000000, 0.9238795325112869605, 1.000000000000000000, 0.9238795325112869605, 1.000000000000000000, 0.9238795325112869605, 1.000000000000000000, 0.9238795325112869605, 1.000000000000000000, 0.9238795325112869605, 1.000000000000000000, 0.9238795325112869605, 1.000000000000000000, 0.9238795325112869605, 1.000000000000000000, 0.9238795325112869605, 1.000000000000000000, 0.9238795325112869605, 1.000000000000000000, 0.9238795325112869605, 1.000000000000000000, 0.9238795325112869605, 1.000000000000000000, 0.9238795325112869605, 1.000000000000000000, 0.9238795325112869605, 1.000000000000000000, 0.9238795325112869605, 1.000000000000000000, 0.9238795325112869605, 1.000000000000000000, 0.9238795325112869605, 1.000000000000000000, 0.9238795325112869605, 1.000000000000000000, 0.9238795325112869605, 1.000000000000000000, 0.9238795325112869605, 1.000000000000000000, 0.9238795325112869605, 1.000000000000000000, 0.9238795325112869605, 1.000000000000000000, 0.9238795325112869605, 1.000000000000000000, 0.9238795325112869605, 1.000000000000000000, 0.9238795325112869605, 1.000000000000000000, 0.9238795325112869605, 1.000000000000000000, 0.9238795325112869605, 1.000000000000000000, 0.9238795325112869605, 1.000000000000000000, 0.9238795325112869605, 1.000000000000000000, 0.9238795325112869605, 1.000000000000000000, 0.9238795325112869605, 1.000000000000000000, 0.9238795325112869605, 1.000000000000000000, 0.9238795325112869605, 1.000000000000000000, 0.9238795325112869605, 1.000000000000000000, 0.9238795325112869605, 1.000000000000000000, 0.9238795325112869605, 1.000000000000000000, 0.9238795325112869605, 1.000000000000000000, 0.9238795325112869605, 1.000000000000000000, 0.9238795325112869605, 1.000000000000000000, 0.9238795325112869605, 1.000000000000000000, 0.9238795325112869605, 1.000000000000000000, 0.9238795325112869605, 1.000000000000000000, 0.9238795325112869605, 1.000000000000000000, 0.9238795325112869605, 1.000000000000000000, 0.9238795325112869605, 1.000000000000000000, 0.9238795325112869605, 1.000000000000000000, 0.9238795325112869605, 1.000000000000000000, 0.9238795325112869605, 1.000000000000000000, 0.9238795325112869605, 1.000000000000000000, 0.9238795325112869605, 1.000000000000000000, 0.9238795325112869605, 1.000000000000000000, 0.9238795325112869605, 1.000000000000000000, 0.9238795325112869605, 1.000000000000000000, 0.9238795325112869605, 1.000000000000000000, 0.9238795325112869605, 1.000000000000000000, 0.9238795325112869605, 1.000000000000000000, 0.9238795325112869605, 1.000000000000000000, 0.9238795325112869605, 1.000000000000000000, 0.9238795325112869605, 1.000000000000000000, 0.9238795325112869605, 1.000000000000000000, 0.9238795325112869605, 1.000000000000000000, 0.9238795325112869605, 1.000000000000000000, 0.9238795325112869605, 1.000000000000000000, 0.9238795325112869605, 1.000000000000000000, 0.9238795325112869605, 1.000000000000000000, 0.9238795325112869605, 1.000000000000000000, 0.9238795325112869605, 1.000000000000000000, 0.9238795325112869605, 1.000000000000000000, 0.9238795325112869605, 1.000000000000000000, 0.9238795325112869605, 1.000000000000000000, 0.9238795325112869605, 1.000000000000000000, 0.9238795325112869605, 1.000000000000000000, 0.9238795325112869605, 1.000000000000000000, 0.9238795325112869605, 1.000000000000000000, 0.9238795325112869605, 1.000000000000000000, 0.9238795325112869605, 1.000000000000000000, 0.9238795325112869605, 1.000000000000000000, 0.9238795325112869605, 1.000000000000000000, 0.9238795325112869605, 1.000000000000000000, 0.9238795325112869605, 1.000000000000000000, 0.9238795325112869605, 1.000000000000000000, 0.9238795325112869605, 1.000000000000000000, 0.9238795325112869605, 1.000000000000000000, 0.9238795325112869605, 1.000000000000000000, 0.9238795325112869605, 1.000000000000000000, 0.9238795325112869605, 1.000000000000000000, 0.9238795325112869605, 1.000000000000000000, 0.9238795325112869605, 1.000000000000000000, 0.9238795325112869605, 1.000000000000000000, 0.9238795325112869605, 1.000000000000000000, 0.9238795325112869605, 1.000000000000000000, 0.9238795325112869605, 1.000000000000000000, 0.9238795325112869605, 1.000000000000000000, 0.9238795325112869605, 1.000000000000000000, 0.9238795325112869605, 1.000000000000000000, 0.9238795325112869605, 1.000000000000000000, 0.9238795325112869605, 1.000000000000000000, 0.9238795325112869605, 1.000000000000000000, 0.9238795325112869605, 1.000000000000000000, 0.9238795325112869605, 1.000000000000000000, 0.9238795325112869605, 1.000000000000000000, 0.9238795325112869605, 1.000000000000000000, 0.9238795325112869605, 1.000000000000000000, 0.9238795325112869605, 1.000000000000000000, 0.9238795325112869605, 1.000000000000000000, 0.9238795325112869605, 1.000000000000000000, 0.9238795325112869605, 1.000000000000000000, 0.9238795325112869605, 1.000000000000000000, 0.9238795325112869605, 1.000000000000000000, 0.9238795325112869605, 1.000000000000000000, 0.9238795325112869605, 1.000000000000000000, 0.9238795325112869605, 1.000000000000000000, 0.9238795325112869605, 1.000000000000000000, 0.9238795325112869605, 1.000000000000000000, 0.9238795325112869605, 1.000000000000000000, 0.9238795325112869605, 1.000000000000000000, 0.9238795325112869605, 1.000000000000000000, 0.9238795325112869605, 1.000000000000000000, 0.9238795325112869605, 1.000000000000000000, 0.9238795325112869605, 1.000000000000000000, 0.9238795325112869605, 1.000000000000000000, 0.9238795325112869605, 1.000000000000000000, 0.9238795325112869605, 1.000000000000000000, 0.9238795325112869605, 1.000000000000000000, 0.9238795325112869605, 1.000000000000000000, 0.9238795325112869605, 1.000000000000000000, 0.9238795325112869605, 1.000000000000000000, 0.9238795325112869605, 1.000000000000000000, 0.9238795325112869605, 1.000000000000000000, 0.9238795325112869605, 1.000000000000000000, 0.9238795325112869605, 1.000000000000000000, 0.9238795325112869605, 1.000000000000000000, 0.9238795325112869605, 1.000000000000000000, 0.9238795325112869605, 1.000000000000000000, 0.9238795325112869605, 1.000000000000000000, 0.9238795325112869605, 1.000000000000000000, 0.9238795325112869605, 1.000000000000000000, 0.9238795325112869605, 1.000000000000000000, 0.9238795325112869605, 1.000000000000000000, 0.9238795325112869605, 1.000000000000000000, 0.9238795325112869605, 1.000000000000000000, 0.9238795325112869605, 1.000000000000000000, 0.9238795325112869605, 1.000000000000000000, 0.9238795325112869605, 1.000000000000000000, 0.9238795325112869605, 1.000000000000000000, 0.9238795325112869605, 1.000000000000000000, 0.9238795325112869605, 1.000000000000000000, 0.9238795325112869605, 1.000000000000000000, 0.9238795325112869605, 1.000000000000000000, 0.9238795325112869605, 1.000000000000000000, 0.9238795325112869605, 1.000000000000000000, 0.9238795325112869605, 1.000000000000000000, 0.9238795325112869605, 1.000000000000000000, 0.9238795325112869605, 1.000000000000000000, 0.9238795325112869605, 1.000000000000000000, 0.9238795325112869605, 1.000000000000000000, 0.9238795325112869605, 1.000000000000000000, 0.9238795325112869605, 1.000000000000000000, 0.9238795325112869605, 1.000000000000000000, 0.9238795325112869605, 1.000000000000000000, 0.9238795325112869605, 1.000000000000000000, 0.9238795325112869605, 1.000000000000000000, 0.9238795325112869605, 1.000000000000000000, 0.9238795325112869605, 1.000000000000000000, 0.9238795325112869605, 1.000000000000000000, 0.9238795325112869605, 1.000000000000000000, 0.9238795325112869605, 1.000000000000000000, 0.9238795325112869605, 1.000000000000000000, 0.9238795325112869605, 1.000000000000000000, 0.9238795325112869605, 1.000000000000000000, 0.9238795325112869605, 1.000000000000000000, 0.9238795325112869605, 1.000000000000000000, 0.9238795325112869605, 1.000000000000000000, 0.9238795325112869605, 1.000000000000000000, 0.9238795325112869605, 1.000000000000000000, 0.9238795325112869605, 1.000000000000000000, 0.9238795325112869605, 1.000000000000000000, 0.9238795325112869605, 1.000000000000000000, 0.9238795325112869605, 1.000000000000000000, 0.9238795325112869605, 1.000000000000000000, 0.9238795325112869605, 1.000000000000000000, 0.9238795325112869605, 1.000000000000000000, 0.9238795325112869605, 1.000000000000000000, 0.9238795325112869605, 1.000000000000000000, 0.9238795325112869605, 1.000000000000000000, 0.9238795325112869605, 1.000000000000000000, 0.9238795325112869605, 1.000000000000000000, 0.9238795325112869605, 1.000000000000000000, 0.9238795325112869605, 1.000000000000000000, 0.9238795325112869605, 1.000000000000000000, 0.9238795325112869605, 1.000000000000000000, 0.9238795325112869605, 1.000000000000000000, 0.9238795325112869605, 1.000000000000000000, 0.9238795325112869605, 1.000000000000000000, 0.9238795325112869605, 1.000000000000000000, 0.9238795325112869605, 1.000000000000000000, 0.9238795325112869605, 1.000000000000000000, 0.9238795325112869605, 1.000000000000000000, 0.9238795325112869605, 1.000000000000000000, 0.9238795325112869605, 1.000000000000000000, 0.9238795325112869605, 1.000000000000000000, 0.9238795325112869605, 1.000000000000000000, 0.9238795325112869605, 1.000000000000000000, 0.9238795325112869605, 1.000000000000000000, 0.9238795325112869605, 1.000000000000000000, 0.9238795325112869605, 1.000000000000000000, 0.9238795325112869605, 1.000000000000000000, 0.9238795325112869605, 1.000000000000000000, 0.9238795325112869605, 1.000000000000000000, 0.9238795325112869605, 1.000000000000000000, 0.9238795325112869605, 1.000000000000000000, 0.9238795325112869605, 1.000000000000000000, 0.9238795325112869605, 1.000000000000000000, 0.9238795325112869605, 1.000000000000000000, 0.9238795325112869605, 1.000000000000000000, 0.9238795325112869605, 1.000000000000000000, 0.9238795325112869605, 1.000000000000000000, 0.9238795325112869605, 1.000000000000000000, 0.9238795325112869605, 1.000000000000000000, 0.9238795325112869605, 1.000000000000000000, 0.9238795325112869605, 1.000000000000000000, 0.9238795325112869605, 1.000000000000000000, 0.9238795325112869605, 1.000000000000000000, 0.9238795325112869605, 1.000000000000000000, 0.9238795325112869605, 1.000000000000000000, 0.9238795325112869605, 1.000000000000000000, 0.9238795325112869605, 1.000000000000000000, 0.9238795325112869605, 1.000000000000000000, 0.9238795325112869605, 1.000000000000000000, 0.9238795325112869605, 1.000000000000000000, 0.9238795325112869605, 1.000000000000000000, 0.9238795325112869605, 1.000000000000000000, 0.9238795325112869605, 1.000000000000000000, 0.9238795325112869605, 1.000000000000000000, 0.9238795325112869605, 1.000000000000000000, 0.9238795325112869605, 1.000000000000000000, 0.9238795325112869605, 1.000000000000000000, 0.9238795325112869605, 1.000000000000000000, 0.9238795325112869605, 1.000000000000000000, 0.9238795325112869605, 1.000000000000000000, 0.9238795325112869605, 1.000000000000000000, 0.9238795325112869605, 1.000000000000000000, 0.9238795325112869605, 1.000000000000000000, 0.9238795325112869605, 1.000000000000000000, 0.9238795325112869605, 1.000000000000000000, 0.9238795325112869605, 1.000000000000000000, 0.9238795325112869605, 1.000000000000000000, 0.9238795325112869605, 1.000000000000000000, 0.9238795325112869605, 1.000000000000000000, 0.9238795325112869605, 1.000000000000000000, 0.9238795325112869605, 1.000000000000000000, 0.9238795325112869605, 1.000000000000000000, 0.9238795325112869605, 1.000000000000000000, 0.9238795325112869605, 1.000000000000000000, 0.9238795325112869605, 1.000000000000000000, 0.9238795325112869605, 1.000000000000000000, 0.9238795325112869605, 1.000000000000000000, 0.9238795325112869605, 1.000000000000000000, 0.9238795325112869605, 1.000000000000000000, 0.9238795325112869605, 1.000000000000000000, 0.9238795325112869605, 1.000000000000000000, 0.9238795325112869605, 1.000000000000000000, 0.9238795325112869605, 1.000000000000000000, 0.9238795325112869605, 1.000000000000000000, 0.9238795325112869605, 1.000000000000000000, 0.9238795325112869605, 1.000000000000000000, 0.9238795325112869605, 1.000000000000000000, 0.9238795325112869605, 1.000000000000000000, 0.9238795325112869605, 1.000000000000000000, 0.9238795325112869605, 1.000000000000000000, 0.9238795325112869605, 1.000000000000000000, 0.9238795325112869605, 1.000000000000000000, 0.9238795325112869605, 1.000000000000000000, 0.9238795325112869605, 1.000000000000000000, 0.9238795325112869605, 1.000000000000000000, 0.9238795325112869605, 1.000000000000000000, 0.9238795325112869605, 1.000000000000000000, 0.9238795325112869605, 1.000000000000000000, 0.9238795325112869605, 1.000000000000000000, 0.9238795325112869605, 1.000000000000000000, 0.9238795325112869605, 1.000000000000000000, 0.9238795325112869605, 1.000000000000000000, 0.9238795325112869605, 1.000000000000000000, 0.9238795325112869605, 1.000000000000000000, 0.9238795325112869605, 1.000000000000000000, 0.9238795325112869605, 1.000000000000000000, 0.9238795325112869605, 1.000000000000000000, 0.9238795325112869605, 1.000000000000000000, 0.9238795325112869605, 1.000000000000000000, 0.9238795325112869605, 1.000000000000000000, 0.9238795325112869605, 1.000000000000000000, 0.9238795325112869605, 1.000000000000000000, 0.9238795325112869605, 1.000000000000000000, 0.9238795325112869605, 1.000000000000000000, 0.9238795325112869605, 1.000000000000000000, 0.9238795325112869605, 1.000000000000000000, 0.9238795325112869605, 1.000000000000000000, 0.9238795325112869605, 1.000000000000000000, 0.9238795325112869605, 1.000000000000000000, 0.9238795325112869605, 1.000000000000000000, 0.9238795325112869605, 1.000000000000000000, 0.9238795325112869605, 1.000000000000000000, 0.9238795325112869605, 1.000000000000000000, 0.9238795325112869605, 1.000000000000000000, 0.9238795325112869605, 1.000000000000000000, 0.9238795325112869605, 1.000000000000000000, 0.9238795325112869605, 1.000000000000000000, 0.9238795325112869605, 1.000000000000000000, 0.9238795325112869605, 1.000000000000000000, 0.9238795325112869605, 1.000000000000000000, 0.9238795325112869605, 1.000000000000000000, 0.9238795325112869605, 1.000000000000000000, 0.9238795325112869605, 1.000000000000000000, 0.9238795325112869605, 1.000000000000000000, 0.9238795325112869605, 1.000000000000000000, 0.9238795325112869605, 1.000000000000000000, 0.9238795325112869605, 1.000000000000000000, 0.9238795325112869605, 1.000000000000000000, 0.9238795325112869605, 1.000000000000000000, 0.9238795325112869605, 1.000000000000000000, 0.9238795325112869605, 1.000000000000000000, 0.9238795325112869605, 1.000000000000000000, 0.9238795325112869605, 1.000000000000000000, 0.9238795325112869605, 1.000000000000000000, 0.9238795325112869605, 1.000000000000000000, 0.9238795325112869605, 1.000000000000000000, 0.9238795325112869605, 1.000000000000000000, 0.9238795325112869605, 1.000000000000000000, 0.9238795325112869605, 1.000000000000000000, 0.9238795325112869605, 1.000000000000000000, 0.9238795325112869605, 1.000000000000000000, 0.9238795325112869605, 1.000000000000000000, 0.9238795325112869605, 1.000000000000000000, 0.9238795325112869605, 1.000000000000000000, 0.9238795325112869605, 1.000000000000000000, 0.9238795325112869605, 1.000000000000000000, 0.9238795325112869605, 1.000000000000000000, 0.9238795325112869605, 1.000000000000000000, 0.9238795325112869605, 1.000000000000000000, 0.9238795325112869605, 1.000000000000000000, 0.9238795325112869605, 1.000000000000000000, 0.9238795325112869605, 1.000000000000000000, 0.9238795325112869605, 1.000000000000000000, 0.9238795325112869605, 1.000000000000000000, 0.9238795325112869605, 1.000000000000000000, 0.9238795325112869605, 1.000000000000000000, 0.9238795325112869605, 1.000000000000000000, 0.9238795325112869605, 1.000000000000000000, 0.9238795325112869605, 1.000000000000000000, 0.9238795325112869605, 1.000000000000000000, 0.9238795325112869605, 1.000000000000000000, 0.9238795325112869605, 1.000000000000000000, 0.9238795325112869605, 1.000000000000000000, 0.9238795325112869605, 1.000000000000000000, 0.9238795325112869605, 1.000000000000000000, 0.9238795325112869605, 1.000000000000000000, 0.9238795325112869605, 1.000000000000000000, 0.9238795325112869605, 1.000000000000000000, 0.9238795325112869605, 1.000000000000000000, 0.9238795325112869605, 1.000000000000000000, 0.9238795325112869605, 1.000000000000000000, 0.9238795325112869605, 1.000000000000000000, 0.9238795325112869605, 1.000000000000000000, 0.9238795325112869605, 1.000000000000000000, 0.9238795325112869605, 1.000000000000000000, 0.9238795325112869605, 1.000000000000000000, 0.9238795325112869605, 1.000000000000000000, 0.9238795325112869605, 1.000000000000000000, 0.9238795325112869605, 1.000000000000000000) ) ) 
 REPRESENTATION_ITEM ( '' )  SURFACE ( )  ) ;
#11430=CARTESIAN_POINT ( 'NONE',  ( -1.100456976456230270E-17, -1.034492628480683019, -0.1797182628040039365 ) ) ;
#11443=CARTESIAN_POINT ( 'NONE',  ( 0.1787899950787401604, -0.7706692912848194243, 0.07405724077823318263 ) ) ;
#11449=CARTESIAN_POINT ( 'NONE',  ( -0.1574803149606299191, -1.602362204724409489, 0.000000000000000000 ) ) ;
#11462=CARTESIAN_POINT ( 'NONE',  ( -0.1787899950787401604, -0.3288641257095537562, 0.07405724077823318263 ) ) ;
#11463=B_SPLINE_CURVE_WITH_KNOTS ( 'NONE', 3,
 ( #3280, #36374, #10255, #28727, #6399, #17902, #43296, #32552, #3531, #28969, #43769, #21256, #24860, #35880, #20782, #10011, #17664, #47140, #43526, #42795, #39932, #7121, #32312, #10496, #25094, #6871, #10742, #21743 ),
 .UNSPECIFIED., .F., .F.,
 ( 4, 2, 2, 2, 2, 2, 2, 2, 2, 2, 2, 2, 2, 4 ),
 ( 0.000000000000000000, 0.001273870958249984650, 0.001910806437374976867, 0.002547741916499968867, 0.003184677395624961084, 0.003821612874749952433, 0.004458548353874944650, 0.005095483832999936867, 0.005732419312124930819, 0.006369354791249923903, 0.007006290270374916987, 0.007643225749499910938, 0.008917096707749896239, 0.01019096766599988241 ),
 .UNSPECIFIED. ) ;
#11464=CARTESIAN_POINT ( 'NONE',  ( -0.02294826503924878025, -0.08955989818537933578, 0.2205244489207712766 ) ) ;
#11465=FACE_OUTER_BOUND ( 'NONE', #16662, .T. ) ;
#11472=CARTESIAN_POINT ( 'NONE',  ( 0.07405724077823318263, -1.331692913332063855, 0.1787899950787401604 ) ) ;
#11474=CARTESIAN_POINT ( 'NONE',  ( -0.1787899950787401604, -1.538385826717890703, -0.07405724077823318263 ) ) ;
#11483=CARTESIAN_POINT ( 'NONE',  ( -0.06523048226347956391, -0.2563976377952757457, 0.1574803149606297803 ) ) ;
#11488=CARTESIAN_POINT ( 'NONE',  ( -0.1233909491491453209, -0.09102144875556358872, -0.1293981901162606918 ) ) ;
#11492=CARTESIAN_POINT ( 'NONE',  ( -0.1574803149606299191, -0.5688976376877488139, 0.000000000000000000 ) ) ;
#11495=CARTESIAN_POINT ( 'NONE',  ( -0.1697971239859669412, -0.08954441352768210960, -0.01236366681777519710 ) ) ;
#11502=CARTESIAN_POINT ( 'NONE',  ( -0.1787899950787401882, -1.614665354276944909, 0.000000000000000000 ) ) ;
#11503=CARTESIAN_POINT ( 'NONE',  ( -1.094772975963752103E-17, -0.6845472440407243120, -0.1787899950787401882 ) ) ;
#11504=CARTESIAN_POINT ( 'NONE',  ( -9.642888182262618425E-18, -1.218503937007874072, -0.1574803149606299191 ) ) ;
#11529=CARTESIAN_POINT ( 'NONE',  ( 0.1110659630103943002, -0.09851382545259528001, 0.09590396427280079017 ) ) ;
#11534=CARTESIAN_POINT ( 'NONE',  ( -0.07405724077823318263, -0.8395669290800948925, -0.1787899950787401604 ) ) ;
#11535=CARTESIAN_POINT ( 'NONE',  ( 0.1787899950787401604, -0.4606299212060784853, 0.07405724077823318263 ) ) ;
#11536=CARTESIAN_POINT ( 'NONE',  ( 0.07405724077823318263, -0.9970472440407247561, -0.1787899950787401604 ) ) ;
#11541=CARTESIAN_POINT ( 'NONE',  ( -0.07444174185955065859, -0.3086068017090296545, 0.1797182628040039087 ) ) ;
#11542=CARTESIAN_POINT ( 'NONE',  ( 0.1113553986120547346, 0.1545275590551181133, -0.1113553986120547346 ) ) ;
#11545=CARTESIAN_POINT ( 'NONE',  ( 3.284318927891251994E-17, -0.03494094482812622193, 0.1787899950787401882 ) ) ;
#11550=PRESENTATION_STYLE_ASSIGNMENT (( #4316 ) ) ;
#11552=CARTESIAN_POINT ( 'NONE',  ( 0.000000000000000000, 0.09842519685039370636, 0.000000000000000000 ) ) ;
#11558=CARTESIAN_POINT ( 'NONE',  ( 0.07405724077823318263, -0.2293307086076536994, 0.1787899950787401604 ) ) ;
#11561=CARTESIAN_POINT ( 'NONE',  ( 3.284318927891251994E-17, -1.171751968450173154, 0.1787899950787401882 ) ) ;
#11571=CARTESIAN_POINT ( 'NONE',  ( -0.1247969209625214848, -0.09842895638388027280, -0.1280391975408537442 ) ) ;
#11585=AXIS2_PLACEMENT_3D ( 'NONE', #27024, #36839, #23170 ) ;
#11589=CARTESIAN_POINT ( 'NONE',  ( 0.1787899950787401604, -1.534572787126878390, 0.07405724077823318263 ) ) ;
#11591=CARTESIAN_POINT ( 'NONE',  ( -0.07405724077823318263, -0.5049212597887556830, 0.1787899950787401604 ) ) ;
#11592=EDGE_CURVE ( 'NONE', #43256, #1072, #45563, .T. ) ;
#11604=CARTESIAN_POINT ( 'NONE',  ( -0.1787899950787401882, 0.1017461105109186970, 0.000000000000000000 ) ) ;
#11605=CARTESIAN_POINT ( 'NONE',  ( 0.1264236179284866091, -1.678641732229700922, 0.1264236179284866091 ) ) ;
#11610=CARTESIAN_POINT ( 'NONE',  ( 0.1113553986120547346, -0.5246062992125984925, 0.1113553986120547346 ) ) ;
#11612=CARTESIAN_POINT ( 'NONE',  ( 0.1797182628040039087, -1.396205226905880226, -0.07444174185955065859 ) ) ;
#11613=DIRECTION ( 'NONE',  ( 0.000000000000000000, 0.000000000000000000, 1.000000000000000000 ) ) ;
#11621=CARTESIAN_POINT ( 'NONE',  ( 0.1574803149606299191, -0.8248031494987716483, -1.928577636452523993E-17 ) ) ;
#11622=CARTESIAN_POINT ( 'NONE',  ( 0.1787899950787401604, 0.1299212598962831977, 0.07405724077823318263 ) ) ;
#11634=CARTESIAN_POINT ( 'NONE',  ( 0.1797182628040039087, 0.01619634789726941138, 0.07444174185955046430 ) ) ;
#11635=CARTESIAN_POINT ( 'NONE',  ( 0.07405724077823318263, -1.252952755851747924, 0.1787899950787401604 ) ) ;
#11642=CARTESIAN_POINT ( 'NONE',  ( -0.07405724077823318263, -0.1505905511273389341, 0.1787899950787401604 ) ) ;
#11646=CARTESIAN_POINT ( 'NONE',  ( -0.04509681258129859954, -0.07057211410339614410, 0.2593943580756443712 ) ) ;
#11649=CARTESIAN_POINT ( 'NONE',  ( -0.1574803149606300301, -0.09891732272711858953, -0.06523048226347956391 ) ) ;
#11659=CARTESIAN_POINT ( 'NONE',  ( -0.07405724077823318263, -0.9144940469693966234, 0.1787899950787401604 ) ) ;
#11661=FACE_OUTER_BOUND ( 'NONE', #28548, .T. ) ;
#11672=CARTESIAN_POINT ( 'NONE',  ( 0.07444174185955046430, -0.9975831796617853353, -0.1797182628040039087 ) ) ;
#11681=CARTESIAN_POINT ( 'NONE',  ( -0.1574803149606299191, -0.6870078739082204899, 0.000000000000000000 ) ) ;
#11685=CARTESIAN_POINT ( 'NONE',  ( 0.1787899950787401882, -0.8469488188438739629, -2.189545951927503898E-17 ) ) ;
#11692=CARTESIAN_POINT ( 'NONE',  ( -0.1113553986120547346, -1.607283464566929165, -0.1113553986120547346 ) ) ;
#11709=CARTESIAN_POINT ( 'NONE',  ( 0.07405724077823318263, -0.5946121572056172200, 0.1787899950787401604 ) ) ;
#11710=CARTESIAN_POINT ( 'NONE',  ( -0.1256064272821220407, -0.08955963219184016888, -0.2158613615193716861 ) ) ;
#11711=CARTESIAN_POINT ( 'NONE',  ( 0.1574803149606300301, 0.04379921270595223126, -0.06523048226347956391 ) ) ;
#11717=( BOUNDED_CURVE ( )  B_SPLINE_CURVE ( 2, ( #17429, #46187, #31372, #9311, #16965, #23934, #38995, #35429, #6402 ),
 .UNSPECIFIED., .F., .T. ) 
 B_SPLINE_CURVE_WITH_KNOTS ( ( 3, 2, 2, 2, 3 ),
 ( 0.02500000000000000139, 0.02750000000000000014, 0.02999999999999999889, 0.03250000000000000111, 0.03500000000000000333 ),
 .UNSPECIFIED. ) 
 CURVE ( )  GEOMETRIC_REPRESENTATION_ITEM ( )  RATIONAL_B_SPLINE_CURVE ( ( 1.000000000000000000, 0.9238795325112869605, 1.000000000000000000, 0.9238795325112869605, 1.000000000000000000, 0.9238795325112869605, 1.000000000000000000, 0.9238795325112869605, 1.000000000000000000 ) ) 
 REPRESENTATION_ITEM ( '' )  ) ;
#11718=CARTESIAN_POINT ( 'NONE',  ( 0.1787899950787401882, -1.768332629646561127, -2.189545951927503898E-17 ) ) ;
#11721=CARTESIAN_POINT ( 'NONE',  ( 0.2471922436403682921, -0.09120620265198671472, 0.04599440333040333284 ) ) ;
#11725=CARTESIAN_POINT ( 'NONE',  ( 3.284318927891251994E-17, -1.334153543253322916, 0.1787899950787401882 ) ) ;
#11726=CARTESIAN_POINT ( 'NONE',  ( 0.1264236179284866091, -1.521161417269070837, 0.1264236179284866091 ) ) ;
#11736=VERTEX_POINT ( 'NONE', #32142 ) ;
#11742=CARTESIAN_POINT ( 'NONE',  ( -0.1066054788070368298, -0.08956136665047831347, 0.1197104361589552413 ) ) ;
#11749=CARTESIAN_POINT ( 'NONE',  ( -0.07405724077823318263, -1.622047244040725866, -0.1787899950787401604 ) ) ;
#11750=CARTESIAN_POINT ( 'NONE',  ( -0.1787899950787401604, -0.7165354330171036512, -0.07405724077823318263 ) ) ;
#11751=CARTESIAN_POINT ( 'NONE',  ( 0.1113553986120547346, -1.144685039370078705, -0.1113553986120547346 ) ) ;
#11776=CARTESIAN_POINT ( 'NONE',  ( 0.02596600997328759458, -0.09851382729582973397, 0.1524084879473496246 ) ) ;
#11784=CARTESIAN_POINT ( 'NONE',  ( 0.1787899950787401882, -0.8518700786863936392, -2.189545951927503898E-17 ) ) ;
#11785=CARTESIAN_POINT ( 'NONE',  ( -0.1264236179284866091, -1.019192913332062966, 0.1264236179284866091 ) ) ;
#11789=CARTESIAN_POINT ( 'NONE',  ( 0.1797182628040039087, -0.2987642820239903574, 0.07444174185955046430 ) ) ;
#11790=CARTESIAN_POINT ( 'NONE',  ( -9.642888182262618425E-18, 0.1200787401574803237, -0.1574803149606299191 ) ) ;
#11801=CARTESIAN_POINT ( 'NONE',  ( -0.1787899950787401882, -0.2810039369541106336, 0.000000000000000000 ) ) ;
#11803=CARTESIAN_POINT ( 'NONE',  ( 0.1787899950787401882, -1.201279527505291433, -2.189545951927503898E-17 ) ) ;
#11812=CARTESIAN_POINT ( 'NONE',  ( -0.1198507064121036164, -0.09842530151305696473, -0.1326724740186921714 ) ) ;
#11820=CARTESIAN_POINT ( 'NONE',  ( -0.2183449438721881963, -0.09851385166753484635, -0.1145859995850722346 ) ) ;
#11826=CARTESIAN_POINT ( 'NONE',  ( 0.1787899950787401604, -1.450911369804040785, -0.07405724077823318263 ) ) ;
#11829=CARTESIAN_POINT ( 'NONE',  ( -0.07405724077823318263, -0.4015748030958427028, -0.1787899950787401604 ) ) ;
#11834=CARTESIAN_POINT ( 'NONE',  ( 0.1787899950787401604, -0.2244094487651340231, 0.07405724077823318263 ) ) ;
#11836=CARTESIAN_POINT ( 'NONE',  ( -0.1787899950787401882, 0.1411161892510761906, 0.000000000000000000 ) ) ;
#11837=CARTESIAN_POINT ( 'NONE',  ( 0.1264236179284866091, -1.708169291284818980, -0.1264236179284866091 ) ) ;
#11842=CARTESIAN_POINT ( 'NONE',  ( -9.642888182262618425E-18, -0.7854330708661416693, -0.1574803149606299191 ) ) ;
#11844=CARTESIAN_POINT ( 'NONE',  ( -0.07444174185955065859, -1.450339085173596443, 0.1797182628040039087 ) ) ;
#11846=CARTESIAN_POINT ( 'NONE',  ( 0.2471922904502826812, 0.08571147543118957934, -0.06121067491484653150 ) ) ;
#11854=CARTESIAN_POINT ( 'NONE',  ( -0.1113553986120547346, -0.8395669290263306772, 0.1113553986120547346 ) ) ;
#11866=CARTESIAN_POINT ( 'NONE',  ( -0.1797182628040039365, -0.07976821903186437357, 0.000000000000000000 ) ) ;
#11867=CARTESIAN_POINT ( 'NONE',  ( 0.1787899950787401604, -1.208661417269070393, 0.07405724077823318263 ) ) ;
#11876=CARTESIAN_POINT ( 'NONE',  ( 3.284318927891251994E-17, -0.1874999999462366451, 0.1787899950787401882 ) ) ;
#11879=CARTESIAN_POINT ( 'NONE',  ( -0.1574803149606299191, 0.09055118110236221041, 0.000000000000000000 ) ) ;
#11882=CARTESIAN_POINT ( 'NONE',  ( -0.1113553986120547346, -0.06200787390822106587, -0.1113553986120547346 ) ) ;
#11888=DIRECTION ( 'NONE',  ( 0.000000000000000000, 0.000000000000000000, 1.000000000000000000 ) ) ;
#11892=CARTESIAN_POINT ( 'NONE',  ( 0.1787899950787401882, -0.9809310548434114763, -2.189545951927503898E-17 ) ) ;
#11904=CARTESIAN_POINT ( 'NONE',  ( 0.1797182628040039087, -1.002504439504306344, -0.07444174185955065859 ) ) ;
#11915=CARTESIAN_POINT ( 'NONE',  ( 0.1574803149606300301, -0.7091535431995588112, 0.06523048226347956391 ) ) ;
#11919=CARTESIAN_POINT ( 'NONE',  ( 0.1787899950787401604, -0.7657480314423001921, -0.07405724077823318263 ) ) ;
#11931=CARTESIAN_POINT ( 'NONE',  ( 2.892866454678787531E-17, -1.750000000000000222, 0.1574803149606299191 ) ) ;
#11939=CARTESIAN_POINT ( 'NONE',  ( -0.1787899950787401604, -1.503937007820251637, -0.07405724077823318263 ) ) ;
#11948=CARTESIAN_POINT ( 'NONE',  ( -0.1264236179284866091, -0.5724664879142778995, -0.1264236179284866091 ) ) ;
#11949=CARTESIAN_POINT ( 'NONE',  ( -0.09248453076245886917, -0.08955999818690787984, 0.2055509654934188912 ) ) ;
#11962=CARTESIAN_POINT ( 'NONE',  ( -0.07405724077823318263, -1.390748031442299082, -0.1787899950787401604 ) ) ;
#11963=CARTESIAN_POINT ( 'NONE',  ( -0.07405724077823318263, -1.528543307032852239, 0.1787899950787401604 ) ) ;
#11970=CARTESIAN_POINT ( 'NONE',  ( 2.892866454678787531E-17, -0.3326771653543306728, 0.1574803149606299191 ) ) ;
#11979=CARTESIAN_POINT ( 'NONE',  ( -0.1376518243080670778, -0.08956097154447616171, 0.08777079064950775444 ) ) ;
#11985=CARTESIAN_POINT ( 'NONE',  ( -1.094772975963752103E-17, -1.506397637741511586, -0.1787899950787401882 ) ) ;
#11986=CARTESIAN_POINT ( 'NONE',  ( -0.1264236179284866091, -0.8272637794737952577, 0.1264236179284866091 ) ) ;
#11987=CARTESIAN_POINT ( 'NONE',  ( 0.1574803149606299191, -1.228346456692913424, -1.928577636452523993E-17 ) ) ;
#12004=CARTESIAN_POINT ( 'NONE',  ( 0.1093692153654458876, 0.09774221684002680488, 0.2222887249338434679 ) ) ;
#12010=CARTESIAN_POINT ( 'NONE',  ( -0.1598411944706594756, -0.09842519685039370636, 0.1688112090790881981 ) ) ;
#12016=CARTESIAN_POINT ( 'NONE',  ( 0.1264236179284866091, -0.9355314960092283583, 0.1264236179284866091 ) ) ;
#12018=CARTESIAN_POINT ( 'NONE',  ( -0.1787899950787401882, -1.024114173174582643, 0.000000000000000000 ) ) ;
#12021=CARTESIAN_POINT ( 'NONE',  ( -0.1797182628040039365, -0.3553587702129669124, 0.000000000000000000 ) ) ;
#12028=CARTESIAN_POINT ( 'NONE',  ( -8.354793841626791791E-17, -0.09842519685039370636, -0.2854330708661417804 ) ) ;
#12035=DIRECTION ( 'NONE',  ( 1.224646799147351482E-16, 0.000000000000000000, -1.000000000000000000 ) ) ;
#12036=CARTESIAN_POINT ( 'NONE',  ( -0.1264236179284866091, -0.4040354330171023745, -0.1264236179284866091 ) ) ;
#12038=CARTESIAN_POINT ( 'NONE',  ( -0.1264236179284866091, -1.304625984198204636, -0.1264236179284866091 ) ) ;
#12045=CARTESIAN_POINT ( 'NONE',  ( -0.1113553986120547346, -1.193897637687748148, 0.1113553986120547346 ) ) ;
#12049=CARTESIAN_POINT ( 'NONE',  ( 0.03943478969741477658, -0.09842516626972255822, -0.1743868110616672018 ) ) ;
#12063=CARTESIAN_POINT ( 'NONE',  ( -0.1787899950787401604, -1.391856251693805779, 0.07405724077823318263 ) ) ;
#12065=CARTESIAN_POINT ( 'NONE',  ( -0.07405724077823318263, -0.4409448818359998357, -0.1787899950787401604 ) ) ;
#12073=CARTESIAN_POINT ( 'NONE',  ( -0.07405724077823318263, -1.769685039316315267, 0.1787899950787401604 ) ) ;
#12074=CARTESIAN_POINT ( 'NONE',  ( -0.1787899950787401604, 0.1102362205262043815, -0.07405724077823318263 ) ) ;
#12081=CARTESIAN_POINT ( 'NONE',  ( 0.1113553986120547346, -0.6820866141732283561, 0.1113553986120547346 ) ) ;
#12083=CARTESIAN_POINT ( 'NONE',  ( 0.1270800023317771588, -1.433114675724777465, -0.1270800023317771588 ) ) ;
#12084=CARTESIAN_POINT ( 'NONE',  ( -0.06523048226347956391, -0.06446850382948084157, -0.1574803149606300301 ) ) ;
#12094=CARTESIAN_POINT ( 'NONE',  ( -0.1264236179284866091, 0.07824803154982658271, 0.1264236179284866091 ) ) ;
#12105=ORIENTED_EDGE ( 'NONE', *, *, #476, .T. ) ;
#12106=CARTESIAN_POINT ( 'NONE',  ( 3.301370929368692659E-17, 0.008814458133489902134, 0.1797182628040039365 ) ) ;
#12107=CARTESIAN_POINT ( 'NONE',  ( -0.1787899950787401604, -1.228346456639149542, -0.07405724077823318263 ) ) ;
#12120=CARTESIAN_POINT ( 'NONE',  ( -9.642888182262618425E-18, -0.02755905501058318954, -0.1574803149606299191 ) ) ;
#12127=CARTESIAN_POINT ( 'NONE',  ( -0.1264236179284866091, -0.9661672753158523363, -0.1264236179284866091 ) ) ;
#12129=CARTESIAN_POINT ( 'NONE',  ( -0.1787899950787401882, 0.03887795280966901967, 0.000000000000000000 ) ) ;
#12139=DIRECTION ( 'NONE',  ( 0.000000000000000000, 0.000000000000000000, 1.000000000000000000 ) ) ;
#12140=CARTESIAN_POINT ( 'NONE',  ( 0.1797182628040039365, -0.9262249119452500290, -2.200913952912460540E-17 ) ) ;
#12149=CARTESIAN_POINT ( 'NONE',  ( -0.1264236179284866091, 0.07332677170730689253, -0.1264236179284866091 ) ) ;
#12154=CARTESIAN_POINT ( 'NONE',  ( 0.1264236179284866091, -0.9207677164816693294, -0.1264236179284866091 ) ) ;
#12157=CARTESIAN_POINT ( 'NONE',  ( -0.1574803149606300301, -1.752460629813732185, -0.06523048226347956391 ) ) ;
#12161=CARTESIAN_POINT ( 'NONE',  ( -0.1574803149606300301, -1.683562992125984259, -0.06523048226347956391 ) ) ;
#12167=CARTESIAN_POINT ( 'NONE',  ( -9.642888182262618425E-18, -0.3425196849318429826, -0.1574803149606299191 ) ) ;
#12168=CARTESIAN_POINT ( 'NONE',  ( -0.1787899950787401882, -1.462106299158834721, 0.000000000000000000 ) ) ;
#12176=CARTESIAN_POINT ( 'NONE',  ( -0.1787899950787401604, -0.5650845981504987181, 0.07405724077823318263 ) ) ;
#12177=CARTESIAN_POINT ( 'NONE',  ( -0.1574815732576543281, -0.08955969983079922758, 0.1660848416297525665 ) ) ;
#12178=CARTESIAN_POINT ( 'NONE',  ( 0.06523048226347956391, 0.03395669302091284397, 0.1574803149606297803 ) ) ;
#12181=FACE_OUTER_BOUND ( 'NONE', #24547, .T. ) ;
#12187=CARTESIAN_POINT ( 'NONE',  ( -0.07405724077823318263, -1.297244094434425010, 0.1787899950787401604 ) ) ;
#12188=CARTESIAN_POINT ( 'NONE',  ( 0.1787899950787401604, -1.513779527505292322, -0.07405724077823318263 ) ) ;
#12196=CARTESIAN_POINT ( 'NONE',  ( 0.1574803149606300301, -0.3203740157480316486, -0.06523048226347956391 ) ) ;
#12206=CARTESIAN_POINT ( 'NONE',  ( -0.1113553986120547346, -0.5344488187901101917, -0.1113553986120547346 ) ) ;
#12207=ADVANCED_FACE ( 'NONE', ( #30933 ), #35103, .T. ) ;
#12210=CARTESIAN_POINT ( 'NONE',  ( -0.1353283724619816497, -0.08956113309537444556, 0.09080182561100422212 ) ) ;
#12218=CARTESIAN_POINT ( 'NONE',  ( 0.1787899950787401882, -1.673720472387181024, -2.189545951927503898E-17 ) ) ;
#12219=CARTESIAN_POINT ( 'NONE',  ( 0.1787899950787401882, -0.8518700786863936392, -2.189545951927503898E-17 ) ) ;
#12220=CARTESIAN_POINT ( 'NONE',  ( 0.1574803149606300301, -1.186515748031495843, -0.06523048226347956391 ) ) ;
#12228=CARTESIAN_POINT ( 'NONE',  ( 0.1574803149606300301, -1.373523621939715555, -0.06523048226347956391 ) ) ;
#12244=CARTESIAN_POINT ( 'NONE',  ( -0.2423422045102378020, -0.09842519685039370636, -0.009343655355443130847 ) ) ;
#12252=APPLICATION_CONTEXT ( 'automotive_design' ) ;
#12254=CARTESIAN_POINT ( 'NONE',  ( 0.07405724077823318263, -0.8198818897100156322, 0.1787899950787401604 ) ) ;
#12255=CARTESIAN_POINT ( 'NONE',  ( -1.094772975963752103E-17, -1.112696850339937038, -0.1787899950787401882 ) ) ;
#12257=CARTESIAN_POINT ( 'NONE',  ( -0.07444174185955065859, -0.3479768804491872314, 0.1797182628040039087 ) ) ;
#12258=CARTESIAN_POINT ( 'NONE',  ( 0.06523048226347956391, 0.1569881889763779237, -0.1574803149606300301 ) ) ;
#12267=CARTESIAN_POINT ( 'NONE',  ( 0.1113553986120547346, -0.9872047243019212992, 0.1113553986120547346 ) ) ;
#12268=CARTESIAN_POINT ( 'NONE',  ( -0.1787899950787401604, -0.3572834645131658382, 0.07405724077823318263 ) ) ;
#12272=CARTESIAN_POINT ( 'NONE',  ( -0.07405724077823318263, -1.174212598371433769, 0.1787899950787401604 ) ) ;
#12284=CARTESIAN_POINT ( 'NONE',  ( 0.06167052456099836322, -0.09842519458604685745, -0.1678199136211908638 ) ) ;
#12302=CARTESIAN_POINT ( 'NONE',  ( 0.1264236179284866091, -1.418923180827663444, 0.1264236179284866091 ) ) ;
#12305=CARTESIAN_POINT ( 'NONE',  ( -0.1264236179284866091, -0.4286417322297008115, 0.1264236179284866091 ) ) ;
#12311=AXIS2_PLACEMENT_3D ( 'NONE', #40869, #12404, #41105 ) ;
#12318=CARTESIAN_POINT ( 'NONE',  ( 0.1787899950787401604, 0.1238917798022573097, -0.07405724077823318263 ) ) ;
#12319=CARTESIAN_POINT ( 'NONE',  ( -0.1264236179284866091, 0.1077755906049446960, -0.1264236179284866091 ) ) ;
#12324=CARTESIAN_POINT ( 'NONE',  ( -0.1574803149606299191, -0.7362204724409449064, 0.000000000000000000 ) ) ;
#12326=CARTESIAN_POINT ( 'NONE',  ( 0.1270800023317771588, -1.629965069425564961, -0.1270800023317771588 ) ) ;
#12328=CARTESIAN_POINT ( 'NONE',  ( 0.1574803149606300301, -0.4680118109160952278, -0.06523048226347956391 ) ) ;
#12337=CARTESIAN_POINT ( 'NONE',  ( 0.1264236179284866091, 0.08809055123486594918, 0.1264236179284866091 ) ) ;
#12343=ORIENTED_EDGE ( 'NONE', *, *, #2059, .F. ) ;
#12360=CARTESIAN_POINT ( 'NONE',  ( -0.05730322896416230327, -0.07836638817768154519, -0.2523490388730016964 ) ) ;
#12365=CARTESIAN_POINT ( 'NONE',  ( 0.06523048226347956391, -0.04478346445940203924, 0.1574803149606297803 ) ) ;
#12370=CARTESIAN_POINT ( 'NONE',  ( 0.1264236179284866091, -1.025222393426088452, 0.1264236179284866091 ) ) ;
#12372=CARTESIAN_POINT ( 'NONE',  ( 0.1787899950787401882, -0.02017716530056720692, -2.189545951927503898E-17 ) ) ;
#12381=CARTESIAN_POINT ( 'NONE',  ( -0.1264236179284866091, -0.5910433070328504623, 0.1264236179284866091 ) ) ;
#12387=CARTESIAN_POINT ( 'NONE',  ( -0.1797182628040039365, -1.182130423756273752, 0.000000000000000000 ) ) ;
#12397=CARTESIAN_POINT ( 'NONE',  ( 0.1264236179284866091, 0.05364173233722803469, 0.1264236179284866091 ) ) ;
#12401=CARTESIAN_POINT ( 'NONE',  ( -0.07405724077823318263, -0.9921259841982054128, -0.1787899950787401604 ) ) ;
#12404=DIRECTION ( 'NONE',  ( -0.000000000000000000, 1.000000000000000000, 0.000000000000000000 ) ) ;
#12406=CARTESIAN_POINT ( 'NONE',  ( 2.892866454678787531E-17, -1.661417322727118062, 0.1574803149606299191 ) ) ;
#12409=CARTESIAN_POINT ( 'NONE',  ( -1.094772975963752103E-17, -0.08907480309584270284, -0.1787899950787401882 ) ) ;
#12418=CARTESIAN_POINT ( 'NONE',  ( 2.892866454678787531E-17, -0.3622047243019216878, 0.1574803149606299191 ) ) ;
#12419=CARTESIAN_POINT ( 'NONE',  ( -0.07405724077823318263, -1.533464566875370805, 0.1787899950787401604 ) ) ;
#12426=CARTESIAN_POINT ( 'NONE',  ( -0.1264236179284866091, -0.5232538894890811365, 0.1264236179284866091 ) ) ;
#12427=CARTESIAN_POINT ( 'NONE',  ( -0.1681363471019937106, -0.08956127397141554203, -0.03619664881022559288 ) ) ;
#12433=CARTESIAN_POINT ( 'NONE',  ( 3.284318927891251994E-17, -1.817545228071759889, 0.1787899950787401882 ) ) ;
#12435=CARTESIAN_POINT ( 'NONE',  ( 0.1787899950787401604, -1.562992125930488196, 0.07405724077823318263 ) ) ;
#12436=CARTESIAN_POINT ( 'NONE',  ( -0.1264236179284866091, -1.609744094434425232, 0.1264236179284866091 ) ) ;
#12446=CARTESIAN_POINT ( 'NONE',  ( 0.06523048226347956391, -0.4483267716535432879, 0.1574803149606297803 ) ) ;
#12461=CARTESIAN_POINT ( 'NONE',  ( -0.1065407853927636261, -0.08956136429197258941, 0.1197608106671575745 ) ) ;
#12462=CARTESIAN_POINT ( 'NONE',  ( -0.1787899950787401604, -0.5147637794737950356, -0.07405724077823318263 ) ) ;
#12468=CARTESIAN_POINT ( 'NONE',  ( -0.1787899950787401882, -1.772145669237574994, 0.000000000000000000 ) ) ;
#12469=CARTESIAN_POINT ( 'NONE',  ( -1.094772975963752103E-17, -0.9601377952218268508, -0.1787899950787401882 ) ) ;
#12470=CARTESIAN_POINT ( 'NONE',  ( -0.1574803149606297803, -1.363681102362204856, 0.06523048226347956391 ) ) ;
#12478=CARTESIAN_POINT ( 'NONE',  ( -0.1113553986120547346, -1.351377952648377789, 0.1113553986120547346 ) ) ;
#12492=CARTESIAN_POINT ( 'NONE',  ( -0.1189708289958600340, -0.09851383554566003897, 0.1141074950210181072 ) ) ;
#12499=CARTESIAN_POINT ( 'NONE',  ( 0.1264236179284866091, -0.9749015747493857686, 0.1264236179284866091 ) ) ;
#12500=CARTESIAN_POINT ( 'NONE',  ( 0.07405724077823318263, -1.075787401521038689, -0.1787899950787401604 ) ) ;
#12504=CARTESIAN_POINT ( 'NONE',  ( -0.07444174185955065859, -0.4021107387169037817, -0.1797182628040039087 ) ) ;
#12506=CARTESIAN_POINT ( 'NONE',  ( -0.1574803149606299191, 0.01181102362204724393, 0.000000000000000000 ) ) ;
#12509=CIRCLE ( 'NONE', #46925, 0.2471922904502826812 ) ;
#12514=PRODUCT_DEFINITION_FORMATION_WITH_SPECIFIED_SOURCE ( 'ANY', '', #5156, .NOT_KNOWN. ) ;
#12518=CARTESIAN_POINT ( 'NONE',  ( -1.094772975963752103E-17, -0.4483267715997795166, -0.1787899950787401882 ) ) ;
#12520=CARTESIAN_POINT ( 'NONE',  ( -0.1264236179284866091, -1.255413385773007873, 0.1264236179284866091 ) ) ;
#12532=CARTESIAN_POINT ( 'NONE',  ( -0.1480151140659365927, -0.09843327264853890535, -0.1007363786963137303 ) ) ;
#12547=CARTESIAN_POINT ( 'NONE',  ( 0.1264236179284866091, -1.645301133583568998, -0.1264236179284866091 ) ) ;
#12550=CARTESIAN_POINT ( 'NONE',  ( 0.1787899950787401604, -0.4507874015210400209, -0.07405724077823318263 ) ) ;
#12552=B_SPLINE_CURVE_WITH_KNOTS ( 'NONE', 3,
 ( #6604, #27973, #28932, #43495, #6361, #46855, #6834, #9745, #20975, #2297, #39426, #2764, #35623, #42761, #13800, #2997, #32028, #43009, #20747, #10218 ),
 .UNSPECIFIED., .F., .F.,
 ( 4, 1, 1, 1, 1, 1, 2, 2, 1, 1, 1, 2, 2, 4 ),
 ( 0.000000000000000000, 0.2499999999999903411, 0.3749999999999857891, 0.4374999999999835132, 0.4687499999999825695, 0.4843749999999820699, 0.4921874999999819034, 0.4999999999999817923, 0.6249999999999863443, 0.6874999999999884537, 0.7187499999999895639, 0.7343749999999904521, 0.7499999999999914513, 1.000000000000000000 ),
 .UNSPECIFIED. ) ;
#12553=DIRECTION ( 'NONE',  ( 0.000000000000000000, 1.000000000000000000, 0.000000000000000000 ) ) ;
#12556=CARTESIAN_POINT ( 'NONE',  ( -0.1787899950787401882, -1.737696850339937038, 0.000000000000000000 ) ) ;
#12562=CARTESIAN_POINT ( 'NONE',  ( -0.06523048226347956391, -0.7829724409448810540, -0.1574803149606300301 ) ) ;
#12564=CARTESIAN_POINT ( 'NONE',  ( 0.1270800023317771588, -1.551224911945249918, -0.1270800023317771588 ) ) ;
#12566=LINE ( 'NONE', #15445, #23059 ) ;
#12570=DIRECTION ( 'NONE',  ( 0.000000000000000000, 1.000000000000000000, 0.000000000000000000 ) ) ;
#12575=CARTESIAN_POINT ( 'NONE',  ( -0.1787899950787401604, 0.03149606304588949135, -0.07405724077823318263 ) ) ;
#12590=CARTESIAN_POINT ( 'NONE',  ( 0.1574803149606300301, -1.097933070758615903, -0.06523048226347956391 ) ) ;
#12591=CARTESIAN_POINT ( 'NONE',  ( -0.1264236179284866091, -1.388287401521039355, -0.1264236179284866091 ) ) ;
#12596=CARTESIAN_POINT ( 'NONE',  ( -9.642888182262618425E-18, 0.04133858267716535029, -0.1574803149606299191 ) ) ;
#12603=CARTESIAN_POINT ( 'NONE',  ( -0.1036066153428575193, -0.09660391682274853398, -0.2256134787374337036 ) ) ;
#12606=CARTESIAN_POINT ( 'NONE',  ( -0.1574803149606299191, -0.01771653532554381960, 0.000000000000000000 ) ) ;
#12610=CARTESIAN_POINT ( 'NONE',  ( 0.07405724077823318263, -1.052289322559947449, -0.1787899950787401604 ) ) ;
#12612=CARTESIAN_POINT ( 'NONE',  ( 0.1787899950787401604, 0.05610236225848785896, 0.07405724077823318263 ) ) ;
#12620=AXIS2_PLACEMENT_3D ( 'NONE', #45352, #23568, #41497 ) ;
#12621=CARTESIAN_POINT ( 'NONE',  ( 0.07405724077823318263, -0.6624015747493856576, 0.1787899950787401604 ) ) ;
#12624=CARTESIAN_POINT ( 'NONE',  ( 0.1797182628040039087, -1.164906014307455884, 0.07444174185955046430 ) ) ;
#12625=CARTESIAN_POINT ( 'NONE',  ( 0.1690594283350484173, 0.1299212598425197318, -0.03640762741699016952 ) ) ;
#12642=CARTESIAN_POINT ( 'NONE',  ( 0.1574803149606300301, -1.732775590443652591, 0.06523048226347956391 ) ) ;
#12648=CARTESIAN_POINT ( 'NONE',  ( -0.1787899950787401604, 0.1200787402112438867, 0.07405724077823318263 ) ) ;
#12652=CARTESIAN_POINT ( 'NONE',  ( -0.009906661468957165401, 0.04209688371799823886, 0.2797134572002688002 ) ) ;
#12655=CARTESIAN_POINT ( 'NONE',  ( -0.1787899950787401882, -1.540846456639149542, 0.000000000000000000 ) ) ;
#12665=CARTESIAN_POINT ( 'NONE',  ( 0.1264236179284866091, -0.5527814485441993053, 0.1264236179284866091 ) ) ;
#12666=CARTESIAN_POINT ( 'NONE',  ( -0.03915270915796512097, -0.08956085038011968313, -0.1800528347341008029 ) ) ;
#12674=CARTESIAN_POINT ( 'NONE',  ( 0.07405724077823318263, -1.449803149552535642, 0.1787899950787401604 ) ) ;
#12679=CARTESIAN_POINT ( 'NONE',  ( 0.07444174185955065859, -0.6580162505279267826, 0.1797182628040039087 ) ) ;
#12686=CARTESIAN_POINT ( 'NONE',  ( -0.06523048226347956391, -0.4532480314960634082, 0.1574803149606297803 ) ) ;
#12700=CARTESIAN_POINT ( 'NONE',  ( 0.1264236179284866091, -0.4975393700249764461, 0.1264236179284866091 ) ) ;
#12709=CARTESIAN_POINT ( 'NONE',  ( -0.07405724077823318263, -1.661417322780881500, -0.1787899950787401604 ) ) ;
#12710=CARTESIAN_POINT ( 'NONE',  ( -1.094772975963752103E-17, -0.9207677164816693294, -0.1787899950787401882 ) ) ;
#12711=CARTESIAN_POINT ( 'NONE',  ( 0.06523048226347956391, -1.432578740157480324, 0.1574803149606297803 ) ) ;
#12729=CARTESIAN_POINT ( 'NONE',  ( 0.1352415222742598400, -0.09842519685039370636, -0.1450469393348480240 ) ) ;
#12735=CARTESIAN_POINT ( 'NONE',  ( 0.1264236179284866091, -1.053641732229700700, 0.1264236179284866091 ) ) ;
#12736=CARTESIAN_POINT ( 'NONE',  ( -0.07405724077823318263, -1.252952755851747924, 0.1787899950787401604 ) ) ;
#12740=CARTESIAN_POINT ( 'NONE',  ( -0.1797182628040039087, -0.4759296363546985376, -0.07444174185955065859 ) ) ;
#12742=CARTESIAN_POINT ( 'NONE',  ( 0.1574803149606300301, -0.04478346456692917921, -0.06523048226347956391 ) ) ;
#12743=CARTESIAN_POINT ( 'NONE',  ( 0.07405724077823318263, -0.1358267715997797664, -0.1787899950787401604 ) ) ;
#12753=CARTESIAN_POINT ( 'NONE',  ( 0.1787899950787401604, -0.3769685038832444324, -0.07405724077823318263 ) ) ;
#12754=CARTESIAN_POINT ( 'NONE',  ( -0.07405724077823318263, -1.449803149552535642, 0.1787899950787401604 ) ) ;
#12771=CARTESIAN_POINT ( 'NONE',  ( -0.1920024521149243935, -0.09851385062432203854, 0.1351331792528293330 ) ) ;
#12775=CARTESIAN_POINT ( 'NONE',  ( 0.07405724077823318263, -1.657604283189869632, 0.1787899950787401604 ) ) ;
#12778=CARTESIAN_POINT ( 'NONE',  ( -0.1787899950787401604, -0.6328740156942683770, -0.07405724077823318263 ) ) ;
#12784=CARTESIAN_POINT ( 'NONE',  ( -0.1264236179284866091, -0.2367125983714334636, 0.1264236179284866091 ) ) ;
#12789=CARTESIAN_POINT ( 'NONE',  ( -0.1264236179284866091, 0.01808469318808409235, -0.1264236179284866091 ) ) ;
#12790=CARTESIAN_POINT ( 'NONE',  ( -0.1787899950787401604, -1.809055118056471123, 0.07405724077823318263 ) ) ;
#12797=CARTESIAN_POINT ( 'NONE',  ( -9.642888182262618425E-18, -0.9035433070866142335, -0.1574803149606299191 ) ) ;
#12799=CARTESIAN_POINT ( 'NONE',  ( 0.1797182628040039365, -1.595516250527927005, -2.200913952912460540E-17 ) ) ;
#12801=CARTESIAN_POINT ( 'NONE',  ( -0.07405724077823318263, -0.3474409448281265411, 0.1787899950787401604 ) ) ;
#12807=DIRECTION ( 'NONE',  ( 0.000000000000000000, 0.000000000000000000, 1.000000000000000000 ) ) ;
#12812=CARTESIAN_POINT ( 'NONE',  ( -0.1574803149606299191, -0.8444881888688503535, 0.000000000000000000 ) ) ;
#12813=CARTESIAN_POINT ( 'NONE',  ( -0.1264236179284866091, 0.03887795280966901967, 0.1264236179284866091 ) ) ;
#12821=CARTESIAN_POINT ( 'NONE',  ( 0.06523048226347956391, -1.107775590443654146, 0.1574803149606297803 ) ) ;
#12822=CARTESIAN_POINT ( 'NONE',  ( -0.07405724077823318263, -1.375984251914741163, 0.1787899950787401604 ) ) ;
#12833=CARTESIAN_POINT ( 'NONE',  ( 0.1651804164989525703, 0.1299212598425197318, 0.06841997037041518126 ) ) ;
#12834=FACE_OUTER_BOUND ( 'NONE', #23947, .T. ) ;
#12836=CARTESIAN_POINT ( 'NONE',  ( 0.06523048226347956391, -0.1874999998924729294, -0.1574803149606300301 ) ) ;
#12841=CARTESIAN_POINT ( 'NONE',  ( -0.07405724077823318263, -1.071974361930026598, 0.1787899950787401604 ) ) ;
#12843=CARTESIAN_POINT ( 'NONE',  ( 3.284318927891251994E-17, -0.1087598424659214497, 0.1787899950787401882 ) ) ;
#12849=PRODUCT_DEFINITION_SHAPE ( 'NONE', 'NONE',  #16326 ) ;
#12852=CARTESIAN_POINT ( 'NONE',  ( 0.1264236179284866091, -0.5812007873478111097, 0.1264236179284866091 ) ) ;
#12856=CARTESIAN_POINT ( 'NONE',  ( -0.07444174185955065859, -1.228882392260211898, -0.1797182628040039087 ) ) ;
#12866=CARTESIAN_POINT ( 'NONE',  ( 0.1264236179284866091, 0.06348425202226751218, -0.1264236179284866091 ) ) ;
#12873=CARTESIAN_POINT ( 'NONE',  ( 2.892866454678787531E-17, -1.622047243986960430, 0.1574803149606299191 ) ) ;
#12876=CARTESIAN_POINT ( 'NONE',  ( 0.07857503534296064740, -0.08918665060160307911, 0.2400663896719301416 ) ) ;
#12878=CARTESIAN_POINT ( 'NONE',  ( -1.094772975963752103E-17, 0.1077755906049446960, -0.1787899950787401882 ) ) ;
#12885=CARTESIAN_POINT ( 'NONE',  ( 0.07405724077823318263, -1.553149606245448178, -0.1787899950787401604 ) ) ;
#12895=CARTESIAN_POINT ( 'NONE',  ( -0.1459235064575962748, -0.08956109133572084935, -0.09835919643184390382 ) ) ;
#12902=CARTESIAN_POINT ( 'NONE',  ( -0.1787899950787401882, -1.788017669016641831, 0.000000000000000000 ) ) ;
#12907=ADVANCED_FACE ( 'NONE', ( #15069 ), #177, .F. ) ;
#12908=CARTESIAN_POINT ( 'NONE',  ( -0.1787899950787401604, -1.425196850339937482, -0.07405724077823318263 ) ) ;
#12913=CARTESIAN_POINT ( 'NONE',  ( -0.07444174185955065859, -0.7170713686381637864, -0.1797182628040039087 ) ) ;
#12916=CARTESIAN_POINT ( 'NONE',  ( 2.892866454678787531E-17, -0.4507874015748031815, 0.1574803149606299191 ) ) ;
#12929=CARTESIAN_POINT ( 'NONE',  ( -0.1787899950787401882, -0.4729330708123779536, 0.000000000000000000 ) ) ;
#12933=EDGE_LOOP ( 'NONE', ( #6001, #6838, #8112, #29479 ) ) ;
#12936=CARTESIAN_POINT ( 'NONE',  ( -0.07405724077823318263, -1.740157480261197875, -0.1787899950787401604 ) ) ;
#12937=CARTESIAN_POINT ( 'NONE',  ( -0.07405724077823318263, -1.075787401521038689, -0.1787899950787401604 ) ) ;
#12938=CARTESIAN_POINT ( 'NONE',  ( -9.642888182262618425E-18, -1.297244094488189115, -0.1574803149606299191 ) ) ;
#12952=CARTESIAN_POINT ( 'NONE',  ( -0.2082510178749903962, 0.06746187776213008469, 0.1651992896370024499 ) ) ;
#12955=CARTESIAN_POINT ( 'NONE',  ( -0.03350623722892267370, -0.09842519685039370636, 0.2233118325431988072 ) ) ;
#12961=CARTESIAN_POINT ( 'NONE',  ( -0.1787899950787401604, -1.031496062938363822, -0.07405724077823318263 ) ) ;
#12963=CARTESIAN_POINT ( 'NONE',  ( -0.1264236179284866091, -1.176673228292692830, 0.1264236179284866091 ) ) ;
#12965=CARTESIAN_POINT ( 'NONE',  ( -0.07444174185955065859, -0.4414808174570614696, -0.1797182628040039087 ) ) ;
#12969=CARTESIAN_POINT ( 'NONE',  ( 0.1574803149606300301, 0.02903543307086614220, 0.06523048226347956391 ) ) ;
#12970=CARTESIAN_POINT ( 'NONE',  ( -0.1787899950787401604, -0.1653543306548978520, -0.07405724077823318263 ) ) ;
#12978=CARTESIAN_POINT ( 'NONE',  ( 0.1787899950787401604, -0.4999999999462365619, 0.07405724077823318263 ) ) ;
#12980=CARTESIAN_POINT ( 'NONE',  ( 0.1264236179284866091, -1.442421259788756016, 0.1264236179284866091 ) ) ;
#12987=FACE_OUTER_BOUND ( 'NONE', #12933, .T. ) ;
#12988=CARTESIAN_POINT ( 'NONE',  ( 0.06523048226347956391, -1.250492125876724314, -0.1574803149606300301 ) ) ;
#13000=CARTESIAN_POINT ( 'NONE',  ( 0.008047257146029232477, -0.09851385040156239448, 0.2239393559163176950 ) ) ;
#13005=CARTESIAN_POINT ( 'NONE',  ( -0.1787899950787401604, -1.593627905237113174, -0.07405724077823318263 ) ) ;
#13008=CARTESIAN_POINT ( 'NONE',  ( -0.07405724077823318263, -0.5442913385289138706, 0.1787899950787401604 ) ) ;
#13014=CARTESIAN_POINT ( 'NONE',  ( -0.1787899950787401882, -0.3597440944344256208, 0.000000000000000000 ) ) ;
#13015=CARTESIAN_POINT ( 'NONE',  ( 0.1787899950787401604, -0.7263779527021420046, -0.07405724077823318263 ) ) ;
#13020=CARTESIAN_POINT ( 'NONE',  ( 0.1787899950787401882, 0.08206107114083996401, -2.189545951927503898E-17 ) ) ;
#13021=CARTESIAN_POINT ( 'NONE',  ( 3.284318927891251994E-17, -1.801673228292693052, 0.1787899950787401882 ) ) ;
#13028=CARTESIAN_POINT ( 'NONE',  ( -0.1574803149606297803, -0.9699803149606308628, 0.06523048226347956391 ) ) ;
#13031=CARTESIAN_POINT ( 'NONE',  ( -0.1270800023317771588, -1.502012313520053155, -0.1270800023317771588 ) ) ;
#13033=CARTESIAN_POINT ( 'NONE',  ( -1.094772975963752103E-17, -0.3646653542769452971, -0.1787899950787401882 ) ) ;
#13036=CARTESIAN_POINT ( 'NONE',  ( 0.1888124183976733761, 0.07899857248962396938, -0.1764221702779007750 ) ) ;
#13041=CARTESIAN_POINT ( 'NONE',  ( 0.1787899950787401882, 0.01427165359707061217, -2.189545951927503898E-17 ) ) ;
#13053=CARTESIAN_POINT ( 'NONE',  ( 3.284318927891251994E-17, -1.294783464513165283, 0.1787899950787401882 ) ) ;
#13068=CARTESIAN_POINT ( 'NONE',  ( -0.03026318032628478802, -0.09782597982458868247, 0.1548971533202315731 ) ) ;
#13072=CARTESIAN_POINT ( 'NONE',  ( -0.1574803149606297803, -0.2514763778452289711, 0.06523048226347956391 ) ) ;
#13074=VECTOR ( 'NONE', #6883, 39.37007874015748143 ) ;
#13078=DIRECTION ( 'NONE',  ( 0.000000000000000000, 0.8660254037844383745, 0.5000000000000003331 ) ) ;
#13080=CARTESIAN_POINT ( 'NONE',  ( 0.07405724077823318263, -1.131029480040261603, -0.1787899950787401604 ) ) ;
#13082=CARTESIAN_POINT ( 'NONE',  ( -0.1787899950787401882, -0.1579724408911182820, 0.000000000000000000 ) ) ;
#13089=CARTESIAN_POINT ( 'NONE',  ( 3.284318927891251994E-17, -0.5861220471903307860, 0.1787899950787401882 ) ) ;
#13093=CARTESIAN_POINT ( 'NONE',  ( -1.100456976456230270E-17, -1.113232785960998061, -0.1797182628040039365 ) ) ;
#13104=CARTESIAN_POINT ( 'NONE',  ( 0.03556354040786432330, 0.1286422661082892160, 0.1787899950787401604 ) ) ;
#13113=CARTESIAN_POINT ( 'NONE',  ( 0.1574803149606299191, -1.612204724301921077, -1.928577636452523993E-17 ) ) ;
#13118=CARTESIAN_POINT ( 'NONE',  ( 0.05938635157346154603, -0.07958416565547918320, 0.2511462791696609798 ) ) ;
#13119=CARTESIAN_POINT ( 'NONE',  ( 0.1787899950787401882, 0.05856299217974772486, -2.189545951927503898E-17 ) ) ;
#13123=PLANE ( 'NONE',  #25236 ) ;
#13124=CARTESIAN_POINT ( 'NONE',  ( -0.08443540605192620396, 0.09133345722616742490, 0.2366842664529267282 ) ) ;
#13127=CARTESIAN_POINT ( 'NONE',  ( 0.1113553986120547346, -0.3966535431995590888, 0.1113553986120547346 ) ) ;
#13128=CARTESIAN_POINT ( 'NONE',  ( 0.1264236179284866091, -1.634350393647023614, -0.1264236179284866091 ) ) ;
#13136=CARTESIAN_POINT ( 'NONE',  ( -0.1264236179284866091, -0.6512066453945926092, -0.1264236179284866091 ) ) ;
#13138=CARTESIAN_POINT ( 'NONE',  ( 0.2030945033354783491, -0.08956025807989388687, 0.03023235614309822961 ) ) ;
#13151=CARTESIAN_POINT ( 'NONE',  ( -0.07444174185955065859, -0.7564414473783218629, -0.1797182628040039087 ) ) ;
#13152=CARTESIAN_POINT ( 'NONE',  ( 0.2471922904502826812, 0.09572725253288333347, 0.02812286105088213084 ) ) ;
#13155=CARTESIAN_POINT ( 'NONE',  ( -0.1574803149606300301, -0.4630905511811017616, -0.06523048226347956391 ) ) ;
#13159=CARTESIAN_POINT ( 'NONE',  ( 0.1574803149606300301, 0.03395669291338582890, -0.06523048226347956391 ) ) ;
#13164=CIRCLE ( 'NONE', #34590, 0.2471922904502826812 ) ;
#13167=CARTESIAN_POINT ( 'NONE',  ( 0.1264236179284866091, -0.5270669290800944484, -0.1264236179284866091 ) ) ;
#13174=CARTESIAN_POINT ( 'NONE',  ( 0.07405724077823318263, -1.641732283410802573, 0.1787899950787401604 ) ) ;
#13175=CARTESIAN_POINT ( 'NONE',  ( 0.1264236179284866091, -1.122539370024976391, -0.1264236179284866091 ) ) ;
#13176=CARTESIAN_POINT ( 'NONE',  ( -0.1574803149606299191, -1.444881889763779625, 0.000000000000000000 ) ) ;
#13190=CARTESIAN_POINT ( 'NONE',  ( 0.05264611394417172130, -0.07553294269950974749, -0.2550375247538704815 ) ) ;
#13193=CARTESIAN_POINT ( 'NONE',  ( -0.1264236179284866091, -0.2082932595678216314, 0.1264236179284866091 ) ) ;
#13195=CARTESIAN_POINT ( 'NONE',  ( -0.04516133130590834627, -0.09842519685039370636, -0.1820366505350590747 ) ) ;
#13204=CARTESIAN_POINT ( 'NONE',  ( -0.07405724077823318263, -1.021653543253323138, 0.1787899950787401604 ) ) ;
#13205=CARTESIAN_POINT ( 'NONE',  ( -0.1787899950787401882, -1.260334645615527549, 0.000000000000000000 ) ) ;
#13207=CARTESIAN_POINT ( 'NONE',  ( -0.1270800023317771588, -0.5079178253310770996, 0.1270800023317771588 ) ) ;
#13210=CARTESIAN_POINT ( 'NONE',  ( -0.1113553986120547346, -0.02263779527559055260, 0.1113553986120547346 ) ) ;
#13217=CARTESIAN_POINT ( 'NONE',  ( 0.1574803149606299191, -0.9822834644594016229, -1.928577636452523993E-17 ) ) ;
#13218=CARTESIAN_POINT ( 'NONE',  ( 0.07405724077823318263, -0.6476377952218281830, -0.1787899950787401604 ) ) ;
#13219=CARTESIAN_POINT ( 'NONE',  ( -0.07405724077823318263, -1.385826771599779184, -0.1787899950787401604 ) ) ;
#13234=CARTESIAN_POINT ( 'NONE',  ( 0.1545837415703855688, -0.09842296937465562501, -0.08999940835115426141 ) ) ;
#13238=CARTESIAN_POINT ( 'NONE',  ( 0.1850388559544986211, -0.08126078924503041256, 0.1786007880588302565 ) ) ;
#13239=CARTESIAN_POINT ( 'NONE',  ( 0.1113553986120547346, -0.08169291338582677919, -0.1113553986120547346 ) ) ;
#13241=CARTESIAN_POINT ( 'NONE',  ( -0.2471922904502826812, 0.09842519685039370636, 5.914624404477007554E-17 ) ) ;
#13243=CARTESIAN_POINT ( 'NONE',  ( -0.08394057657693032581, -0.09851384873590177116, 0.2125522580681921125 ) ) ;
#13247=CARTESIAN_POINT ( 'NONE',  ( 0.07405724077823318263, -1.578864125709555477, 0.1787899950787401604 ) ) ;
#13250=CARTESIAN_POINT ( 'NONE',  ( -0.1787899950787401604, -0.5492125983714331028, 0.07405724077823318263 ) ) ;
#13255=CARTESIAN_POINT ( 'NONE',  ( -0.1787899950787401604, -0.7066929133320629663, 0.07405724077823318263 ) ) ;
#13262=CARTESIAN_POINT ( 'NONE',  ( 0.1264236179284866091, 0.07713981129832027384, 0.1264236179284866091 ) ) ;
#13267=CARTESIAN_POINT ( 'NONE',  ( -0.1113553986120547346, -0.9773622047244094890, -0.1113553986120547346 ) ) ;
#13269=CARTESIAN_POINT ( 'NONE',  ( -0.1797182628040039087, -1.617661919819267213, -0.07444174185955065859 ) ) ;
#13275=CARTESIAN_POINT ( 'NONE',  ( 0.1264236179284866091, -0.09891732278088229136, -0.1264236179284866091 ) ) ;
#13276=CARTESIAN_POINT ( 'NONE',  ( 0.1787899950787401604, -0.06200787396198446239, 0.07405724077823318263 ) ) ;
#13278=CARTESIAN_POINT ( 'NONE',  ( -0.1264236179284866091, -0.9109251967966299768, -0.1264236179284866091 ) ) ;
#13299=CARTESIAN_POINT ( 'NONE',  ( 3.284318927891251994E-17, 0.08316929139234625901, 0.1787899950787401882 ) ) ;
#13304=CARTESIAN_POINT ( 'NONE',  ( 3.284318927891251994E-17, -1.187623968229238214, 0.1787899950787401882 ) ) ;
#13307=CARTESIAN_POINT ( 'NONE',  ( 3.284318927891251994E-17, -0.06938976372576398377, 0.1787899950787401882 ) ) ;
#13314=CARTESIAN_POINT ( 'NONE',  ( -0.07405724077823318263, -0.7608267715997808489, -0.1787899950787401604 ) ) ;
#13318=CARTESIAN_POINT ( 'NONE',  ( 0.1270800023317771588, -1.167366644228714501, 0.1270800023317771588 ) ) ;
#13323=EDGE_CURVE ( 'NONE', #2820, #4638, #2194, .T. ) ;
#13328=CARTESIAN_POINT ( 'NONE',  ( -1.094772975963752103E-17, 0.02903543312462964626, -0.1787899950787401882 ) ) ;
#13341=CARTESIAN_POINT ( 'NONE',  ( 0.1036066153429698738, -0.09660391682274865888, 0.2256134787373819950 ) ) ;
#13343=CARTESIAN_POINT ( 'NONE',  ( 3.284318927891251994E-17, 0.08809055123486594918, 0.1787899950787401882 ) ) ;
#13350=CARTESIAN_POINT ( 'NONE',  ( -0.1264236179284866091, -1.614665354276944909, 0.1264236179284866091 ) ) ;
#13357=CARTESIAN_POINT ( 'NONE',  ( 0.1529906210716822090, 0.1251777869743438687, -0.05500979718732867257 ) ) ;
#13358=DIRECTION ( 'NONE',  ( 0.000000000000000000, 0.000000000000000000, 1.000000000000000000 ) ) ;
#13359=CARTESIAN_POINT ( 'NONE',  ( -0.1787899950787401882, -0.6856554642922303433, 0.000000000000000000 ) ) ;
#13361=CARTESIAN_POINT ( 'NONE',  ( 0.1078383211903921335, -0.08956014831809350207, 0.1858721435341346429 ) ) ;
#13362=CARTESIAN_POINT ( 'NONE',  ( -0.04828142644392272725, -0.08854577535781626985, 0.1504058830162713911 ) ) ;
#13368=ORIENTED_EDGE ( 'NONE', *, *, #45103, .T. ) ;
#13378=CARTESIAN_POINT ( 'NONE',  ( -0.06523048226347956391, -0.5073818897637790704, -0.1574803149606300301 ) ) ;
#13387=CARTESIAN_POINT ( 'NONE',  ( 0.06523048226347956391, -0.5812007872940475606, -0.1574803149606300301 ) ) ;
#13392=CARTESIAN_POINT ( 'NONE',  ( -0.1787899950787401604, -0.5935039369541101895, -0.07405724077823318263 ) ) ;
#13394=ORIENTED_EDGE ( 'NONE', *, *, #16001, .F. ) ;
#13398=CARTESIAN_POINT ( 'NONE',  ( -0.05769625742918065708, 0.07859832706092176324, -0.2521221211081704494 ) ) ;
#13399=FACE_OUTER_BOUND ( 'NONE', #45385, .T. ) ;
#13400=CARTESIAN_POINT ( 'NONE',  ( 0.1270800023317771588, 0.05310579671616700442, 0.1270800023317771588 ) ) ;
#13401=CARTESIAN_POINT ( 'NONE',  ( -0.07405724077823318263, -1.021653543253323138, 0.1787899950787401604 ) ) ;
#13402=CARTESIAN_POINT ( 'NONE',  ( 0.1574803149606300301, -1.304625984251967630, -0.06523048226347956391 ) ) ;
#13410=CARTESIAN_POINT ( 'NONE',  ( 0.1574803149606299191, 0.001968504044534917247, -1.928577636452523993E-17 ) ) ;
#13419=CARTESIAN_POINT ( 'NONE',  ( 0.07405724077823318263, -0.2796515272843568267, 0.1787899950787401604 ) ) ;
#13420=CARTESIAN_POINT ( 'NONE',  ( 0.05362475593144094138, -0.09842519685039370636, 0.2150385860745854250 ) ) ;
#13430=CARTESIAN_POINT ( 'NONE',  ( -0.1787899950787401882, -1.068405511757259951, 0.000000000000000000 ) ) ;
#13431=CARTESIAN_POINT ( 'NONE',  ( -0.07405724077823318263, -1.149606299158835387, -0.1787899950787401604 ) ) ;
#13432=CARTESIAN_POINT ( 'NONE',  ( 3.301370929368692659E-17, -0.5423666442287149447, 0.1797182628040039365 ) ) ;
#13437=CARTESIAN_POINT ( 'NONE',  ( -0.1113553986120547346, 0.01673228346456692717, 0.1113553986120547346 ) ) ;
#13445=CARTESIAN_POINT ( 'NONE',  ( -0.1574803149606300301, -1.004429133750739833, -0.06523048226347956391 ) ) ;
#13446=CARTESIAN_POINT ( 'NONE',  ( -0.1787899950787401882, -0.5959645668753701386, 0.000000000000000000 ) ) ;
#13447=CARTESIAN_POINT ( 'NONE',  ( 0.1787899950787401882, -1.319389763725763665, -2.189545951927503898E-17 ) ) ;
#13457=CARTESIAN_POINT ( 'NONE',  ( 0.1287673665127798128, -0.09842951992213312684, -0.1240475571185562509 ) ) ;
#13460=CARTESIAN_POINT ( 'NONE',  ( 0.2278981769376444422, -0.05062618494133044184, 0.1538518510339534628 ) ) ;
#13467=CARTESIAN_POINT ( 'NONE',  ( -0.03865401764462641360, -0.09851384930164665266, 0.2227661591646389883 ) ) ;
#13470=CARTESIAN_POINT ( 'NONE',  ( 0.1787899950787401604, -1.573942865867034246, 0.07405724077823318263 ) ) ;
#13472=CARTESIAN_POINT ( 'NONE',  ( -1.094772975963752103E-17, -0.5615157479777322935, -0.1787899950787401882 ) ) ;
#13478=CARTESIAN_POINT ( 'NONE',  ( 0.1787899950787401882, -0.2613188975840319284, -2.189545951927503898E-17 ) ) ;
#13479=ADVANCED_FACE ( 'NONE', ( #29674 ), #43986, .T. ) ;
#13483=CARTESIAN_POINT ( 'NONE',  ( -0.1264236179284866091, -0.02128538555207338742, -0.1264236179284866091 ) ) ;
#13484=CARTESIAN_POINT ( 'NONE',  ( 0.07405724077823318263, 0.08562992131360593062, 0.1787899950787401604 ) ) ;
#13489=CARTESIAN_POINT ( 'NONE',  ( -0.1574803149606299191, -0.8543307086614173596, 0.000000000000000000 ) ) ;
#13491=CARTESIAN_POINT ( 'NONE',  ( -0.1797182628040039087, -1.735772156039738778, -0.07444174185955065859 ) ) ;
#13501=CARTESIAN_POINT ( 'NONE',  ( -1.094772975963752103E-17, -0.1333661416785198728, -0.1787899950787401882 ) ) ;
#13503=CARTESIAN_POINT ( 'NONE',  ( -1.094772975963752103E-17, -0.8764763778989921317, -0.1787899950787401882 ) ) ;
#13521=( BOUNDED_CURVE ( )  B_SPLINE_CURVE ( 2, ( #36793, #33459, #30120, #44655, #26499, #41059, #8257, #22882, #12596 ),
 .UNSPECIFIED., .F., .T. ) 
 B_SPLINE_CURVE_WITH_KNOTS ( ( 3, 2, 2, 2, 3 ),
 ( 0.05500000000000000028, 0.05750000000000000250, 0.05999999999999999778, 0.06250000000000000000, 0.06500000000000000222 ),
 .UNSPECIFIED. ) 
 CURVE ( )  GEOMETRIC_REPRESENTATION_ITEM ( )  RATIONAL_B_SPLINE_CURVE ( ( 1.000000000000000000, 0.9238795325112869605, 1.000000000000000000, 0.9238795325112869605, 1.000000000000000000, 0.9238795325112869605, 1.000000000000000000, 0.9238795325112869605, 1.000000000000000000 ) ) 
 REPRESENTATION_ITEM ( '' )  ) ;
#13524=CARTESIAN_POINT ( 'NONE',  ( 0.1787899950787401604, -1.175320818622938912, -0.07405724077823318263 ) ) ;
#13526=CARTESIAN_POINT ( 'NONE',  ( -0.1264236179284866091, -0.1924212597887563214, 0.1264236179284866091 ) ) ;
#13534=CARTESIAN_POINT ( 'NONE',  ( 0.1797182628040039087, -0.2200241245436755921, 0.07444174185955046430 ) ) ;
#13538=CARTESIAN_POINT ( 'NONE',  ( 3.301370929368692659E-17, -1.329768219031864041, 0.1797182628040039365 ) ) ;
#13547=CARTESIAN_POINT ( 'NONE',  ( 0.1787899950787401882, 0.01919291343959027632, -2.189545951927503898E-17 ) ) ;
#13561=CARTESIAN_POINT ( 'NONE',  ( -0.07405724077823318263, -0.03248031490686641154, 0.1787899950787401604 ) ) ;
#13568=CARTESIAN_POINT ( 'NONE',  ( 0.07405724077823318263, -1.671259842465922407, -0.1787899950787401604 ) ) ;
#13575=ORIENTED_EDGE ( 'NONE', *, *, #45043, .F. ) ;
#13576=CARTESIAN_POINT ( 'NONE',  ( -0.1165037417137196885, -0.08956132732375866878, 0.1114237959394338701 ) ) ;
#13581=CARTESIAN_POINT ( 'NONE',  ( 2.892866454678787531E-17, 0.06102362204724409711, 0.1574803149606299191 ) ) ;
#13590=CARTESIAN_POINT ( 'NONE',  ( 0.07444174185955046430, -0.7219926284806829075, -0.1797182628040039087 ) ) ;
#13593=CARTESIAN_POINT ( 'NONE',  ( 0.06523048226347956391, -0.5910433070866143446, -0.1574803149606300301 ) ) ;
#13594=CARTESIAN_POINT ( 'NONE',  ( 0.2471922904502826812, 0.03219022224904102836, -0.1427165354330708902 ) ) ;
#13612=CARTESIAN_POINT ( 'NONE',  ( -1.100456976456230270E-17, 0.06786957624372617903, -0.1797182628040039365 ) ) ;
#13613=CARTESIAN_POINT ( 'NONE',  ( -0.07405724077823318263, -0.9822834645131651721, 0.1787899950787401604 ) ) ;
#13614=CARTESIAN_POINT ( 'NONE',  ( 0.06523048226347956391, -1.457185039370078483, -0.1574803149606300301 ) ) ;
#13630=CARTESIAN_POINT ( 'NONE',  ( -0.2471922904502826812, 0.09210780053718727045, 0.04262551151394271265 ) ) ;
#13632=CARTESIAN_POINT ( 'NONE',  ( -0.1478471407235199264, 0.09575019180979009448, 0.2000734843705010146 ) ) ;
#13635=CARTESIAN_POINT ( 'NONE',  ( 0.1264236179284866091, -0.3067184564182153794, -0.1264236179284866091 ) ) ;
#13646=CARTESIAN_POINT ( 'NONE',  ( 0.1264236179284866091, -1.201279527505291433, -0.1264236179284866091 ) ) ;
#13647=CARTESIAN_POINT ( 'NONE',  ( 0.07405724077823318263, -1.233267716481668774, -0.1787899950787401604 ) ) ;
#13650=CARTESIAN_POINT ( 'NONE',  ( 0.1270800023317771588, -0.5669729434413133262, -0.1270800023317771588 ) ) ;
#13654=CARTESIAN_POINT ( 'NONE',  ( -0.1574803149606299191, -0.1456692913385826960, 0.000000000000000000 ) ) ;
#13665=CARTESIAN_POINT ( 'NONE',  ( -1.094772975963752103E-17, -0.5270669290800944484, -0.1787899950787401882 ) ) ;
#13666=CARTESIAN_POINT ( 'NONE',  ( -0.1264236179284866091, -1.422736220418677311, -0.1264236179284866091 ) ) ;
#13671=VERTEX_POINT ( 'NONE', #4666 ) ;
#13672=CARTESIAN_POINT ( 'NONE',  ( 0.000000000000000000, -0.09842519685039370636, 0.000000000000000000 ) ) ;
#13677=CARTESIAN_POINT ( 'NONE',  ( 0.2020936974007922493, -0.07057211410380534455, 0.1687521643630704726 ) ) ;
#13688=CARTESIAN_POINT ( 'NONE',  ( 0.2037444935048909334, -0.09851384560802105284, 0.05109213554274055769 ) ) ;
#13692=CARTESIAN_POINT ( 'NONE',  ( 0.1787899950787401604, -1.687131842244987023, -0.07405724077823318263 ) ) ;
#13694=CARTESIAN_POINT ( 'NONE',  ( 0.1264236179284866091, -0.5369094487651339120, 0.1264236179284866091 ) ) ;
#13701=CARTESIAN_POINT ( 'NONE',  ( 0.1787899950787401604, -0.2588582676627719792, -0.07405724077823318263 ) ) ;
#13706=CARTESIAN_POINT ( 'NONE',  ( 3.284318927891251994E-17, 0.07221855145580058366, 0.1787899950787401882 ) ) ;
#13707=CARTESIAN_POINT ( 'NONE',  ( -0.07405724077823318263, 0.08070866147108628208, 0.1787899950787401604 ) ) ;
#13714=CARTESIAN_POINT ( 'NONE',  ( 0.06523048226347956391, -0.8666338582677162172, -0.1574803149606300301 ) ) ;
#13716=CARTESIAN_POINT ( 'NONE',  ( 0.07444174185955065859, -1.721008376512180860, 0.1797182628040039087 ) ) ;
#13717=CARTESIAN_POINT ( 'NONE',  ( -1.094772975963752103E-17, -0.3252952755367877757, -0.1787899950787401882 ) ) ;
#13720=CARTESIAN_POINT ( 'NONE',  ( 0.2082510178750321406, 0.06746187776208821540, -0.1651992896369783026 ) ) ;
#13725=CARTESIAN_POINT ( 'NONE',  ( 0.1264236179284866091, -0.05954724404072461036, -0.1264236179284866091 ) ) ;
#13728=CARTESIAN_POINT ( 'NONE',  ( 0.07405724077823318263, -0.8543307086076546986, 0.1787899950787401604 ) ) ;
#13736=CARTESIAN_POINT ( 'NONE',  ( -0.06523048226347956391, -1.152066929026331676, 0.1574803149606297803 ) ) ;
#13757=CARTESIAN_POINT ( 'NONE',  ( -1.094772975963752103E-17, -1.207309007599316919, -0.1787899950787401882 ) ) ;
#13759=CARTESIAN_POINT ( 'NONE',  ( 0.1264236179284866091, -0.09399606293836260118, -0.1264236179284866091 ) ) ;
#13766=CARTESIAN_POINT ( 'NONE',  ( 0.1787899950787401604, -1.444881889710016631, 0.07405724077823318263 ) ) ;
#13800=CARTESIAN_POINT ( 'NONE',  ( 0.1607584476970183585, 0.09202339627321219628, 0.1926191378137618593 ) ) ;
#13802=ORIENTED_EDGE ( 'NONE', *, *, #1297, .F. ) ;
#13805=ORIENTED_EDGE ( 'NONE', *, *, #27645, .T. ) ;
#13807=CARTESIAN_POINT ( 'NONE',  ( 0.07405724077823318263, -1.749999999946236340, -0.1787899950787401604 ) ) ;
#13812=EDGE_CURVE ( 'NONE', #3096, #5551, #21348, .T. ) ;
#13815=CARTESIAN_POINT ( 'NONE',  ( -0.1787899950787401604, -0.7274861729536492572, -0.07405724077823318263 ) ) ;
#13817=CARTESIAN_POINT ( 'NONE',  ( 0.08374778445418129547, -0.08956243157244035691, 0.1193195044654234288 ) ) ;
#13832=CARTESIAN_POINT ( 'NONE',  ( 0.1797182628040039087, -0.8893154631263514576, 0.07444174185955046430 ) ) ;
#13834=CARTESIAN_POINT ( 'NONE',  ( 0.1113553986120547346, -0.5541338582677165503, -0.1113553986120547346 ) ) ;
#13841=CARTESIAN_POINT ( 'NONE',  ( 0.06523048226347956391, -0.6599409447743623813, -0.1574803149606300301 ) ) ;
#13845=CARTESIAN_POINT ( 'NONE',  ( -0.07405724077823318263, -0.6230314960092281362, 0.1787899950787401604 ) ) ;
#13854=CARTESIAN_POINT ( 'NONE',  ( -0.1797182628040039087, 0.03588138726734815126, -0.07444174185955065859 ) ) ;
#13855=CARTESIAN_POINT ( 'NONE',  ( -0.07405724077823318263, -1.036417322780882833, -0.1787899950787401604 ) ) ;
#13856=CARTESIAN_POINT ( 'NONE',  ( 0.1574803149606300301, -1.585137795275590955, 0.06523048226347956391 ) ) ;
#13857=CARTESIAN_POINT ( 'NONE',  ( 2.700008691033534577E-17, 0.0004086818895575684884, 0.2204724409448818867 ) ) ;
#13874=CARTESIAN_POINT ( 'NONE',  ( 3.284318927891251994E-17, -0.2033719997253019829, 0.1787899950787401882 ) ) ;
#13876=CARTESIAN_POINT ( 'NONE',  ( -0.1717103871139409321, -0.09842519685039370636, -0.03673106526238755637 ) ) ;
#13884=CARTESIAN_POINT ( 'NONE',  ( -1.094772975963752103E-17, -1.117618110182456714, -0.1787899950787401882 ) ) ;
#13886=CARTESIAN_POINT ( 'NONE',  ( -0.1787899950787401604, -1.454724409395055096, 0.07405724077823318263 ) ) ;
#13904=CARTESIAN_POINT ( 'NONE',  ( -0.06523048226347956391, -1.481791338475149322, -0.1574803149606300301 ) ) ;
#13905=CARTESIAN_POINT ( 'NONE',  ( 0.1787899950787401604, -0.5393700786863945273, 0.07405724077823318263 ) ) ;
#13906=CARTESIAN_POINT ( 'NONE',  ( 0.1574803149606299191, -0.9921259842519685179, -1.928577636452523993E-17 ) ) ;
#13923=CARTESIAN_POINT ( 'NONE',  ( 0.1986060025684610320, -0.07294156354275010967, 0.1707667409196649000 ) ) ;
#13926=CARTESIAN_POINT ( 'NONE',  ( -0.06523048226347956391, -0.1432086613097958705, -0.1574803149606300301 ) ) ;
#13928=CARTESIAN_POINT ( 'NONE',  ( 0.1235961452251413406, -0.09842519685039370636, -0.2140748031496062798 ) ) ;
#13936=( BOUNDED_CURVE ( )  B_SPLINE_CURVE ( 2, ( #30076, #7978, #14957, #21902, #29136, #7505, #47302, #44613, #22125 ),
 .UNSPECIFIED., .F., .T. ) 
 B_SPLINE_CURVE_WITH_KNOTS ( ( 3, 2, 2, 2, 3 ),
 ( 0.05500000000000000028, 0.05750000000000000250, 0.05999999999999999778, 0.06250000000000000000, 0.06500000000000000222 ),
 .UNSPECIFIED. ) 
 CURVE ( )  GEOMETRIC_REPRESENTATION_ITEM ( )  RATIONAL_B_SPLINE_CURVE ( ( 1.000000000000000000, 0.9238795325112869605, 1.000000000000000000, 0.9238795325112869605, 1.000000000000000000, 0.9238795325112869605, 1.000000000000000000, 0.9238795325112869605, 1.000000000000000000 ) ) 
 REPRESENTATION_ITEM ( '' )  ) ;
#13937=ORIENTED_EDGE ( 'NONE', *, *, #19047, .F. ) ;
#13938=CARTESIAN_POINT ( 'NONE',  ( 0.07405724077823318263, -0.6820866141194646959, -0.1787899950787401604 ) ) ;
#13943=CARTESIAN_POINT ( 'NONE',  ( -1.094772975963752103E-17, -0.7977362204186770889, -0.1787899950787401882 ) ) ;
#13947=CARTESIAN_POINT ( 'NONE',  ( -0.07405724077823318263, -0.1418562516938056128, -0.1787899950787401604 ) ) ;
#13955=CARTESIAN_POINT ( 'NONE',  ( -0.07444174185955065859, -1.765299715094856614, 0.1797182628040039087 ) ) ;
#13956=CARTESIAN_POINT ( 'NONE',  ( -0.07405724077823318263, -0.4409448818359998357, -0.1787899950787401604 ) ) ;
#13962=ORIENTED_EDGE ( 'NONE', *, *, #36802, .F. ) ;
#13964=CARTESIAN_POINT ( 'NONE',  ( -0.2374471364664500761, -0.04193537623287351551, -0.1483429027089311902 ) ) ;
#13967=CARTESIAN_POINT ( 'NONE',  ( 0.1787899950787401604, -0.1850393700249766959, 0.07405724077823318263 ) ) ;
#13969=CARTESIAN_POINT ( 'NONE',  ( 0.07405724077823318263, -1.115157480261196987, -0.1787899950787401604 ) ) ;
#13979=CARTESIAN_POINT ( 'NONE',  ( 0.2471922904502826812, -0.09842519685039370636, 0.1427165354330708902 ) ) ;
#13983=DIRECTION ( 'NONE',  ( 0.000000000000000000, 0.000000000000000000, 1.000000000000000000 ) ) ;
#13986=PRODUCT_DEFINITION_CONTEXT ( 'detailed design', #12252, 'design' ) ;
#13990=CARTESIAN_POINT ( 'NONE',  ( -1.094772975963752103E-17, 0.02411417328210995956, -0.1787899950787401882 ) ) ;
#13998=CARTESIAN_POINT ( 'NONE',  ( -0.1787899950787401604, -1.239297196575694926, -0.07405724077823318263 ) ) ;
#14000=CARTESIAN_POINT ( 'NONE',  ( -0.07405724077823318263, -0.2440944881352131168, -0.1787899950787401604 ) ) ;
#14007=AXIS2_PLACEMENT_3D ( 'NONE', #20725, #5890, #2511 ) ;
#14008=CARTESIAN_POINT ( 'NONE',  ( -0.07405724077823318263, -1.533464566875370805, 0.1787899950787401604 ) ) ;
#14009=CARTESIAN_POINT ( 'NONE',  ( 0.07405724077823318263, -0.7805118109698575557, 0.1787899950787401604 ) ) ;
#14012=CARTESIAN_POINT ( 'NONE',  ( 0.1797182628040039087, -1.243646171787769816, 0.07444174185955046430 ) ) ;
#14019=FACE_OUTER_BOUND ( 'NONE', #28002, .T. ) ;
#14021=CARTESIAN_POINT ( 'NONE',  ( -0.06523048226347956391, -0.7583661416247552411, 0.1574803149606297803 ) ) ;
#14023=CARTESIAN_POINT ( 'NONE',  ( 3.284318927891251994E-17, 0.04872047249470835839, 0.1787899950787401882 ) ) ;
#14039=CARTESIAN_POINT ( 'NONE',  ( 0.07405724077823318263, -0.02755905506434671789, 0.1787899950787401604 ) ) ;
#14047=CARTESIAN_POINT ( 'NONE',  ( 0.1787899950787401604, -1.720472440891118726, 0.07405724077823318263 ) ) ;
#14055=CARTESIAN_POINT ( 'NONE',  ( 0.07405724077823318263, -0.7520924721662473056, 0.1787899950787401604 ) ) ;
#14057=CARTESIAN_POINT ( 'NONE',  ( 2.892866454678787531E-17, -0.007874015640504449659, 0.1574803149606299191 ) ) ;
#14064=CARTESIAN_POINT ( 'NONE',  ( 0.1574803149606300301, -0.01033464566929132716, 0.06523048226347956391 ) ) ;
#14074=CARTESIAN_POINT ( 'NONE',  ( 0.07444174185955065859, -0.8548666442287150558, 0.1797182628040039087 ) ) ;
#14075=CARTESIAN_POINT ( 'NONE',  ( 0.2471922904502827090, 0.06732389326662464868, 0.09794877975417727589 ) ) ;
#14077=AXIS2_PLACEMENT_3D ( 'NONE', #39092, #9885, #24498 ) ;
#14080=CARTESIAN_POINT ( 'NONE',  ( 0.06523048226347956391, -0.6451771653543302287, 0.1574803149606297803 ) ) ;
#14091=CARTESIAN_POINT ( 'NONE',  ( 3.284318927891251994E-17, -0.6599409448281259305, 0.1787899950787401882 ) ) ;
#14100=CARTESIAN_POINT ( 'NONE',  ( 0.1787899950787401604, -1.794291338528913426, 0.07405724077823318263 ) ) ;
#14101=CARTESIAN_POINT ( 'NONE',  ( -0.07405724077823318263, -1.193897637741512696, -0.1787899950787401604 ) ) ;
#14102=CARTESIAN_POINT ( 'NONE',  ( 0.06523048226347956391, -1.496555118110236782, -0.1574803149606300301 ) ) ;
#14105=VERTEX_POINT ( 'NONE', #31984 ) ;
#14106=CARTESIAN_POINT ( 'NONE',  ( -0.06523048226347956391, 0.06840551191855072377, 0.1574803149606297803 ) ) ;
#14115=CARTESIAN_POINT ( 'NONE',  ( -0.2471922904502825702, 0.05534442469272835008, 0.1143959998688603985 ) ) ;
#14117=CARTESIAN_POINT ( 'NONE',  ( 0.07564704710180411573, -0.08785038237306361242, -0.2417569064345358731 ) ) ;
#14120=CARTESIAN_POINT ( 'NONE',  ( 0.1264236179284866091, -0.4641987713788449099, -0.1264236179284866091 ) ) ;
#14121=CARTESIAN_POINT ( 'NONE',  ( -0.1490350107398933088, -0.09842519685039370636, -0.1001871157495389797 ) ) ;
#14129=CARTESIAN_POINT ( 'NONE',  ( 0.1787899950787401604, -1.164370078686393306, -0.07405724077823318263 ) ) ;
#14130=CARTESIAN_POINT ( 'NONE',  ( -0.07405724077823318263, -1.371062992072219489, 0.1787899950787401604 ) ) ;
#14139=CARTESIAN_POINT ( 'NONE',  ( 0.1574803149606299191, -0.08661417322834646937, -1.928577636452523993E-17 ) ) ;
#14149=CARTESIAN_POINT ( 'NONE',  ( -0.07405724077823318263, -0.03248031490686641154, 0.1787899950787401604 ) ) ;
#14150=CARTESIAN_POINT ( 'NONE',  ( -9.642888182262618425E-18, 0.09055118120988918384, -0.1574803149606299191 ) ) ;
#14152=CARTESIAN_POINT ( 'NONE',  ( 0.1113553986120547346, -1.499015747923968522, 0.1113553986120547346 ) ) ;
#14153=CARTESIAN_POINT ( 'NONE',  ( -0.1787899950787401882, -0.6353346456155275490, 0.000000000000000000 ) ) ;
#14154=CARTESIAN_POINT ( 'NONE',  ( 2.892866454678787531E-17, -1.120078740157480324, 0.1574803149606299191 ) ) ;
#14172=CARTESIAN_POINT ( 'NONE',  ( 0.1574803149606300301, -0.2760826770578272416, 0.06523048226347956391 ) ) ;
#14179=CARTESIAN_POINT ( 'NONE',  ( -0.1564116827871401549, -0.09851383672212755960, -0.08632843964392854230 ) ) ;
#14183=CARTESIAN_POINT ( 'NONE',  ( -0.1787899950787401882, -1.748647590276482422, 0.000000000000000000 ) ) ;
#14188=CARTESIAN_POINT ( 'NONE',  ( -0.1264236179284866091, -0.9404527558517480346, 0.1264236179284866091 ) ) ;
#14190=CARTESIAN_POINT ( 'NONE',  ( -0.2471922436403682644, -0.09120620265207400601, -0.04599440333008567028 ) ) ;
#14193=CARTESIAN_POINT ( 'NONE',  ( -0.1787899950787401604, -0.09264365326860893313, 0.07405724077823318263 ) ) ;
#14194=CARTESIAN_POINT ( 'NONE',  ( -0.07405724077823318263, -0.2440944881352131168, -0.1787899950787401604 ) ) ;
#14195=CARTESIAN_POINT ( 'NONE',  ( 0.1787899950787401882, 0.09301181107738563936, -2.189545951927503898E-17 ) ) ;
#14200=CARTESIAN_POINT ( 'NONE',  ( 2.458936486476969154E-17, 0.1299212598425196763, -0.2007874015748031815 ) ) ;
#14202=CARTESIAN_POINT ( 'NONE',  ( 0.1797182628040039365, -1.792366644228716721, -2.200913952912460540E-17 ) ) ;
#14205=CARTESIAN_POINT ( 'NONE',  ( 0.07405724077823318263, -0.4606299212060784853, 0.1787899950787401604 ) ) ;
#14216=CARTESIAN_POINT ( 'NONE',  ( -0.1787899950787401604, -0.08661417317458304510, -0.07405724077823318263 ) ) ;
#14218=CARTESIAN_POINT ( 'NONE',  ( 3.284318927891251994E-17, -1.014271653489543290, 0.1787899950787401882 ) ) ;
#14224=CARTESIAN_POINT ( 'NONE',  ( -0.1574803149606299191, -1.159448818790110192, 0.000000000000000000 ) ) ;
#14238=CARTESIAN_POINT ( 'NONE',  ( -0.1264236179284866091, 0.03887795280966901967, 0.1264236179284866091 ) ) ;
#14247=CARTESIAN_POINT ( 'NONE',  ( -0.07405724077823318263, -1.268824755630812540, 0.1787899950787401604 ) ) ;
#14249=CARTESIAN_POINT ( 'NONE',  ( 0.1787899950787401604, -0.2982283464029296116, 0.07405724077823318263 ) ) ;
#14253=CARTESIAN_POINT ( 'NONE',  ( -0.2471922967771591484, -0.09275221067063765812, 0.04038134086896451314 ) ) ;
#14256=CARTESIAN_POINT ( 'NONE',  ( -0.07405724077823318263, -1.651574803095843258, 0.1787899950787401604 ) ) ;
#14259=CARTESIAN_POINT ( 'NONE',  ( -0.09722930128650188186, -0.09842519685039370636, 0.1314396626312874239 ) ) ;
#14281=ORIENTED_EDGE ( 'NONE', *, *, #45103, .F. ) ;
#14285=CARTESIAN_POINT ( 'NONE',  ( 0.1264236179284866091, 0.05364173233722803469, 0.1264236179284866091 ) ) ;
#14294=CARTESIAN_POINT ( 'NONE',  ( -0.1574803149606300301, 0.09793307097366882319, -0.06523048226347956391 ) ) ;
#14304=CARTESIAN_POINT ( 'NONE',  ( -0.1264236179284866091, -0.8086869603552225838, -0.1264236179284866091 ) ) ;
#14306=CARTESIAN_POINT ( 'NONE',  ( 0.04463444342724977310, -0.08956241828510866365, 0.1426423949953722625 ) ) ;
#14323=CARTESIAN_POINT ( 'NONE',  ( 0.1574803149606300301, -0.6008858267716538082, 0.06523048226347956391 ) ) ;
#14334=CARTESIAN_POINT ( 'NONE',  ( 0.07405724077823318263, -0.6820866141194646959, -0.1787899950787401604 ) ) ;
#14341=CARTESIAN_POINT ( 'NONE',  ( 0.1787899950787401882, -1.284940944828125930, -2.189545951927503898E-17 ) ) ;
#14342=CARTESIAN_POINT ( 'NONE',  ( -0.1574803149606300301, -1.486712598425197873, -0.06523048226347956391 ) ) ;
#14346=ORIENTED_EDGE ( 'NONE', *, *, #7469, .F. ) ;
#14347=CARTESIAN_POINT ( 'NONE',  ( 0.06523048226347956391, -1.422736220364914095, 0.1574803149606297803 ) ) ;
#14354=CARTESIAN_POINT ( 'NONE',  ( -0.1850060400416962680, 0.08128102204192841351, -0.1786197838463617626 ) ) ;
#14358=CARTESIAN_POINT ( 'NONE',  ( 0.07405724077823318263, -0.4223680627174279945, -0.1787899950787401604 ) ) ;
#14359=CARTESIAN_POINT ( 'NONE',  ( -0.1563790690919384108, -0.09842519685039370636, -0.08631298726982068736 ) ) ;
#14370=CARTESIAN_POINT ( 'NONE',  ( -0.1787899950787401882, -1.225885826717889815, 0.000000000000000000 ) ) ;
#14371=CARTESIAN_POINT ( 'NONE',  ( 0.1787899950787401604, -1.321850393647023392, 0.07405724077823318263 ) ) ;
#14376=CARTESIAN_POINT ( 'NONE',  ( -0.1113553986120547346, -0.1013779527559055121, 0.1113553986120547346 ) ) ;
#14386=CARTESIAN_POINT ( 'NONE',  ( -0.1787899950787401882, -0.07923228341080354453, 0.000000000000000000 ) ) ;
#14388=CARTESIAN_POINT ( 'NONE',  ( -0.1574803149606300301, -1.555610236112946021, -0.06523048226347956391 ) ) ;
#14389=CARTESIAN_POINT ( 'NONE',  ( 0.1787899950787401882, -0.8124999999462361178, -2.189545951927503898E-17 ) ) ;
#14391=CARTESIAN_POINT ( 'NONE',  ( -0.06523048226347956391, -1.019192913385827293, -0.1574803149606300301 ) ) ;
#14394=( BOUNDED_CURVE ( )  B_SPLINE_CURVE ( 2, ( #12833, #24084, #17343, #31977, #9217, #20468, #42715, #46565, #17107, #31748, #9931, #28389, #8311, #45857, #33989, #1115, #35104, #15775, #2250, #27927, #13299, #31514, #31048, #23836, #11119, #3670, #21893, #3439, #18293, #28879, #29125, #21405, #32220, #25250, #46805, #43916, #32934, #7029, #14238, #22113, #10165, #297, #36738, #24773, #13990, #47289, #28640, #21655, #39371, #55, #36515, #10409, #14701, #39840, #25738, #25012, #43439, #43199, #3898, #36287, #40311, #29376, #14944, #10645, #39610, #18052, #33176, #6786, #36031, #40076, #25507, #3192, #7493, #32699, #42958, #43678, #18523, #17820, #7275, #6555, #21165, #35797, #14467, #2941, #32467, #47045, #17578, #10888, #29827, #26441, #524, #34334, #1465 ),
 .UNSPECIFIED., .F., .T. ) 
 B_SPLINE_CURVE_WITH_KNOTS ( ( 3, 2, 2, 2, 2, 2, 2, 2, 2, 2, 2, 2, 2, 2, 2, 2, 2, 2, 2, 2, 2, 2, 2, 2, 2, 2, 2, 2, 2, 2, 2, 2, 2, 2, 2, 2, 2, 2, 2, 2, 2, 2, 2, 2, 2, 2, 3 ),
 ( 0.000000000000000000, 0.01120958318856041767, 0.03362875003688474418, 0.05604791688520911058, 0.07846708373353343535, 0.1008862505818577671, 0.1233054174301821265, 0.1457245842785064582, 0.1681437511268307761, 0.1905629179751551494, 0.2129820848234795228, 0.2354012516718038128, 0.2578204185201281584, 0.2802395853684525040, 0.3026587522167768496, 0.3250779190651011952, 0.3474970859134255963, 0.3699162527617498308, 0.3923354196100741764, 0.4147545864583985220, 0.4371737533067229231, 0.4595929201550472687, 0.4820120870033716143, 0.5044312538516959599, 0.5268504207000203055, 0.5492695875483445400, 0.5716887543966688856, 0.5941079212449933422, 0.6165270880933176878, 0.6389462549416420334, 0.6613654217899663790, 0.6837845886382906135, 0.7062037554866149591, 0.7286229223349393047, 0.7510420891832636503, 0.7734612560315881069, 0.7958804228799124525, 0.8182995897282366871, 0.8407187565765610326, 0.8631379234248853782, 0.8855570902732097238, 0.9079762571215340694, 0.9303954239698584150, 0.9528145908181826496, 0.9752337576665071062, 0.9976529245148314518, 1.000000000000000000 ),
 .UNSPECIFIED. ) 
 CURVE ( )  GEOMETRIC_REPRESENTATION_ITEM ( )  RATIONAL_B_SPLINE_CURVE ( ( 0.9619397662556434803, 0.9619397670555891455, 1.000000000000000000, 0.9238795325112869605, 1.000000000000000000, 0.9238795325112869605, 1.000000000000000000, 0.9238795325112869605, 1.000000000000000000, 0.9238795325112869605, 1.000000000000000000, 0.9238795325112869605, 1.000000000000000000, 0.9238795325112869605, 1.000000000000000000, 0.9238795325112869605, 1.000000000000000000, 0.9238795325112869605, 1.000000000000000000, 0.9238795325112869605, 1.000000000000000000, 0.9238795325112869605, 1.000000000000000000, 0.9238795325112869605, 1.000000000000000000, 0.9238795325112869605, 1.000000000000000000, 0.9238795325112869605, 1.000000000000000000, 0.9238795325112869605, 1.000000000000000000, 0.9238795325112869605, 1.000000000000000000, 0.9238795325112869605, 1.000000000000000000, 0.9238795325112869605, 1.000000000000000000, 0.9238795325112869605, 1.000000000000000000, 0.9238795325112869605, 1.000000000000000000, 0.9238795325112869605, 1.000000000000000000, 0.9238795325112869605, 1.000000000000000000, 0.9238795325112869605, 1.000000000000000000, 0.9238795325112869605, 1.000000000000000000, 0.9238795325112869605, 1.000000000000000000, 0.9238795325112869605, 1.000000000000000000, 0.9238795325112869605, 1.000000000000000000, 0.9238795325112869605, 1.000000000000000000, 0.9238795325112869605, 1.000000000000000000, 0.9238795325112869605, 1.000000000000000000, 0.9238795325112869605, 1.000000000000000000, 0.9238795325112869605, 1.000000000000000000, 0.9238795325112869605, 1.000000000000000000, 0.9238795325112869605, 1.000000000000000000, 0.9238795325112869605, 1.000000000000000000, 0.9238795325112869605, 1.000000000000000000, 0.9238795325112869605, 1.000000000000000000, 0.9238795325112869605, 1.000000000000000000, 0.9238795325112869605, 1.000000000000000000, 0.9238795325112869605, 1.000000000000000000, 0.9238795325112869605, 1.000000000000000000, 0.9238795325112869605, 1.000000000000000000, 0.9238795325112869605, 1.000000000000000000, 0.9238795325112869605, 1.000000000000000000, 0.9238795325112869605, 1.000000000000000000, 0.9920309044323080139, 0.9857303872709801684 ) ) 
 REPRESENTATION_ITEM ( '' )  ) ;
#14402=CARTESIAN_POINT ( 'NONE',  ( 0.06523048226347956391, -1.265255905404284453, 0.1574803149606297803 ) ) ;
#14411=CARTESIAN_POINT ( 'NONE',  ( 0.1574803149606300301, -0.2367125983176700255, 0.06523048226347956391 ) ) ;
#14420=CARTESIAN_POINT ( 'NONE',  ( -0.1787899950787401604, -1.672368062717427106, -0.07405724077823318263 ) ) ;
#14424=CARTESIAN_POINT ( 'NONE',  ( 0.1787899950787401604, -0.9281496062454495100, 0.07405724077823318263 ) ) ;
#14429=CARTESIAN_POINT ( 'NONE',  ( -0.1797182628040039087, -0.1560477465909194950, 0.07444174185955065859 ) ) ;
#14430=CARTESIAN_POINT ( 'NONE',  ( 0.1264236179284866091, -0.1492381414575852383, -0.1264236179284866091 ) ) ;
#14431=CARTESIAN_POINT ( 'NONE',  ( -0.1264236179284866091, -0.2711614172690712810, 0.1264236179284866091 ) ) ;
#14437=CARTESIAN_POINT ( 'NONE',  ( -1.100456976456230270E-17, -1.782524124543677368, -0.1797182628040039365 ) ) ;
#14445=CARTESIAN_POINT ( 'NONE',  ( -0.1787899950787401604, -0.1998031495525358359, 0.07405724077823318263 ) ) ;
#14448=CARTESIAN_POINT ( 'NONE',  ( 0.1264236179284866091, -1.048720472387181024, 0.1264236179284866091 ) ) ;
#14467=CARTESIAN_POINT ( 'NONE',  ( 0.1264236179284866091, -0.06938976372576398377, 0.1264236179284866091 ) ) ;
#14476=CARTESIAN_POINT ( 'NONE',  ( 0.07405724077823318263, -1.327879873741049765, -0.1787899950787401604 ) ) ;
#14478=CARTESIAN_POINT ( 'NONE',  ( -0.1264236179284866091, -0.2416338582139531399, -0.1264236179284866091 ) ) ;
#14482=CARTESIAN_POINT ( 'NONE',  ( -0.2471889898701305766, -0.06575181108605680780, 0.09853485309532654390 ) ) ;
#14485=CARTESIAN_POINT ( 'NONE',  ( -0.07405724077823318263, -1.740157480261197875, -0.1787899950787401604 ) ) ;
#14489=CARTESIAN_POINT ( 'NONE',  ( 0.07444174185955065859, -1.248567431630288826, 0.1797182628040039087 ) ) ;
#14495=LINE ( 'NONE', #25539, #8244 ) ;
#14496=CARTESIAN_POINT ( 'NONE',  ( 0.000000000000000000, -0.09842519685039370636, 0.000000000000000000 ) ) ;
#14517=CARTESIAN_POINT ( 'NONE',  ( 3.284318927891251994E-17, -0.06938976372576398377, 0.1787899950787401882 ) ) ;
#14518=ORIENTED_EDGE ( 'NONE', *, *, #582, .T. ) ;
#14527=CARTESIAN_POINT ( 'NONE',  ( 0.1264236179284866091, -1.801673228292693052, 0.1264236179284866091 ) ) ;
#14536=CARTESIAN_POINT ( 'NONE',  ( 0.07405724077823318263, -0.8948090075993178072, -0.1787899950787401604 ) ) ;
#14537=CARTESIAN_POINT ( 'NONE',  ( -0.1371053627424283494, -0.08956161432658386878, 0.08897719781895610525 ) ) ;
#14539=CARTESIAN_POINT ( 'NONE',  ( -0.07405724077823318263, 0.1102362205262043815, -0.1787899950787401604 ) ) ;
#14547=CARTESIAN_POINT ( 'NONE',  ( 0.1270800023317771588, -0.8031934158822577885, -0.1270800023317771588 ) ) ;
#14552=CARTESIAN_POINT ( 'NONE',  ( -9.642888182262618425E-18, -0.6279527559055118058, -0.1574803149606299191 ) ) ;
#14560=CARTESIAN_POINT ( 'NONE',  ( -0.1113553986120547346, -0.6131889762704252345, -0.1113553986120547346 ) ) ;
#14571=CARTESIAN_POINT ( 'NONE',  ( 0.1574803149606300301, -1.506397637795275024, 0.06523048226347956391 ) ) ;
#14574=CARTESIAN_POINT ( 'NONE',  ( 0.06523048226347956391, 0.1176181102362204994, -0.1574803149606297803 ) ) ;
#14576=CARTESIAN_POINT ( 'NONE',  ( -0.1574803149606300301, -0.3351377951680634681, -0.06523048226347956391 ) ) ;
#14578=EDGE_CURVE ( 'NONE', #36213, #26985, #35222, .T. ) ;
#14581=CARTESIAN_POINT ( 'NONE',  ( -0.2471922904502827645, 0.08571147543119535250, 0.06121067491482544420 ) ) ;
#14584=CARTESIAN_POINT ( 'NONE',  ( 0.08643384275326014554, 0.09202339627320528515, -0.2355304684854532260 ) ) ;
#14586=CARTESIAN_POINT ( 'NONE',  ( -0.1787899950787401604, -0.4125255430323886419, -0.07405724077823318263 ) ) ;
#14587=CARTESIAN_POINT ( 'NONE',  ( -0.1189464023891061012, -0.09842519685039370636, 0.1140809237429826761 ) ) ;
#14593=CARTESIAN_POINT ( 'NONE',  ( 0.2471902452994138577, -0.09796597228571109206, 0.01325394226265646895 ) ) ;
#14597=CARTESIAN_POINT ( 'NONE',  ( 0.1787899950787401604, -1.169291338528914537, 0.07405724077823318263 ) ) ;
#14598=CARTESIAN_POINT ( 'NONE',  ( 0.1787899950787401604, -1.439960629867495401, 0.07405724077823318263 ) ) ;
#14604=CARTESIAN_POINT ( 'NONE',  ( -0.1574803149606300301, -0.1481299212598424508, -0.06523048226347956391 ) ) ;
#14619=CARTESIAN_POINT ( 'NONE',  ( -0.06523048226347956391, 0.1077755906587081480, 0.1574803149606297803 ) ) ;
#14620=CARTESIAN_POINT ( 'NONE',  ( 3.284318927891251994E-17, -1.565452755851747924, 0.1787899950787401882 ) ) ;
#14621=CARTESIAN_POINT ( 'NONE',  ( -0.1113553986120547346, -1.548228346349165285, 0.1113553986120547346 ) ) ;
#14622=CARTESIAN_POINT ( 'NONE',  ( 0.1264236179284866091, -0.7682086613635590311, -0.1264236179284866091 ) ) ;
#14625=CARTESIAN_POINT ( 'NONE',  ( -0.06523048226347956391, -1.004429133858267598, 0.1574803149606297803 ) ) ;
#14633=ORIENTED_EDGE ( 'NONE', *, *, #32550, .F. ) ;
#14646=CARTESIAN_POINT ( 'NONE',  ( -0.1407580821002830940, -0.09851383941439428860, -0.1134402804189334618 ) ) ;
#14655=VECTOR ( 'NONE', #33738, 39.37007874015748143 ) ;
#14657=CARTESIAN_POINT ( 'NONE',  ( -0.1264236179284866091, -0.8715551180564724554, -0.1264236179284866091 ) ) ;
#14658=CARTESIAN_POINT ( 'NONE',  ( -0.2471922732848683135, -0.07885118474262710342, -0.07559718168567093610 ) ) ;
#14661=CARTESIAN_POINT ( 'NONE',  ( -0.1270800023317771588, -0.1142170379295021632, 0.1270800023317771588 ) ) ;
#14662=CARTESIAN_POINT ( 'NONE',  ( -0.1787899950787401604, -0.1320137320087663158, 0.07405724077823318263 ) ) ;
#14663=CARTESIAN_POINT ( 'NONE',  ( -0.1787899950787401604, -0.3129921259304885850, 0.07405724077823318263 ) ) ;
#14664=CARTESIAN_POINT ( 'NONE',  ( -1.094772975963752103E-17, -0.09399606293836239301, -0.1787899950787401882 ) ) ;
#14665=CARTESIAN_POINT ( 'NONE',  ( 0.2471922931865138395, -0.07794380098771452881, -0.07736948232533663594 ) ) ;
#14672=CARTESIAN_POINT ( 'NONE',  ( 0.000000000000000000, 0.09842519685039370636, 0.000000000000000000 ) ) ;
#14675=CARTESIAN_POINT ( 'NONE',  ( -0.1854358583624131085, -0.08093302715482435239, 0.1783713581464878017 ) ) ;
#14680=CARTESIAN_POINT ( 'NONE',  ( 0.1264236179284866091, -0.3449803149068665364, 0.1264236179284866091 ) ) ;
#14683=CARTESIAN_POINT ( 'NONE',  ( -1.094772975963752103E-17, -1.073326771599779628, -0.1787899950787401882 ) ) ;
#14691=CARTESIAN_POINT ( 'NONE',  ( -0.06523048226347956391, -1.127460629813733295, -0.1574803149606300301 ) ) ;
#14701=CARTESIAN_POINT ( 'NONE',  ( 3.284318927891251994E-17, 0.004429133912031243958, 0.1787899950787401882 ) ) ;
#14708=CARTESIAN_POINT ( 'NONE',  ( 0.1264236179284866091, -1.251600346181994228, -0.1264236179284866091 ) ) ;
#14710=CARTESIAN_POINT ( 'NONE',  ( -0.1787899950787401882, -0.3548228345919058890, 0.000000000000000000 ) ) ;
#14716=EDGE_CURVE ( 'NONE', #47206, #7112, #25745, .T. ) ;
#14717=CARTESIAN_POINT ( 'NONE',  ( -0.2471922904502826812, -0.04197619597928321789, 0.1314166662981948452 ) ) ;
#14721=CARTESIAN_POINT ( 'NONE',  ( -0.1264236179284866091, -1.703248031442299304, -0.1264236179284866091 ) ) ;
#14722=CARTESIAN_POINT ( 'NONE',  ( -0.1264236179284866091, -1.658956692859621995, -0.1264236179284866091 ) ) ;
#14725=CARTESIAN_POINT ( 'NONE',  ( -0.1401001227007565297, -0.09842519685039370636, 0.09069709532487360559 ) ) ;
#14726=CARTESIAN_POINT ( 'NONE',  ( -0.1270800023317771588, -1.452799715094856392, 0.1270800023317771588 ) ) ;
#14735=CARTESIAN_POINT ( 'NONE',  ( -0.06523048226347956391, -0.7731299211523151582, -0.1574803149606300301 ) ) ;
#14754=CARTESIAN_POINT ( 'NONE',  ( 0.1787899950787401882, -0.2170275590013547307, -2.189545951927503898E-17 ) ) ;
#14755=ORIENTED_EDGE ( 'NONE', *, *, #38581, .F. ) ;
#14764=CARTESIAN_POINT ( 'NONE',  ( 0.1574803149606300301, 0.04379921270595223126, -0.06523048226347956391 ) ) ;
#14771=EDGE_CURVE ( 'NONE', #34774, #36271, #38593, .T. ) ;
#14775=CARTESIAN_POINT ( 'NONE',  ( 0.07405724077823318263, -0.7914625509064031617, 0.1787899950787401604 ) ) ;
#14778=CARTESIAN_POINT ( 'NONE',  ( -1.094772975963752103E-17, 0.1471456693451021758, -0.1787899950787401882 ) ) ;
#14791=CARTESIAN_POINT ( 'NONE',  ( -0.1270800023317771588, -0.9016186127326516475, 0.1270800023317771588 ) ) ;
#14806=CARTESIAN_POINT ( 'NONE',  ( -0.07405724077823318263, -0.7805118109698575557, 0.1787899950787401604 ) ) ;
#14811=CARTESIAN_POINT ( 'NONE',  ( -0.1574803149606299191, -1.720472440944881942, 0.000000000000000000 ) ) ;
#14825=CARTESIAN_POINT ( 'NONE',  ( -1.094772975963752103E-17, -0.4592775115363252336, -0.1787899950787401882 ) ) ;
#14826=CARTESIAN_POINT ( 'NONE',  ( -0.2128335240989271959, -0.08955970507752815390, -0.1176384946248013735 ) ) ;
#14836=CARTESIAN_POINT ( 'NONE',  ( 0.1264236179284866091, -1.398129921206078707, -0.1264236179284866091 ) ) ;
#14837=CARTESIAN_POINT ( 'NONE',  ( -1.094772975963752103E-17, -1.348917322780881944, -0.1787899950787401882 ) ) ;
#14842=CARTESIAN_POINT ( 'NONE',  ( 0.1270800023317771588, -0.6063430221814705146, -0.1270800023317771588 ) ) ;
#14847=CARTESIAN_POINT ( 'NONE',  ( -0.1574803149606297803, -0.3400590551181101318, 0.06523048226347956391 ) ) ;
#14861=CARTESIAN_POINT ( 'NONE',  ( -0.1113553986120547346, 0.09547244105240886014, -0.1113553986120547346 ) ) ;
#14863=CARTESIAN_POINT ( 'NONE',  ( -0.1264236179284866091, -1.580216535379306952, -0.1264236179284866091 ) ) ;
#14864=CARTESIAN_POINT ( 'NONE',  ( -0.1113553986120547346, -1.518700787294047005, -0.1113553986120547346 ) ) ;
#14865=CARTESIAN_POINT ( 'NONE',  ( -0.1787899950787401604, -0.7903543306548983516, 0.07405724077823318263 ) ) ;
#14866=CARTESIAN_POINT ( 'NONE',  ( 2.892866454678787531E-17, -1.080708661417322913, 0.1574803149606299191 ) ) ;
#14882=CARTESIAN_POINT ( 'NONE',  ( 0.1179171413540825442, 0.09842519685039370636, 0.2173535775632911005 ) ) ;
#14894=AXIS2_PLACEMENT_3D ( 'NONE', #10958, #36364, #47119 ) ;
#14900=CARTESIAN_POINT ( 'NONE',  ( -0.07405724077823318263, -0.3917322834108032947, 0.1787899950787401604 ) ) ;
#14901=CARTESIAN_POINT ( 'NONE',  ( -0.1264236179284866091, -0.9109251967966299768, -0.1264236179284866091 ) ) ;
#14906=CARTESIAN_POINT ( 'NONE',  ( -0.07444174185955065859, -0.2692367229688725216, 0.1797182628040039087 ) ) ;
#14907=CARTESIAN_POINT ( 'NONE',  ( -0.07405724077823318263, -0.03740157474938609478, 0.1787899950787401604 ) ) ;
#14908=CARTESIAN_POINT ( 'NONE',  ( 0.2471922904502827090, -0.09842519685039370636, -0.01321092903673363843 ) ) ;
#14920=CARTESIAN_POINT ( 'NONE',  ( 0.06523048226347956391, -0.9502952754830243931, 0.1574803149606297803 ) ) ;
#14921=CARTESIAN_POINT ( 'NONE',  ( 0.1264236179284866091, -0.2563976377415121966, -0.1264236179284866091 ) ) ;
#14924=CARTESIAN_POINT ( 'NONE',  ( -0.07405724077823318263, -1.056102362150961982, 0.1787899950787401604 ) ) ;
#14928=EDGE_LOOP ( 'NONE', ( #25651, #18758, #18437 ) ) ;
#14934=CARTESIAN_POINT ( 'NONE',  ( 0.1574803149606299191, -1.179133858160189119, -1.928577636452523993E-17 ) ) ;
#14944=CARTESIAN_POINT ( 'NONE',  ( 0.1264236179284866091, -0.02017716530056720692, -0.1264236179284866091 ) ) ;
#14953=CARTESIAN_POINT ( 'NONE',  ( 0.1787899950787401604, -1.416462550906403939, 0.07405724077823318263 ) ) ;
#14955=CARTESIAN_POINT ( 'NONE',  ( -0.1264236179284866091, -0.2711614172690712810, 0.1264236179284866091 ) ) ;
#14957=CARTESIAN_POINT ( 'NONE',  ( -0.1113553986120547346, 0.02657480325713335034, 0.1113553986120547346 ) ) ;
#14962=DIRECTION ( 'NONE',  ( 0.000000000000000000, 0.000000000000000000, 1.000000000000000000 ) ) ;
#14970=CARTESIAN_POINT ( 'NONE',  ( -0.1787899950787401604, -1.582677165300567346, -0.07405724077823318263 ) ) ;
#14971=CARTESIAN_POINT ( 'NONE',  ( 0.1264236179284866091, -1.718011810969858333, 0.1264236179284866091 ) ) ;
#14974=CARTESIAN_POINT ( 'NONE',  ( 0.07444174185955065859, -1.406047746590921133, 0.1797182628040039087 ) ) ;
#14980=CARTESIAN_POINT ( 'NONE',  ( 0.06841996760812382727, 0.1299212598425196763, 0.1651804176431311000 ) ) ;
#14982=CARTESIAN_POINT ( 'NONE',  ( 0.1574803149606300301, -0.8223425195775115881, -0.06523048226347956391 ) ) ;
#14998=CARTESIAN_POINT ( 'NONE',  ( -0.1270800023317771588, 0.1220034345114427293, 0.1270800023317771588 ) ) ;
#15006=CARTESIAN_POINT ( 'NONE',  ( -0.07405724077823318263, -0.2293307086076536994, 0.1787899950787401604 ) ) ;
#15007=ORIENTED_EDGE ( 'NONE', *, *, #586, .F. ) ;
#15009=CARTESIAN_POINT ( 'NONE',  ( 0.2275913475568078770, -0.05179116514251743547, -0.1540331450889871889 ) ) ;
#15014=CARTESIAN_POINT ( 'NONE',  ( 0.1574803149606300301, 0.08316929144610965552, -0.06523048226347956391 ) ) ;
#15019=EDGE_CURVE ( 'NONE', #38566, #26779, #14394, .T. ) ;
#15022=CARTESIAN_POINT ( 'NONE',  ( 0.1787899950787401604, -0.9046515272843580480, 0.07405724077823318263 ) ) ;
#15033=CARTESIAN_POINT ( 'NONE',  ( -0.07405724077823318263, -0.4852362204186770889, -0.1787899950787401604 ) ) ;
#15035=CARTESIAN_POINT ( 'NONE',  ( 0.1270800023317771588, -0.9606737308428878741, -0.1270800023317771588 ) ) ;
#15043=DIRECTION ( 'NONE',  ( 1.776356839400250070E-15, 0.000000000000000000, 1.000000000000000000 ) ) ;
#15047=CARTESIAN_POINT ( 'NONE',  ( -0.07405724077823318263, -0.7165354330171036512, -0.1787899950787401604 ) ) ;
#15054=CARTESIAN_POINT ( 'NONE',  ( 0.06523048226347956391, -1.732775590551180134, -0.1574803149606300301 ) ) ;
#15061=CARTESIAN_POINT ( 'NONE',  ( 0.1787899950787401604, -1.439960629867495401, -0.07405724077823318263 ) ) ;
#15068=CARTESIAN_POINT ( 'NONE',  ( 0.04076295239693379646, 0.06762482675903873364, -0.2618985693268080506 ) ) ;
#15069=FACE_OUTER_BOUND ( 'NONE', #42876, .T. ) ;
#15070=CARTESIAN_POINT ( 'NONE',  ( 0.1787899950787401604, -0.3485491650796322949, -0.07405724077823318263 ) ) ;
#15071=CARTESIAN_POINT ( 'NONE',  ( -0.1917820371396724566, -0.08955957972813564927, -0.1527325450606088486 ) ) ;
#15073=DIRECTION ( 'NONE',  ( -0.4999999999999998890, 0.000000000000000000, 0.8660254037844388186 ) ) ;
#15082=CARTESIAN_POINT ( 'NONE',  ( -0.1787899950787401604, -1.307086614119465695, -0.07405724077823318263 ) ) ;
#15083=CARTESIAN_POINT ( 'NONE',  ( 0.1264236179284866091, -1.471948818843874074, -0.1264236179284866091 ) ) ;
#15091=CARTESIAN_POINT ( 'NONE',  ( 0.1113553986120547346, -0.2391732283464566844, -0.1113553986120547346 ) ) ;
#15094=CARTESIAN_POINT ( 'NONE',  ( -0.1264236179284866091, -0.2071850393163153503, -0.1264236179284866091 ) ) ;
#15101=CARTESIAN_POINT ( 'NONE',  ( -0.1337103929845034622, -0.08955973559652113947, 0.09286901502511588080 ) ) ;
#15103=EDGE_LOOP ( 'NONE', ( #3492, #17210, #42277 ) ) ;
#15106=CARTESIAN_POINT ( 'NONE',  ( -0.07405724077823318263, -1.567913385773008095, 0.1787899950787401604 ) ) ;
#15107=CARTESIAN_POINT ( 'NONE',  ( -0.1787899950787401604, -0.6771653542769455747, -0.07405724077823318263 ) ) ;
#15108=CARTESIAN_POINT ( 'NONE',  ( -0.06523048226347956391, -1.161909448818897461, 0.1574803149606297803 ) ) ;
#15132=CARTESIAN_POINT ( 'NONE',  ( 0.06901435990846417623, -0.09851382358029528441, 0.1342407315491202791 ) ) ;
#15136=ORIENTED_EDGE ( 'NONE', *, *, #18130, .F. ) ;
#15138=CARTESIAN_POINT ( 'NONE',  ( -0.1787899950787401604, -0.8690944881352120621, 0.07405724077823318263 ) ) ;
#15139=CARTESIAN_POINT ( 'NONE',  ( 0.1264236179284866091, -0.3745078739619845942, -0.1264236179284866091 ) ) ;
#15140=CARTESIAN_POINT ( 'NONE',  ( 0.07405724077823318263, -1.036417322780882833, -0.1787899950787401604 ) ) ;
#15144=CARTESIAN_POINT ( 'NONE',  ( 3.301370929368692659E-17, -0.1486658568271399528, 0.1797182628040039365 ) ) ;
#15146=CARTESIAN_POINT ( 'NONE',  ( 0.1264236179284866091, -0.03001968498560653523, 0.1264236179284866091 ) ) ;
#15160=CARTESIAN_POINT ( 'NONE',  ( 0.1787899950787401604, -0.3375984251430867999, -0.07405724077823318263 ) ) ;
#15162=CARTESIAN_POINT ( 'NONE',  ( 0.07405724077823318263, -1.169291338528914537, 0.1787899950787401604 ) ) ;
#15172=CARTESIAN_POINT ( 'NONE',  ( 0.06523048226347956391, -1.211122047136568236, -0.1574803149606300301 ) ) ;
#15188=CARTESIAN_POINT ( 'NONE',  ( -0.07405724077823318263, -1.465675149331600480, 0.1787899950787401604 ) ) ;
#15190=CARTESIAN_POINT ( 'NONE',  ( -0.1264236179284866091, -0.3991141731745826982, -0.1264236179284866091 ) ) ;
#15198=CARTESIAN_POINT ( 'NONE',  ( -0.1787899950787401604, -1.700787401521039355, -0.07405724077823318263 ) ) ;
#15199=CARTESIAN_POINT ( 'NONE',  ( 0.1787899950787401604, -1.754921259788755128, 0.07405724077823318263 ) ) ;
#15205=CARTESIAN_POINT ( 'NONE',  ( -0.1270800023317771588, -1.374059557614541349, 0.1270800023317771588 ) ) ;
#15213=CARTESIAN_POINT ( 'NONE',  ( 0.1264236179284866091, 0.1373031496600628232, -0.1264236179284866091 ) ) ;
#15216=EDGE_CURVE ( 'NONE', #37608, #44070, #34004, .T. ) ;
#15227=CARTESIAN_POINT ( 'NONE',  ( 0.1270800023317771588, -0.01579184107910856436, -0.1270800023317771588 ) ) ;
#15229=CARTESIAN_POINT ( 'NONE',  ( -0.1264236179284866091, -1.152066929080094448, -0.1264236179284866091 ) ) ;
#15238=CARTESIAN_POINT ( 'NONE',  ( 0.07405724077823318263, -0.1456692912848192578, 0.1787899950787401604 ) ) ;
#15240=CARTESIAN_POINT ( 'NONE',  ( -0.1113553986120547346, 0.08562992125984252023, -0.1113553986120547346 ) ) ;
#15241=CARTESIAN_POINT ( 'NONE',  ( -0.03810507699822204830, -0.06563552548610597503, 0.2634293601846930954 ) ) ;
#15244=CARTESIAN_POINT ( 'NONE',  ( 0.1574803149606300301, -0.03986220461688239070, 0.06523048226347956391 ) ) ;
#15251=CARTESIAN_POINT ( 'NONE',  ( -0.1264236179284866091, -0.9956948343709705052, 0.1264236179284866091 ) ) ;
#15262=CARTESIAN_POINT ( 'NONE',  ( -1.100456976456230270E-17, -1.073862707220840651, -0.1797182628040039365 ) ) ;
#15269=CARTESIAN_POINT ( 'NONE',  ( 2.892866454678787531E-17, 0.1102362205799679168, 0.1574803149606299191 ) ) ;
#15274=CARTESIAN_POINT ( 'NONE',  ( -0.1787899950787401604, -0.8297244093950564281, -0.07405724077823318263 ) ) ;
#15281=CARTESIAN_POINT ( 'NONE',  ( -9.642888182262618425E-18, -1.651574803149606474, -0.1574803149606299191 ) ) ;
#15284=FACE_BOUND ( 'NONE', #1299, .T. ) ;
#15293=CARTESIAN_POINT ( 'NONE',  ( 0.04878249046419585316, 0.07306521771081567196, -0.2572684868648978385 ) ) ;
#15295=CARTESIAN_POINT ( 'NONE',  ( -0.1787899950787401882, -0.6069153068119154115, 0.000000000000000000 ) ) ;
#15296=CARTESIAN_POINT ( 'NONE',  ( -0.1204886227201696774, -0.08955993428987342464, 0.1930813601014000069 ) ) ;
#15301=CARTESIAN_POINT ( 'NONE',  ( -0.1264236179284866091, -1.753568850119002098, -0.1264236179284866091 ) ) ;
#15307=CARTESIAN_POINT ( 'NONE',  ( -0.1787899950787401882, -1.304625984198204636, 0.000000000000000000 ) ) ;
#15309=CARTESIAN_POINT ( 'NONE',  ( 0.1264236179284866091, -1.511318897584031484, -0.1264236179284866091 ) ) ;
#15317=CARTESIAN_POINT ( 'NONE',  ( -9.642888182262618425E-18, -0.2736220472440945017, -0.1574803149606299191 ) ) ;
#15321=CARTESIAN_POINT ( 'NONE',  ( -0.1487246401439196453, -0.09667468234190848553, -0.09990315886301043280 ) ) ;
#15327=CARTESIAN_POINT ( 'NONE',  ( -0.1690507553807868990, -0.08956027919751255451, -0.02600493670471536872 ) ) ;
#15336=CARTESIAN_POINT ( 'NONE',  ( -0.1787899950787401604, -1.538385826717890703, -0.07405724077823318263 ) ) ;
#15337=CARTESIAN_POINT ( 'NONE',  ( -1.094772975963752103E-17, -0.8026574802611967652, -0.1787899950787401882 ) ) ;
#15338=CARTESIAN_POINT ( 'NONE',  ( -0.06523048226347956391, -1.137303149606299080, -0.1574803149606300301 ) ) ;
#15345=CARTESIAN_POINT ( 'NONE',  ( 0.1113553986120547346, -1.331692913278299084, -0.1113553986120547346 ) ) ;
#15355=CARTESIAN_POINT ( 'NONE',  ( 0.1235961452251413406, 0.09842519685039370636, 0.2140748031496062798 ) ) ;
#15362=CARTESIAN_POINT ( 'NONE',  ( 0.08192804256358189596, -0.09851382410610984297, 0.1254088401684838594 ) ) ;
#15370=CARTESIAN_POINT ( 'NONE',  ( 0.1787899950787401604, -0.8494094487651332459, -0.07405724077823318263 ) ) ;
#15372=CARTESIAN_POINT ( 'NONE',  ( 0.1264236179284866091, -1.048720472387181024, 0.1264236179284866091 ) ) ;
#15378=CARTESIAN_POINT ( 'NONE',  ( 0.1797182628040039087, -0.3381343607641479343, 0.07444174185955046430 ) ) ;
#15380=CARTESIAN_POINT ( 'NONE',  ( 0.1787899950787401604, -0.06692913380450424277, 0.07405724077823318263 ) ) ;
#15395=CARTESIAN_POINT ( 'NONE',  ( -0.1787899950787401604, -0.3179133857730082058, 0.07405724077823318263 ) ) ;
#15397=CARTESIAN_POINT ( 'NONE',  ( -0.1264236179284866091, -1.216043307032850462, 0.1264236179284866091 ) ) ;
#15407=CARTESIAN_POINT ( 'NONE',  ( -0.1393745452458122480, -0.09844044251944331081, -0.1120857077816562464 ) ) ;
#15416=CARTESIAN_POINT ( 'NONE',  ( -0.1819224463268279690, -0.09851385391904804445, -0.1710117998103236336 ) ) ;
#15424=CARTESIAN_POINT ( 'NONE',  ( 0.07405724077823318263, -1.382013732008767537, 0.1787899950787401604 ) ) ;
#15426=CARTESIAN_POINT ( 'NONE',  ( 3.284318927891251994E-17, -0.5024606298674960669, 0.1787899950787401882 ) ) ;
#15434=CARTESIAN_POINT ( 'NONE',  ( 0.07405724077823318263, -1.789370078686394194, -0.1787899950787401604 ) ) ;
#15435=CARTESIAN_POINT ( 'NONE',  ( -0.07405724077823318263, -1.622047244040725866, -0.1787899950787401604 ) ) ;
#15441=CARTESIAN_POINT ( 'NONE',  ( 0.06523048226347956391, -0.6845472440944881942, 0.1574803149606297803 ) ) ;
#15443=CARTESIAN_POINT ( 'NONE',  ( -0.07444174185955065859, -1.410969006433440365, 0.1797182628040039087 ) ) ;
#15445=CARTESIAN_POINT ( 'NONE',  ( 1.928577636452524610E-17, -0.09842519685039370636, -0.1574803149606299191 ) ) ;
#15468=CARTESIAN_POINT ( 'NONE',  ( -0.1270800023317771588, -0.03547688044918728689, 0.1270800023317771588 ) ) ;
#15469=CARTESIAN_POINT ( 'NONE',  ( 0.07405724077823318263, -1.292322834591905778, 0.1787899950787401604 ) ) ;
#15470=LINE ( 'NONE', #19274, #40119 ) ;
#15476=CARTESIAN_POINT ( 'NONE',  ( -0.1264236179284866091, -0.1136811023084411398, 0.1264236179284866091 ) ) ;
#15482=CARTESIAN_POINT ( 'NONE',  ( -0.1574803149606297803, -0.09399606288459895487, 0.06523048226347956391 ) ) ;
#15490=CARTESIAN_POINT ( 'NONE',  ( 3.284318927891251994E-17, -0.9514034957882933075, 0.1787899950787401882 ) ) ;
#15492=CARTESIAN_POINT ( 'NONE',  ( 0.1787899950787401604, 0.1003937008411650705, -0.07405724077823318263 ) ) ;
#15503=CARTESIAN_POINT ( 'NONE',  ( -0.1797182628040039087, -0.9877406599767465378, -0.07444174185955065859 ) ) ;
#15517=CARTESIAN_POINT ( 'NONE',  ( -0.1264236179284866091, -0.7436023621509606496, 0.1264236179284866091 ) ) ;
#15526=CARTESIAN_POINT ( 'NONE',  ( -0.1574803149606297803, -1.678641732283464583, 0.06523048226347956391 ) ) ;
#15536=CARTESIAN_POINT ( 'NONE',  ( 0.1787899950787401604, -1.597440944828127485, -0.07405724077823318263 ) ) ;
#15543=CARTESIAN_POINT ( 'NONE',  ( -0.1264236179284866091, -0.6118365666544350878, -0.1264236179284866091 ) ) ;
#15544=CARTESIAN_POINT ( 'NONE',  ( 0.03780438559997598841, -0.08956001823431022912, 0.2156824087300551196 ) ) ;
#15560=CARTESIAN_POINT ( 'NONE',  ( 0.1264236179284866091, -1.368602362150960650, 0.1264236179284866091 ) ) ;
#15561=CARTESIAN_POINT ( 'NONE',  ( 0.1787899950787401604, -1.518700787347811554, 0.07405724077823318263 ) ) ;
#15569=CARTESIAN_POINT ( 'NONE',  ( -0.1113553986120547346, -0.2982283464566929387, 0.1113553986120547346 ) ) ;
#15577=CARTESIAN_POINT ( 'NONE',  ( 0.1574803149606299191, -0.5492125983176693316, -1.928577636452523993E-17 ) ) ;
#15579=CARTESIAN_POINT ( 'NONE',  ( -0.1217943169637149825, -0.08954727061951725520, 0.1064691133493027853 ) ) ;
#15583=CARTESIAN_POINT ( 'NONE',  ( -0.1113553986120547346, -0.03248031496062991907, -0.1113553986120547346 ) ) ;
#15584=CARTESIAN_POINT ( 'NONE',  ( 0.1787899950787401604, -1.597440944828127485, 0.07405724077823318263 ) ) ;
#15585=CARTESIAN_POINT ( 'NONE',  ( 0.1787899950787401604, -0.8543307086076546986, 0.07405724077823318263 ) ) ;
#15586=CARTESIAN_POINT ( 'NONE',  ( -0.1574803149606300301, -1.211122047244094002, -0.06523048226347956391 ) ) ;
#15594=CARTESIAN_POINT ( 'NONE',  ( 0.1574803149606300301, -1.299704724301920855, 0.06523048226347956391 ) ) ;
#15608=CARTESIAN_POINT ( 'NONE',  ( -0.1818951543555252237, -0.09842519685039370636, -0.1709882076668135797 ) ) ;
#15616=CARTESIAN_POINT ( 'NONE',  ( -0.1264236179284866091, -0.9060039369541103005, 0.1264236179284866091 ) ) ;
#15617=CARTESIAN_POINT ( 'NONE',  ( 0.1787899950787401882, -1.083169291284818980, -2.189545951927503898E-17 ) ) ;
#15621=CARTESIAN_POINT ( 'NONE',  ( -0.1797182628040039365, -0.3947288489531244338, 0.000000000000000000 ) ) ;
#15634=CARTESIAN_POINT ( 'NONE',  ( 0.07405724077823318263, -0.3720472440407247561, -0.1787899950787401604 ) ) ;
#15637=CARTESIAN_POINT ( 'NONE',  ( 0.1264236179284866091, -1.206200787347811110, 0.1264236179284866091 ) ) ;
#15649=CARTESIAN_POINT ( 'NONE',  ( -0.1230701032824740720, -0.09842685872290869720, -0.1297086761450524928 ) ) ;
#15658=CARTESIAN_POINT ( 'NONE',  ( -0.09073039027163543047, -0.09851385255785906347, -0.2376265320636606060 ) ) ;
#15665=CARTESIAN_POINT ( 'NONE',  ( -0.07405724077823318263, -1.505045228071758778, 0.1787899950787401604 ) ) ;
#15668=CARTESIAN_POINT ( 'NONE',  ( -0.1787899950787401882, -0.3941929133320630219, 0.000000000000000000 ) ) ;
#15672=EDGE_CURVE ( 'NONE', #19219, #6112, #19138, .T. ) ;
#15673=FACE_OUTER_BOUND ( 'NONE', #46744, .T. ) ;
#15678=CARTESIAN_POINT ( 'NONE',  ( 0.1787899950787401882, 0.1214311498809974438, -2.189545951927503898E-17 ) ) ;
#15684=CARTESIAN_POINT ( 'NONE',  ( -0.1574803149606300301, -0.7386811023622060768, -0.06523048226347956391 ) ) ;
#15686=CARTESIAN_POINT ( 'NONE',  ( 0.1797182628040039087, -1.356835148165722371, -0.07444174185955065859 ) ) ;
#15692=AXIS2_PLACEMENT_3D ( 'NONE', #23339, #22619, #11613 ) ;
#15697=CARTESIAN_POINT ( 'NONE',  ( -0.1264236179284866091, 0.1176181102899840625, 0.1264236179284866091 ) ) ;
#15709=CARTESIAN_POINT ( 'NONE',  ( 0.07444174185955046430, -0.01333121115784871406, -0.1797182628040039087 ) ) ;
#15710=CARTESIAN_POINT ( 'NONE',  ( 0.1113553986120547346, -1.056102362097196989, -0.1113553986120547346 ) ) ;
#15711=CARTESIAN_POINT ( 'NONE',  ( 0.07405724077823318263, -1.159448818843874074, -0.1787899950787401604 ) ) ;
#15720=CARTESIAN_POINT ( 'NONE',  ( -0.2471922904502826812, -0.09842519685039370636, -0.1427165354330708902 ) ) ;
#15723=CARTESIAN_POINT ( 'NONE',  ( -0.06523048226347956391, -0.04970472430192178492, 0.1574803149606297803 ) ) ;
#15731=DIRECTION ( 'NONE',  ( 0.000000000000000000, 1.000000000000000000, 0.000000000000000000 ) ) ;
#15732=CARTESIAN_POINT ( 'NONE',  ( 0.1264236179284866091, -1.015379873741049099, -0.1264236179284866091 ) ) ;
#15734=CARTESIAN_POINT ( 'NONE',  ( -0.1264236179284866091, 0.004429133912031228346, 0.1264236179284866091 ) ) ;
#15741=CARTESIAN_POINT ( 'NONE',  ( 0.000000000000000000, 0.09842519685039370636, 0.000000000000000000 ) ) ;
#15742=CARTESIAN_POINT ( 'NONE',  ( -0.07405724077823318263, -0.5492125983714331028, 0.1787899950787401604 ) ) ;
#15745=CARTESIAN_POINT ( 'NONE',  ( -0.07444174185955065859, -0.9532918410791076935, -0.1797182628040039087 ) ) ;
#15746=CARTESIAN_POINT ( 'NONE',  ( 0.1502195169528062479, 0.1299212598425197041, -0.07817644135598977861 ) ) ;
#15754=CARTESIAN_POINT ( 'NONE',  ( -0.06523048226347956391, -0.6943897636720013367, -0.1574803149606300301 ) ) ;
#15755=CARTESIAN_POINT ( 'NONE',  ( 0.1787899950787401604, 0.1003937008411650705, -0.07405724077823318263 ) ) ;
#15760=CARTESIAN_POINT ( 'NONE',  ( 0.1264236179284866091, -0.8124999999462361178, 0.1264236179284866091 ) ) ;
#15765=CARTESIAN_POINT ( 'NONE',  ( 0.1113553986120547346, -1.725393700679874076, -0.1113553986120547346 ) ) ;
#15770=CARTESIAN_POINT ( 'NONE',  ( -9.642888182262618425E-18, -1.690944881889763884, -0.1574803149606299191 ) ) ;
#15775=CARTESIAN_POINT ( 'NONE',  ( 0.1787899950787401604, 0.09055118115612578733, 0.07405724077823318263 ) ) ;
#15777=CARTESIAN_POINT ( 'NONE',  ( -0.07405724077823318263, -1.548228346402928723, -0.1787899950787401604 ) ) ;
#15787=CARTESIAN_POINT ( 'NONE',  ( -0.1264236179284866091, -0.5626239682292386579, 0.1264236179284866091 ) ) ;
#15788=CARTESIAN_POINT ( 'NONE',  ( -0.1891223223152169453, -0.08955981945756850970, 0.1329000297558324828 ) ) ;
#15798=CARTESIAN_POINT ( 'NONE',  ( -0.07405724077823318263, -1.375984251914741163, 0.1787899950787401604 ) ) ;
#15799=CARTESIAN_POINT ( 'NONE',  ( -0.1264236179284866091, -1.540846456639149542, -0.1264236179284866091 ) ) ;
#15804=CARTESIAN_POINT ( 'NONE',  ( -0.1574803149606300301, -0.2662401574803150983, -0.06523048226347956391 ) ) ;
#15808=CARTESIAN_POINT ( 'NONE',  ( -0.1343543525242022474, -0.09328364641522272904, -0.1179723892412200270 ) ) ;
#15811=CARTESIAN_POINT ( 'NONE',  ( 0.1113553986120547346, -0.5541338581601890079, 0.1113553986120547346 ) ) ;
#15814=CARTESIAN_POINT ( 'NONE',  ( -0.1666288720097009179, -0.08956157984806185912, 0.02185444682987447082 ) ) ;
#15823=CARTESIAN_POINT ( 'NONE',  ( -0.1574803149606299191, -0.02755905511811023584, 0.000000000000000000 ) ) ;
#15824=CARTESIAN_POINT ( 'NONE',  ( -0.1264236179284866091, -1.698326771599779628, -0.1264236179284866091 ) ) ;
#15825=CARTESIAN_POINT ( 'NONE',  ( 0.1787899950787401882, -0.9306102361667086820, -2.189545951927503898E-17 ) ) ;
#15826=CARTESIAN_POINT ( 'NONE',  ( -0.1113553986120547346, -1.213582677165354395, -0.1113553986120547346 ) ) ;
#15844=CARTESIAN_POINT ( 'NONE',  ( 0.06179214533981935986, 0.08095196624129888385, 0.2497573591203926524 ) ) ;
#15850=CARTESIAN_POINT ( 'NONE',  ( -0.2415622317366385718, -0.09842519685039370636, -0.02995051380158457108 ) ) ;
#15856=CARTESIAN_POINT ( 'NONE',  ( -1.094772975963752103E-17, -0.8420275590013542866, -0.1787899950787401882 ) ) ;
#15857=CARTESIAN_POINT ( 'NONE',  ( 0.1787899950787401604, -1.046259842465921297, 0.07405724077823318263 ) ) ;
#15859=CARTESIAN_POINT ( 'NONE',  ( -1.100456976456230270E-17, -0.3258312111578488546, -0.1797182628040039365 ) ) ;
#15868=CARTESIAN_POINT ( 'NONE',  ( -1.094772975963752103E-17, -0.4089566928596221063, -0.1787899950787401882 ) ) ;
#15870=CARTESIAN_POINT ( 'NONE',  ( -0.1787899950787401604, -1.223425196796630532, -0.07405724077823318263 ) ) ;
#15883=ADVANCED_FACE ( 'NONE', ( #20114 ), #27352, .T. ) ;
#15884=CARTESIAN_POINT ( 'NONE',  ( -0.1302006108103286042, -0.09843743769978773039, -0.1225641731413484731 ) ) ;
#15895=CARTESIAN_POINT ( 'NONE',  ( -0.1522882881087165574, -0.09851385314725177866, -0.2000479292304901680 ) ) ;
#15901=CARTESIAN_POINT ( 'NONE',  ( -0.07405724077823318263, -1.401698771378846464, -0.1787899950787401604 ) ) ;
#15904=CARTESIAN_POINT ( 'NONE',  ( 0.07405724077823318263, -0.3818897637257640532, 0.1787899950787401604 ) ) ;
#15910=CARTESIAN_POINT ( 'NONE',  ( 0.1264236179284866091, -0.2170275590013547307, -0.1264236179284866091 ) ) ;
#15912=CARTESIAN_POINT ( 'NONE',  ( -1.094772975963752103E-17, -1.747539370024976391, -0.1787899950787401882 ) ) ;
#15917=CARTESIAN_POINT ( 'NONE',  ( 0.06523048226347956391, -0.7632874015748020158, 0.1574803149606297803 ) ) ;
#15919=CARTESIAN_POINT ( 'NONE',  ( -0.07444174185955065859, -1.568449321394070006, 0.1797182628040039087 ) ) ;
#15928=CARTESIAN_POINT ( 'NONE',  ( -0.06523048226347956391, -0.8518700786326312002, -0.1574803149606300301 ) ) ;
#15929=CARTESIAN_POINT ( 'NONE',  ( -0.07405724077823318263, -0.01279527553678766298, -0.1787899950787401604 ) ) ;
#15943=CARTESIAN_POINT ( 'NONE',  ( 0.1797182628040039365, 0.01865697781852925299, -2.200913952912460540E-17 ) ) ;
#15944=CARTESIAN_POINT ( 'NONE',  ( 0.1264236179284866091, -1.368602362150960650, 0.1264236179284866091 ) ) ;
#15961=CARTESIAN_POINT ( 'NONE',  ( 0.1113553986120547346, -0.04232283453814220803, 0.1113553986120547346 ) ) ;
#15966=CARTESIAN_POINT ( 'NONE',  ( 0.1787899950787401604, -1.022761763504828059, 0.07405724077823318263 ) ) ;
#15968=CARTESIAN_POINT ( 'NONE',  ( 0.1264236179284866091, 0.09301181107738563936, 0.1264236179284866091 ) ) ;
#15975=CARTESIAN_POINT ( 'NONE',  ( 3.284318927891251994E-17, -0.7042322834108031282, 0.1787899950787401882 ) ) ;
#15980=CARTESIAN_POINT ( 'NONE',  ( 0.1797182628040039365, -1.044335148165722593, -2.200913952912460540E-17 ) ) ;
#15993=CARTESIAN_POINT ( 'NONE',  ( 0.07405724077823318263, -0.9576771653005667906, -0.1787899950787401604 ) ) ;
#15997=CARTESIAN_POINT ( 'NONE',  ( -0.06523048226347956391, -1.678641732175937706, -0.1574803149606300301 ) ) ;
#16001=EDGE_CURVE ( 'NONE', #30540, #3096, #44254, .T. ) ;
#16003=CARTESIAN_POINT ( 'NONE',  ( -0.1574803149606299191, -1.799212598425196763, 0.000000000000000000 ) ) ;
#16010=CARTESIAN_POINT ( 'NONE',  ( 0.1264236179284866091, -1.526082677111590513, 0.1264236179284866091 ) ) ;
#16012=AXIS2_PLACEMENT_3D ( 'NONE', #7801, #32526, #44212 ) ;
#16018=CARTESIAN_POINT ( 'NONE',  ( 0.07405724077823318263, -0.6339822359457745193, 0.1787899950787401604 ) ) ;
#16019=CARTESIAN_POINT ( 'NONE',  ( -0.1609361112149740314, -0.08956130496922656836, -0.06600197363463798650 ) ) ;
#16028=CARTESIAN_POINT ( 'NONE',  ( 0.1787899950787401882, -1.560531496009228247, -2.189545951927503898E-17 ) ) ;
#16029=CARTESIAN_POINT ( 'NONE',  ( -0.1787899950787401604, -1.572834645615527327, 0.07405724077823318263 ) ) ;
#16036=CARTESIAN_POINT ( 'NONE',  ( 0.1574803149606300301, -0.4384842519685039908, -0.06523048226347956391 ) ) ;
#16048=CARTESIAN_POINT ( 'NONE',  ( -0.09718287230280656108, -0.08956224776672244703, 0.1265413919071203541 ) ) ;
#16049=CARTESIAN_POINT ( 'NONE',  ( 0.07405724077823318263, -0.5393700786863945273, 0.1787899950787401604 ) ) ;
#16057=CARTESIAN_POINT ( 'NONE',  ( -0.1264236179284866091, -1.727854330654897685, 0.1264236179284866091 ) ) ;
#16058=CARTESIAN_POINT ( 'NONE',  ( -0.1787899950787401604, -0.9478346456155283262, 0.07405724077823318263 ) ) ;
#16059=CARTESIAN_POINT ( 'NONE',  ( 2.892866454678787531E-17, -1.198818897637795367, 0.1574803149606299191 ) ) ;
#16065=ORIENTED_EDGE ( 'NONE', *, *, #10024, .T. ) ;
#16068=CARTESIAN_POINT ( 'NONE',  ( -0.1574803149606299191, -1.395669291231055098, 0.000000000000000000 ) ) ;
#16075=DIRECTION ( 'NONE',  ( 0.4999999999999998890, 0.000000000000000000, -0.8660254037844388186 ) ) ;
#16081=CARTESIAN_POINT ( 'NONE',  ( -0.2037826476351566884, -0.09842519685039370636, 0.1181336077123911338 ) ) ;
#16089=CARTESIAN_POINT ( 'NONE',  ( 3.284318927891251994E-17, -0.9404527558517480346, 0.1787899950787401882 ) ) ;
#16090=EDGE_CURVE ( 'NONE', #799, #5551, #26561, .T. ) ;
#16091=CARTESIAN_POINT ( 'NONE',  ( 0.1264236179284866091, -1.117618110182456714, -0.1264236179284866091 ) ) ;
#16094=CARTESIAN_POINT ( 'NONE',  ( -0.1270800023317771588, -0.3110674316302897702, 0.1270800023317771588 ) ) ;
#16097=CARTESIAN_POINT ( 'NONE',  ( 0.1787899950787401604, -0.1850393700249766959, 0.07405724077823318263 ) ) ;
#16106=CARTESIAN_POINT ( 'NONE',  ( -0.1787899950787401882, -0.3991141731745826982, 0.000000000000000000 ) ) ;
#16109=CARTESIAN_POINT ( 'NONE',  ( -0.07405724077823318263, -1.188976377898991688, -0.1787899950787401604 ) ) ;
#16119=CARTESIAN_POINT ( 'NONE',  ( -0.08452081858070546738, -0.09842406081630053483, -0.1575734998833499545 ) ) ;
#16123=CARTESIAN_POINT ( 'NONE',  ( -0.05467468201772657937, -0.07678538764759451629, 0.2538665577330194156 ) ) ;
#16137=CARTESIAN_POINT ( 'NONE',  ( 0.1264236179284866091, -0.4483267715997795166, -0.1264236179284866091 ) ) ;
#16147=CARTESIAN_POINT ( 'NONE',  ( -0.1264236179284866091, -1.732775590497417362, 0.1264236179284866091 ) ) ;
#16151=CARTESIAN_POINT ( 'NONE',  ( 0.1113553986120547346, -0.7509842519685040463, -0.1113553986120547346 ) ) ;
#16153=CARTESIAN_POINT ( 'NONE',  ( 0.1797182628040039087, -1.553685541866510755, -0.07444174185955065859 ) ) ;
#16155=CARTESIAN_POINT ( 'NONE',  ( 0.2471922904502825702, 0.07746962187842010295, -0.07828042841528085050 ) ) ;
#16163=CARTESIAN_POINT ( 'NONE',  ( -0.1787899950787401882, -0.005413385773008132923, 0.000000000000000000 ) ) ;
#16174=CARTESIAN_POINT ( 'NONE',  ( -0.1787899950787401882, -1.383366141678519678, 0.000000000000000000 ) ) ;
#16190=CARTESIAN_POINT ( 'NONE',  ( 0.1574803149606300301, -0.0004921258767249256719, 0.06523048226347956391 ) ) ;
#16194=CARTESIAN_POINT ( 'NONE',  ( -0.1264236179284866091, -1.044907432796167157, -0.1264236179284866091 ) ) ;
#16197=CARTESIAN_POINT ( 'NONE',  ( -1.094772975963752103E-17, 0.02903543312462964626, -0.1787899950787401882 ) ) ;
#16208=CARTESIAN_POINT ( 'NONE',  ( 0.1264236179284866091, -0.6107283464029291675, -0.1264236179284866091 ) ) ;
#16213=CARTESIAN_POINT ( 'NONE',  ( -0.1797182628040039365, -1.103390266275958709, 0.000000000000000000 ) ) ;
#16217=FACE_OUTER_BOUND ( 'NONE', #17502, .T. ) ;
#16229=CARTESIAN_POINT ( 'NONE',  ( 0.06523048226347956391, -1.683562992018456272, -0.1574803149606300301 ) ) ;
#16235=CARTESIAN_POINT ( 'NONE',  ( 0.07405724077823318263, 0.1299212598962831977, 0.1787899950787401604 ) ) ;
#16241=CARTESIAN_POINT ( 'NONE',  ( -0.05557684098944758871, 0.07733267719194715506, 0.2533457667601751728 ) ) ;
#16243=CARTESIAN_POINT ( 'NONE',  ( 3.284318927891251994E-17, -1.531003936954110189, 0.1787899950787401882 ) ) ;
#16251=CARTESIAN_POINT ( 'NONE',  ( -1.094772975963752103E-17, -0.5773877477567976868, -0.1787899950787401882 ) ) ;
#16252=CARTESIAN_POINT ( 'NONE',  ( 0.1974933268882626269, -0.08956039363871731718, -0.04058527935846337892 ) ) ;
#16255=CARTESIAN_POINT ( 'NONE',  ( -0.07405724077823318263, -1.820005857993018505, 0.1787899950787401604 ) ) ;
#16257=ORIENTED_EDGE ( 'NONE', *, *, #30083, .F. ) ;
#16261=CARTESIAN_POINT ( 'NONE',  ( 0.07405724077823318263, -1.513779527505292322, -0.1787899950787401604 ) ) ;
#16267=CARTESIAN_POINT ( 'NONE',  ( -0.1797182628040039087, -0.7515201875358006323, -0.07444174185955065859 ) ) ;
#16271=CARTESIAN_POINT ( 'NONE',  ( -0.06523048226347956391, -0.4286417322834646937, -0.1574803149606300301 ) ) ;
#16283=CARTESIAN_POINT ( 'NONE',  ( -0.1264236179284866091, -0.5073818897100158543, 0.1264236179284866091 ) ) ;
#16290=CARTESIAN_POINT ( 'NONE',  ( -0.07405724077823318263, -1.700787401521039355, -0.1787899950787401604 ) ) ;
#16291=CARTESIAN_POINT ( 'NONE',  ( -0.1787899950787401604, -0.9133858267178897039, -0.07405724077823318263 ) ) ;
#16292=CARTESIAN_POINT ( 'NONE',  ( 0.1113553986120547346, -1.420275590551181244, -0.1113553986120547346 ) ) ;
#16301=CARTESIAN_POINT ( 'NONE',  ( -0.1574803149606299191, -1.356299212490897466, 0.000000000000000000 ) ) ;
#16312=CARTESIAN_POINT ( 'NONE',  ( -0.1806410355270206824, 0.08353766247254197641, 0.1811399203779236189 ) ) ;
#16316=CARTESIAN_POINT ( 'NONE',  ( 0.1815364857181279989, -0.09842519685039370636, -0.08952795644902836192 ) ) ;
#16320=EDGE_CURVE ( 'NONE', #36603, #33652, #5559, .T. ) ;
#16325=CARTESIAN_POINT ( 'NONE',  ( 3.284318927891251994E-17, -1.250492125930488196, 0.1787899950787401882 ) ) ;
#16326=PRODUCT_DEFINITION ( 'UNKNOWN', '', #12514, #13986 ) ;
#16328=CARTESIAN_POINT ( 'NONE',  ( -0.1270800023317771588, -0.2815398725751716569, -0.1270800023317771588 ) ) ;
#16329=CARTESIAN_POINT ( 'NONE',  ( 0.1574803149606300301, -1.806594488081449512, -0.06523048226347956391 ) ) ;
#16332=CARTESIAN_POINT ( 'NONE',  ( 2.892866454678787531E-17, -0.01771653543307086590, 0.1574803149606299191 ) ) ;
#16339=AXIS2_PLACEMENT_3D ( 'NONE', #4463, #30413, #22949 ) ;
#16341=CARTESIAN_POINT ( 'NONE',  ( 3.284318927891251994E-17, -0.4680118109698582773, 0.1787899950787401882 ) ) ;
#16343=CARTESIAN_POINT ( 'NONE',  ( 0.07405724077823318263, -1.444881889710016631, 0.1787899950787401604 ) ) ;
#16351=CARTESIAN_POINT ( 'NONE',  ( -0.1545411696117860445, -0.09842519685039370636, -0.08990488994085453489 ) ) ;
#16356=CARTESIAN_POINT ( 'NONE',  ( 0.1898890638025254318, -0.07836638817768155907, -0.1758005714383412132 ) ) ;
#16363=CARTESIAN_POINT ( 'NONE',  ( -0.2092529681372728712, -0.09851385015114920429, 0.1092847636717405591 ) ) ;
#16368=CARTESIAN_POINT ( 'NONE',  ( 0.1787899950787401882, -1.650222393426088896, -2.189545951927503898E-17 ) ) ;
#16371=CARTESIAN_POINT ( 'NONE',  ( -0.1787899950787401604, -0.5147637794737950356, -0.07405724077823318263 ) ) ;
#16376=CARTESIAN_POINT ( 'NONE',  ( 0.07405724077823318263, -0.2145669290800947537, -0.1787899950787401604 ) ) ;
#16380=CARTESIAN_POINT ( 'NONE',  ( -0.1264236179284866091, 0.1066673703534383871, 0.1264236179284866091 ) ) ;
#16381=CARTESIAN_POINT ( 'NONE',  ( -0.07405724077823318263, -1.779527559001355952, -0.1787899950787401604 ) ) ;
#16387=CARTESIAN_POINT ( 'NONE',  ( -0.1574803149606300301, -0.8174212598425197873, -0.06523048226347956391 ) ) ;
#16388=CARTESIAN_POINT ( 'NONE',  ( 2.892866454678787531E-17, 0.1003937007874015908, 0.1574803149606299191 ) ) ;
#16389=CARTESIAN_POINT ( 'NONE',  ( -0.1270800023317771588, -1.531539872575170991, 0.1270800023317771588 ) ) ;
#16390=CARTESIAN_POINT ( 'NONE',  ( 2.892866454678787531E-17, -0.04724409438066189126, 0.1574803149606299191 ) ) ;
#16391=CARTESIAN_POINT ( 'NONE',  ( 0.06523048226347956391, -0.4778543306011345249, 0.1574803149606297803 ) ) ;
#16392=CARTESIAN_POINT ( 'NONE',  ( 0.1264236179284866091, -0.3794291338045042705, 0.1264236179284866091 ) ) ;
#16393=DIRECTION ( 'NONE',  ( 0.000000000000000000, 1.000000000000000000, 0.000000000000000000 ) ) ;
#16397=DIRECTION ( 'NONE',  ( 0.000000000000000000, 0.000000000000000000, 1.000000000000000000 ) ) ;
#16400=CARTESIAN_POINT ( 'NONE',  ( 0.07405724077823318263, 0.06102362210100767403, -0.1787899950787401604 ) ) ;
#16402=FACE_OUTER_BOUND ( 'NONE', #41874, .T. ) ;
#16415=DIRECTION ( 'NONE',  ( 0.000000000000000000, 1.000000000000000000, 0.000000000000000000 ) ) ;
#16425=CARTESIAN_POINT ( 'NONE',  ( -0.1113553986120547346, -0.1801181101286933040, -0.1113553986120547346 ) ) ;
#16431=CARTESIAN_POINT ( 'NONE',  ( 0.1787899950787401604, -1.214690897363096989, -0.07405724077823318263 ) ) ;
#16433=CARTESIAN_POINT ( 'NONE',  ( -1.094772975963752103E-17, -0.01033464561552785432, -0.1787899950787401882 ) ) ;
#16434=EDGE_LOOP ( 'NONE', ( #14755, #1539, #32756, #17283 ) ) ;
#16439=AXIS2_PLACEMENT_3D ( 'NONE', #24455, #37767, #12139 ) ;
#16441=CARTESIAN_POINT ( 'NONE',  ( -0.1787899950787401604, -0.5541338582139530011, 0.07405724077823318263 ) ) ;
#16444=CARTESIAN_POINT ( 'NONE',  ( -0.1797182628040039365, -1.221500502496431162, 0.000000000000000000 ) ) ;
#16458=CARTESIAN_POINT ( 'NONE',  ( 0.1574803149606300301, -1.767224409341291658, -0.06523048226347956391 ) ) ;
#16462=CARTESIAN_POINT ( 'NONE',  ( 0.1787899950787401604, 0.1397637795813224670, -0.07405724077823318263 ) ) ;
#16472=CARTESIAN_POINT ( 'NONE',  ( -0.07405724077823318263, -1.587598425143086800, -0.1787899950787401604 ) ) ;
#16482=CARTESIAN_POINT ( 'NONE',  ( -0.1264236179284866091, -0.7299468028749075410, -0.1264236179284866091 ) ) ;
#16483=CARTESIAN_POINT ( 'NONE',  ( 0.2021875001600378363, -0.08956021568874587835, -0.01555348493781427179 ) ) ;
#16488=CARTESIAN_POINT ( 'NONE',  ( -0.1787899950787401604, -1.824927117835538182, 0.07405724077823318263 ) ) ;
#16490=CARTESIAN_POINT ( 'NONE',  ( -0.1264236179284866091, -1.467027559001354398, -0.1264236179284866091 ) ) ;
#16497=CARTESIAN_POINT ( 'NONE',  ( -0.07444174185955065859, -0.7023075891106040913, 0.1797182628040039087 ) ) ;
#16500=CARTESIAN_POINT ( 'NONE',  ( -0.1113553986120547346, -0.3868110236220472786, -0.1113553986120547346 ) ) ;
#16504=DIRECTION ( 'NONE',  ( 0.000000000000000000, 1.000000000000000000, 0.000000000000000000 ) ) ;
#16514=CARTESIAN_POINT ( 'NONE',  ( -0.1642785720453234233, -0.08956005481713959215, -0.05376805096173911669 ) ) ;
#16515=CARTESIAN_POINT ( 'NONE',  ( -0.1787899950787401882, -0.5123031495525355306, 0.000000000000000000 ) ) ;
#16522=CARTESIAN_POINT ( 'NONE',  ( -1.094772975963752103E-17, -1.781988188922614347, -0.1787899950787401882 ) ) ;
#16523=CARTESIAN_POINT ( 'NONE',  ( 0.07405724077823318263, -0.9773622046706458288, 0.1787899950787401604 ) ) ;
#16524=CARTESIAN_POINT ( 'NONE',  ( -0.1574803149606300301, -1.289862204724410155, -0.06523048226347956391 ) ) ;
#16533=CARTESIAN_POINT ( 'NONE',  ( 0.1574803149606300301, 0.004429133965794757564, -0.06523048226347956391 ) ) ;
#16540=CARTESIAN_POINT ( 'NONE',  ( -0.2227678560577956990, 0.05525422739379964865, -0.1568179892043777002 ) ) ;
#16543=CARTESIAN_POINT ( 'NONE',  ( 0.03810507699822260341, -0.06563552548610589177, -0.2634293601846930399 ) ) ;
#16547=CARTESIAN_POINT ( 'NONE',  ( 0.1576911482518127960, -0.09842519685039370636, -0.1232761894637649652 ) ) ;
#16550=CARTESIAN_POINT ( 'NONE',  ( -0.1264236179284866091, -1.063484251914740275, 0.1264236179284866091 ) ) ;
#16552=CARTESIAN_POINT ( 'NONE',  ( -0.07405724077823318263, -1.267716535379307619, -0.1787899950787401604 ) ) ;
#16556=CARTESIAN_POINT ( 'NONE',  ( 0.1574803149606299191, 0.03149606299212598381, -1.928577636452523993E-17 ) ) ;
#16557=CIRCLE ( 'NONE', #8120, 0.2471922904502826812 ) ;
#16565=CARTESIAN_POINT ( 'NONE',  ( -0.1264236179284866091, -0.4434055117572598959, -0.1264236179284866091 ) ) ;
#16567=CARTESIAN_POINT ( 'NONE',  ( 3.284318927891251994E-17, -1.329232283410803239, 0.1787899950787401882 ) ) ;
#16577=CARTESIAN_POINT ( 'NONE',  ( 0.06523048226347956391, -1.225885826664126155, 0.1574803149606297803 ) ) ;
#16581=CARTESIAN_POINT ( 'NONE',  ( 0.1441367711531681417, -0.09842284166182276028, -0.1062059330993350148 ) ) ;
#16592=CARTESIAN_POINT ( 'NONE',  ( 0.1098255079058281514, -0.09851384733571673380, 0.1889249215128767645 ) ) ;
#16599=CARTESIAN_POINT ( 'NONE',  ( 0.1787899950787401604, -0.6131889763241887836, 0.07405724077823318263 ) ) ;
#16604=CARTESIAN_POINT ( 'NONE',  ( -0.1787899950787401882, -0.8272637794737952577, 0.000000000000000000 ) ) ;
#16608=CARTESIAN_POINT ( 'NONE',  ( -0.07405724077823318263, 0.03038784279438331778, 0.1787899950787401604 ) ) ;
#16609=CARTESIAN_POINT ( 'NONE',  ( 0.07405724077823318263, -1.799212598371432659, 0.1787899950787401604 ) ) ;
#16615=CARTESIAN_POINT ( 'NONE',  ( -9.642888182262618425E-18, -0.8641732283464567121, -0.1574803149606299191 ) ) ;
#16617=CARTESIAN_POINT ( 'NONE',  ( -0.07444174185955065859, -1.607819400134226528, 0.1797182628040039087 ) ) ;
#16625=CARTESIAN_POINT ( 'NONE',  ( 0.07405724077823318263, 0.1003937008411650705, -0.1787899950787401604 ) ) ;
#16636=CARTESIAN_POINT ( 'NONE',  ( 0.07405724077823318263, -1.316929133804503937, -0.1787899950787401604 ) ) ;
#16643=CARTESIAN_POINT ( 'NONE',  ( 0.2471922904502826812, 0.03219022224904102836, -0.1427165354330708902 ) ) ;
#16655=CARTESIAN_POINT ( 'NONE',  ( -0.1574803149606299191, -0.2145669290263310935, 0.000000000000000000 ) ) ;
#16659=CARTESIAN_POINT ( 'NONE',  ( -0.1787899950787401604, -1.195005857993017839, 0.07405724077823318263 ) ) ;
#16661=CARTESIAN_POINT ( 'NONE',  ( -1.094772975963752103E-17, -0.08907480309584270284, -0.1787899950787401882 ) ) ;
#16662=EDGE_LOOP ( 'NONE', ( #13962, #3513, #20540, #37451 ) ) ;
#16667=CARTESIAN_POINT ( 'NONE',  ( -0.1787899950787401604, -0.5984251967966303098, -0.07405724077823318263 ) ) ;
#16673=CARTESIAN_POINT ( 'NONE',  ( 0.07444174185955065859, -1.091087116669658963, 0.1797182628040039087 ) ) ;
#16679=EDGE_CURVE ( 'NONE', #5551, #30540, #24257, .T. ) ;
#16693=CARTESIAN_POINT ( 'NONE',  ( 0.06523048226347956391, -1.698326771546016190, 0.1574803149606297803 ) ) ;
#16698=CARTESIAN_POINT ( 'NONE',  ( -0.1264236179284866091, 0.07332677170730689253, -0.1264236179284866091 ) ) ;
#16702=CARTESIAN_POINT ( 'NONE',  ( -0.1787899950787401882, -1.698326771599779628, 0.000000000000000000 ) ) ;
#16709=CARTESIAN_POINT ( 'NONE',  ( 0.07405724077823318263, -0.6585885351583735670, -0.1787899950787401604 ) ) ;
#16711=CARTESIAN_POINT ( 'NONE',  ( 0.1920494157074515706, -0.08956033323250511824, 0.08002985433875355048 ) ) ;
#16721=CARTESIAN_POINT ( 'NONE',  ( -1.094772975963752103E-17, -1.550688976324188895, -0.1787899950787401882 ) ) ;
#16725=CARTESIAN_POINT ( 'NONE',  ( 3.301370929368692659E-17, -0.6998469591893444752, 0.1797182628040039365 ) ) ;
#16729=CARTESIAN_POINT ( 'NONE',  ( 0.1113553986120547346, -0.4458661417322834497, 0.1113553986120547346 ) ) ;
#16730=CARTESIAN_POINT ( 'NONE',  ( -0.04902506021456321667, -0.09842519685039372024, 0.1521997253933253247 ) ) ;
#16743=CARTESIAN_POINT ( 'NONE',  ( 0.07405724077823318263, -0.6181102361667089040, 0.1787899950787401604 ) ) ;
#16750=CARTESIAN_POINT ( 'NONE',  ( 0.1787899950787401882, -1.791830708607653699, -2.189545951927503898E-17 ) ) ;
#16751=CARTESIAN_POINT ( 'NONE',  ( -0.1264236179284866091, -1.033956692859621995, -0.1264236179284866091 ) ) ;
#16752=CARTESIAN_POINT ( 'NONE',  ( 0.1574803149606300301, -1.422736220472442081, -0.06523048226347956391 ) ) ;
#16768=CARTESIAN_POINT ( 'NONE',  ( -0.1264236179284866091, -0.2968759367331759713, -0.1264236179284866091 ) ) ;
#16770=CARTESIAN_POINT ( 'NONE',  ( 0.1917573881879755804, -0.09842519685039370636, 0.09087608798953976386 ) ) ;
#16778=B_SPLINE_CURVE_WITH_KNOTS ( 'NONE', 3,
 ( #22494, #37114, #30437, #40918, #11488, #36888, #45228, #40454, #37836, #18895, #33794, #44757, #15808, #7639, #44522, #4994, #666, #15321, #1152 ),
 .UNSPECIFIED., .F., .F.,
 ( 4, 2, 1, 1, 2, 2, 2, 1, 2, 2, 4 ),
 ( 0.000000000000000000, 0.1250000000000000278, 0.1875000000000001110, 0.2187500000000001388, 0.2343750000000006661, 0.2500000000000011657, 0.3750000000000031086, 0.4375000000000041078, 0.4687500000000042744, 0.5000000000000044409, 1.000000000000000000 ),
 .UNSPECIFIED. ) ;
#16779=CARTESIAN_POINT ( 'NONE',  ( -0.1787899950787401604, -1.257874015694269376, 0.07405724077823318263 ) ) ;
#16783=CARTESIAN_POINT ( 'NONE',  ( -0.1797182628040039087, -0.4365595576145414047, -0.07444174185955065859 ) ) ;
#16786=CARTESIAN_POINT ( 'NONE',  ( 0.1574803149606300301, -0.005413385826771673418, -0.06523048226347956391 ) ) ;
#16791=CARTESIAN_POINT ( 'NONE',  ( 3.284318927891251994E-17, -0.6254921259304881964, 0.1787899950787401882 ) ) ;
#16792=CARTESIAN_POINT ( 'NONE',  ( -0.1787899950787401604, -1.459645669237573884, -0.07405724077823318263 ) ) ;
#16802=CARTESIAN_POINT ( 'NONE',  ( 0.1349619066862741967, -0.09842519684088384124, -0.1172652914709395727 ) ) ;
#16806=CYLINDRICAL_SURFACE ( 'NONE', #20009, 0.1574803149606299191 ) ;
#16812=CARTESIAN_POINT ( 'NONE',  ( 0.1917907757321275775, -0.09851384566401279186, 0.09088981981130157817 ) ) ;
#16816=CARTESIAN_POINT ( 'NONE',  ( -0.1264236179284866091, -1.625616094213490292, 0.1264236179284866091 ) ) ;
#16819=CARTESIAN_POINT ( 'NONE',  ( -0.1787899950787401882, -0.5910433070328504623, 0.000000000000000000 ) ) ;
#16823=CARTESIAN_POINT ( 'NONE',  ( -0.1264236179284866091, -0.7042322834108031282, 0.1264236179284866091 ) ) ;
#16828=CARTESIAN_POINT ( 'NONE',  ( 0.07405724077823318263, 0.05007288216446208196, -0.1787899950787401604 ) ) ;
#16829=CARTESIAN_POINT ( 'NONE',  ( 0.1787899950787401882, 0.05364173233722811102, -2.189545951927503898E-17 ) ) ;
#16835=CARTESIAN_POINT ( 'NONE',  ( 0.1574803149606299191, -0.9527559055118109965, -1.928577636452523993E-17 ) ) ;
#16837=CARTESIAN_POINT ( 'NONE',  ( -0.1797182628040039365, -1.536461132417690667, 0.000000000000000000 ) ) ;
#16838=CARTESIAN_POINT ( 'NONE',  ( -9.642888182262618425E-18, -0.06692913375074074911, -0.1574803149606299191 ) ) ;
#16847=CARTESIAN_POINT ( 'NONE',  ( -0.07405724077823318263, 0.1053149606836847191, -0.1787899950787401604 ) ) ;
#16849=CARTESIAN_POINT ( 'NONE',  ( 0.1264236179284866091, -0.05462598419820496182, -0.1264236179284866091 ) ) ;
#16851=CARTESIAN_POINT ( 'NONE',  ( -0.1787899950787401604, -0.9084645668753701386, -0.07405724077823318263 ) ) ;
#16857=CARTESIAN_POINT ( 'NONE',  ( -0.06523048226347956391, -1.073326771546015301, 0.1574803149606297803 ) ) ;
#16858=CARTESIAN_POINT ( 'NONE',  ( -0.07405724077823318263, -1.336614173174582865, 0.1787899950787401604 ) ) ;
#16866=UNCERTAINTY_MEASURE_WITH_UNIT (LENGTH_MEASURE( 1.000000000000000082E-05 ), #6683, 'distance_accuracy_value', 'NONE') ;
#16878=CARTESIAN_POINT ( 'NONE',  ( -0.2471922904502826812, 0.07845432542752767135, -0.07637674237069251582 ) ) ;
#16881=CARTESIAN_POINT ( 'NONE',  ( 0.1787899950787401604, -1.180242078465460143, 0.07405724077823318263 ) ) ;
#16883=CARTESIAN_POINT ( 'NONE',  ( -0.1264236179284866091, -0.1235236219934805202, -0.1264236179284866091 ) ) ;
#16891=CARTESIAN_POINT ( 'NONE',  ( 0.07405724077823318263, -0.5688976377415115859, -0.1787899950787401604 ) ) ;
#16899=CARTESIAN_POINT ( 'NONE',  ( 0.1270800023317771588, -1.196894203283832780, -0.1270800023317771588 ) ) ;
#16923=CARTESIAN_POINT ( 'NONE',  ( 0.1787899950787401882, 0.1373031496600628232, -2.189545951927503898E-17 ) ) ;
#16930=CARTESIAN_POINT ( 'NONE',  ( -0.1113553986120547346, -0.4064960628845984414, 0.1113553986120547346 ) ) ;
#16931=CARTESIAN_POINT ( 'NONE',  ( -0.1264236179284866091, -1.693405511757259951, 0.1264236179284866091 ) ) ;
#16935=EDGE_CURVE ( 'NONE', #36616, #3517, #25456, .T. ) ;
#16938=CARTESIAN_POINT ( 'NONE',  ( 0.1561172342761355525, 0.1239648558221263380, -0.04236179190153568225 ) ) ;
#16940=CARTESIAN_POINT ( 'NONE',  ( 0.1264236179284866091, -0.6708916847646714254, 0.1264236179284866091 ) ) ;
#16942=CARTESIAN_POINT ( 'NONE',  ( 0.1614456555785303005, -0.08956047347222421962, -0.1130746612548063079 ) ) ;
#16959=CARTESIAN_POINT ( 'NONE',  ( 2.892866454678787531E-17, -0.4901574803149605919, 0.1574803149606299191 ) ) ;
#16965=CARTESIAN_POINT ( 'NONE',  ( 0.1574803149606299191, 0.08070866152484981737, -1.928577636452523993E-17 ) ) ;
#16969=CARTESIAN_POINT ( 'NONE',  ( 0.06523048226347956391, -0.5959645668216069225, 0.1574803149606297803 ) ) ;
#16974=CARTESIAN_POINT ( 'NONE',  ( 0.07405724077823318263, -0.4999999999462365619, 0.1787899950787401604 ) ) ;
#16982=CARTESIAN_POINT ( 'NONE',  ( -0.07444174185955065859, 0.1244640644327026091, 0.1797182628040039087 ) ) ;
#16983=CARTESIAN_POINT ( 'NONE',  ( -0.1787899950787401604, -1.065944881836000224, 0.07405724077823318263 ) ) ;
#16984=CARTESIAN_POINT ( 'NONE',  ( 0.1574803149606300301, -1.343996062992125706, -0.06523048226347956391 ) ) ;
#17004=CARTESIAN_POINT ( 'NONE',  ( 0.1264236179284866091, -0.2279782989379003921, -0.1264236179284866091 ) ) ;
#17005=CARTESIAN_POINT ( 'NONE',  ( 0.07326958550568327122, -0.09842519685039370636, 0.2080556247247394019 ) ) ;
#17008=EDGE_CURVE ( 'NONE', #40254, #10382, #3870, .T. ) ;
#17016=CARTESIAN_POINT ( 'NONE',  ( -1.094772975963752103E-17, -1.152066929080094448, -0.1787899950787401882 ) ) ;
#17018=CARTESIAN_POINT ( 'NONE',  ( -0.07444174185955065859, -0.5595910536775339228, -0.1797182628040039087 ) ) ;
#17022=CARTESIAN_POINT ( 'NONE',  ( -0.1574803149606300301, 0.04872047244094490637, -0.06523048226347956391 ) ) ;
#17032=CARTESIAN_POINT ( 'NONE',  ( 3.284318927891251994E-17, -0.6648622046706456068, 0.1787899950787401882 ) ) ;
#17033=CARTESIAN_POINT ( 'NONE',  ( 0.1787899950787401604, -1.361220472387181690, 0.07405724077823318263 ) ) ;
#17051=CARTESIAN_POINT ( 'NONE',  ( -0.2379425218648307250, -0.09851385171600395008, 0.03197312892090157371 ) ) ;
#17057=CARTESIAN_POINT ( 'NONE',  ( 0.1264236179284866091, -0.5270669290800944484, -0.1264236179284866091 ) ) ;
#17060=CARTESIAN_POINT ( 'NONE',  ( -0.1787899950787401882, -0.7878937007336378473, 0.000000000000000000 ) ) ;
#17066=CARTESIAN_POINT ( 'NONE',  ( -0.1787899950787401882, 0.06237603177076121719, 0.000000000000000000 ) ) ;
#17067=CARTESIAN_POINT ( 'NONE',  ( -0.1264236179284866091, 0.03887795280966901967, 0.1264236179284866091 ) ) ;
#17069=CARTESIAN_POINT ( 'NONE',  ( 0.04918729031099923488, -0.09842519685039373412, 0.1567634384477433751 ) ) ;
#17072=CARTESIAN_POINT ( 'NONE',  ( -0.1574803149606299191, -0.8937007874015748810, 0.000000000000000000 ) ) ;
#17074=CARTESIAN_POINT ( 'NONE',  ( 0.1270800023317771588, -1.797287904071236397, 0.1270800023317771588 ) ) ;
#17081=CARTESIAN_POINT ( 'NONE',  ( -0.1351206911654056209, -0.09842519685039369248, -0.2074211034487065675 ) ) ;
#17085=CARTESIAN_POINT ( 'NONE',  ( 0.06523048226347956391, -0.8961614172153083979, -0.1574803149606300301 ) ) ;
#17086=CARTESIAN_POINT ( 'NONE',  ( -0.1264236179284866091, -0.1678149605761578844, -0.1264236179284866091 ) ) ;
#17088=CARTESIAN_POINT ( 'NONE',  ( -0.1787899950787401882, -0.8666338582139527791, 0.000000000000000000 ) ) ;
#17096=CARTESIAN_POINT ( 'NONE',  ( -0.1113553986120547346, -1.075787401467275695, 0.1113553986120547346 ) ) ;
#17101=CARTESIAN_POINT ( 'NONE',  ( -0.2471922904502826812, -0.09842519685039370636, 0.1427165354330708902 ) ) ;
#17107=CARTESIAN_POINT ( 'NONE',  ( -0.1787899950787401882, 0.1126968504474643862, 0.000000000000000000 ) ) ;
#17114=CARTESIAN_POINT ( 'NONE',  ( -0.2471922904502826812, 0.07885719401822635644, -0.07558487950069482653 ) ) ;
#17116=CARTESIAN_POINT ( 'NONE',  ( -1.094772975963752103E-17, -1.089198771378844466, -0.1787899950787401882 ) ) ;
#17119=CARTESIAN_POINT ( 'NONE',  ( 0.07405724077823318263, -0.1850393700249766959, 0.1787899950787401604 ) ) ;
#17125=CARTESIAN_POINT ( 'NONE',  ( -0.07444174185955065859, -0.2298666442287148337, 0.1797182628040039087 ) ) ;
#17126=CARTESIAN_POINT ( 'NONE',  ( 0.07405724077823318263, -0.8051181101824581576, -0.1787899950787401604 ) ) ;
#17130=CARTESIAN_POINT ( 'NONE',  ( -0.1270800023317771588, -1.147681604858635795, -0.1270800023317771588 ) ) ;
#17138=CARTESIAN_POINT ( 'NONE',  ( -0.1574803149606299191, -0.7263779526483780113, 0.000000000000000000 ) ) ;
#17140=CARTESIAN_POINT ( 'NONE',  ( -0.07405724077823318263, 0.04625984257344856188, 0.1787899950787401604 ) ) ;
#17157=CARTESIAN_POINT ( 'NONE',  ( 0.07405724077823318263, -0.01279527553678768380, -0.1787899950787401604 ) ) ;
#17167=CARTESIAN_POINT ( 'NONE',  ( 0.1787899950787401604, -1.759842519631276581, 0.07405724077823318263 ) ) ;
#17176=CARTESIAN_POINT ( 'NONE',  ( 0.1264236179284866091, -0.7004192438197893722, -0.1264236179284866091 ) ) ;
#17184=CARTESIAN_POINT ( 'NONE',  ( 0.06523048226347956391, -0.0004921259842519827002, -0.1574803149606300301 ) ) ;
#17186=VECTOR ( 'NONE', #9688, 39.37007874015748143 ) ;
#17192=CARTESIAN_POINT ( 'NONE',  ( -1.100456976456230270E-17, -0.6801619198192657700, -0.1797182628040039365 ) ) ;
#17193=CARTESIAN_POINT ( 'NONE',  ( -0.1574803149606297803, -0.6550196850393706915, 0.06523048226347956391 ) ) ;
#17194=CARTESIAN_POINT ( 'NONE',  ( 0.000000000000000000, -0.09842519685039370636, 0.000000000000000000 ) ) ;
#17207=CARTESIAN_POINT ( 'NONE',  ( -0.1611263444889494134, -0.08956074569868537061, -0.06449846707264046686 ) ) ;
#17208=CARTESIAN_POINT ( 'NONE',  ( -0.1787899950787401604, -0.6673228345919050009, 0.07405724077823318263 ) ) ;
#17209=AXIS2_PLACEMENT_3D ( 'NONE', #313, #33654, #14962 ) ;
#17210=ORIENTED_EDGE ( 'NONE', *, *, #46039, .T. ) ;
#17219=CARTESIAN_POINT ( 'NONE',  ( -0.07405724077823318263, -1.804133858213953889, 0.1787899950787401604 ) ) ;
#17220=CARTESIAN_POINT ( 'NONE',  ( -0.1787899950787401604, -1.105314960576158301, 0.07405724077823318263 ) ) ;
#17221=CARTESIAN_POINT ( 'NONE',  ( 0.1113553986120547346, -1.302165354330708791, -0.1113553986120547346 ) ) ;
#17232=CARTESIAN_POINT ( 'NONE',  ( -0.2471922904502826257, 0.07319706521783654607, 0.08615678709745397401 ) ) ;
#17234=CARTESIAN_POINT ( 'NONE',  ( -0.2272550450522833887, 0.05212746764704522667, 0.1542273094305053049 ) ) ;
#17237=CARTESIAN_POINT ( 'NONE',  ( 0.07405724077823318263, -0.3042578264969555413, -0.1787899950787401604 ) ) ;
#17238=CARTESIAN_POINT ( 'NONE',  ( 0.03196316912850031416, -0.09842519685039370636, -0.1894554451039858478 ) ) ;
#17248=CARTESIAN_POINT ( 'NONE',  ( -0.1787899950787401604, -1.188976377898991688, -0.07405724077823318263 ) ) ;
#17249=CARTESIAN_POINT ( 'NONE',  ( -1.094772975963752103E-17, -1.270177165300566902, -0.1787899950787401882 ) ) ;
#17250=CARTESIAN_POINT ( 'NONE',  ( -0.1797182628040039087, -0.4710083765121794164, 0.07444174185955065859 ) ) ;
#17253=CARTESIAN_POINT ( 'NONE',  ( 0.1113553986120547346, 0.03641732283464567399, -0.1113553986120547346 ) ) ;
#17259=CARTESIAN_POINT ( 'NONE',  ( 1.928577636452524610E-17, -0.09842519685039370636, -0.1574803149606299191 ) ) ;
#17267=CARTESIAN_POINT ( 'NONE',  ( 0.07405724077823318263, -0.5688976377415115859, -0.1787899950787401604 ) ) ;
#17268=CARTESIAN_POINT ( 'NONE',  ( 0.1787899950787401604, -1.316929133804503937, -0.07405724077823318263 ) ) ;
#17278=CARTESIAN_POINT ( 'NONE',  ( 0.1635870200194612933, -0.09842519684036495076, -0.07221633666346874425 ) ) ;
#17283=ORIENTED_EDGE ( 'NONE', *, *, #7959, .F. ) ;
#17288=CARTESIAN_POINT ( 'NONE',  ( -0.002277221062301980261, -0.09851385079347381446, 0.2245454195424968769 ) ) ;
#17292=CARTESIAN_POINT ( 'NONE',  ( 0.1787899950787401604, -1.726501920985144656, -0.07405724077823318263 ) ) ;
#17294=CARTESIAN_POINT ( 'NONE',  ( -0.1264236179284866091, -0.5959645668753701386, -0.1264236179284866091 ) ) ;
#17298=CARTESIAN_POINT ( 'NONE',  ( 0.1787899950787401604, -0.6919291338045056028, 0.07405724077823318263 ) ) ;
#17303=CARTESIAN_POINT ( 'NONE',  ( -0.1787899950787401882, 0.02300595303060378252, 0.000000000000000000 ) ) ;
#17304=CARTESIAN_POINT ( 'NONE',  ( 0.1787899950787401604, 0.05118110241596821736, 0.07405724077823318263 ) ) ;
#17310=CARTESIAN_POINT ( 'NONE',  ( -0.1574803149606300301, -0.8961614173228339419, -0.06523048226347956391 ) ) ;
#17312=CARTESIAN_POINT ( 'NONE',  ( 0.1797182628040039365, -1.674256408008242047, -2.200913952912460540E-17 ) ) ;
#17313=CARTESIAN_POINT ( 'NONE',  ( -0.1787899950787401604, -0.3917322834108032947, 0.07405724077823318263 ) ) ;
#17315=CARTESIAN_POINT ( 'NONE',  ( 0.1854001451104992926, 0.08095196624128539464, -0.1783922471787993125 ) ) ;
#17322=CARTESIAN_POINT ( 'NONE',  ( 0.07405724077823318263, -0.05708661411946481384, -0.1787899950787401604 ) ) ;
#17324=CARTESIAN_POINT ( 'NONE',  ( 0.07405724077823318263, -0.9183070865604088251, -0.1787899950787401604 ) ) ;
#17329=ORIENTED_EDGE ( 'NONE', *, *, #2117, .T. ) ;
#17332=CARTESIAN_POINT ( 'NONE',  ( 2.892866454678787531E-17, -1.149606299105070839, 0.1574803149606299191 ) ) ;
#17343=CARTESIAN_POINT ( 'NONE',  ( 0.1264236179284866091, 0.1274606299750234428, 0.1264236179284866091 ) ) ;
#17351=CARTESIAN_POINT ( 'NONE',  ( -0.1787899950787401882, -1.197466487914277566, 0.000000000000000000 ) ) ;
#17353=CARTESIAN_POINT ( 'NONE',  ( -0.1787899950787401604, -0.1161417322297011862, 0.07405724077823318263 ) ) ;
#17370=CARTESIAN_POINT ( 'NONE',  ( 0.1787899950787401604, 0.02165354336085011100, -0.07405724077823318263 ) ) ;
#17384=CARTESIAN_POINT ( 'NONE',  ( 0.1787899950787401604, -0.09645669285962235606, -0.07405724077823318263 ) ) ;
#17394=CARTESIAN_POINT ( 'NONE',  ( 0.07405724077823318263, -1.646653543253324026, 0.1787899950787401604 ) ) ;
#17401=CARTESIAN_POINT ( 'NONE',  ( -0.1787899950787401604, -0.6831948343709717264, 0.07405724077823318263 ) ) ;
#17403=CARTESIAN_POINT ( 'NONE',  ( -0.01513468283956021648, -0.08956185498306418191, 0.1527452548388714693 ) ) ;
#17404=DIRECTION ( 'NONE',  ( 1.000000000000000000, 0.000000000000000000, -2.392722035830075028E-16 ) ) ;
#17413=DIRECTION ( 'NONE',  ( 0.000000000000000000, -1.000000000000000000, 0.000000000000000000 ) ) ;
#17420=CARTESIAN_POINT ( 'NONE',  ( -0.07444174185955065859, -0.8991579828113921424, 0.1797182628040039087 ) ) ;
#17424=CARTESIAN_POINT ( 'NONE',  ( -0.1113553986120547346, -0.5738188976377952555, 0.1113553986120547346 ) ) ;
#17429=CARTESIAN_POINT ( 'NONE',  ( -9.642888182262618425E-18, 0.09055118120988918384, -0.1574803149606299191 ) ) ;
#17433=CARTESIAN_POINT ( 'NONE',  ( -9.642888182262618425E-18, -0.6574803148531023211, -0.1574803149606299191 ) ) ;
#17437=CARTESIAN_POINT ( 'NONE',  ( -0.1264236179284866091, -0.6353346456155275490, -0.1264236179284866091 ) ) ;
#17445=CARTESIAN_POINT ( 'NONE',  ( -0.1797182628040039365, 0.03834201718860799635, 0.000000000000000000 ) ) ;
#17446=CARTESIAN_POINT ( 'NONE',  ( 0.1787899950787401882, -1.088090551127338657, -2.189545951927503898E-17 ) ) ;
#17447=CARTESIAN_POINT ( 'NONE',  ( -0.1574803149606299191, -1.523622047244094446, 0.000000000000000000 ) ) ;
#17463=CARTESIAN_POINT ( 'NONE',  ( 0.1787899950787401882, -0.3116397162607351112, -2.189545951927503898E-17 ) ) ;
#17466=CARTESIAN_POINT ( 'NONE',  ( 0.000000000000000000, 0.1102362204724409434, 0.000000000000000000 ) ) ;
#17472=CARTESIAN_POINT ( 'NONE',  ( -1.094772975963752103E-17, -1.235728346402928945, -0.1787899950787401882 ) ) ;
#17473=CARTESIAN_POINT ( 'NONE',  ( -0.07405724077823318263, -1.449803149552535642, 0.1787899950787401604 ) ) ;
#17478=CARTESIAN_POINT ( 'NONE',  ( 0.1270800023317771588, -0.4587052269058803367, 0.1270800023317771588 ) ) ;
#17481=CARTESIAN_POINT ( 'NONE',  ( -0.1574803149606297803, -0.1825787401574804625, 0.06523048226347956391 ) ) ;
#17496=CARTESIAN_POINT ( 'NONE',  ( -0.1264236179284866091, -0.5221456692375747721, -0.1264236179284866091 ) ) ;
#17497=CARTESIAN_POINT ( 'NONE',  ( -0.1574803149606297803, -1.009350393700786608, 0.06523048226347956391 ) ) ;
#17501=ORIENTED_EDGE ( 'NONE', *, *, #26383, .T. ) ;
#17502=EDGE_LOOP ( 'NONE', ( #26926, #27649, #41815 ) ) ;
#17506=CARTESIAN_POINT ( 'NONE',  ( 2.892866454678787531E-17, -1.267716535325543070, 0.1574803149606299191 ) ) ;
#17511=CARTESIAN_POINT ( 'NONE',  ( 0.1925175471591499543, -0.07678538764768121083, 0.1742829424377221881 ) ) ;
#17513=CARTESIAN_POINT ( 'NONE',  ( -0.1113553986120547346, -0.1407480313885360323, -0.1113553986120547346 ) ) ;
#17515=DIRECTION ( 'NONE',  ( 0.000000000000000000, 0.000000000000000000, 1.000000000000000000 ) ) ;
#17518=CARTESIAN_POINT ( 'NONE',  ( -0.1490661257827161357, -0.09851383790554034403, -0.1002053949427159502 ) ) ;
#17525=CARTESIAN_POINT ( 'NONE',  ( -0.07405724077823318263, -0.6771653542769455747, -0.1787899950787401604 ) ) ;
#17532=CARTESIAN_POINT ( 'NONE',  ( 0.1264236179284866091, -0.3056102361667090705, 0.1264236179284866091 ) ) ;
#17537=CARTESIAN_POINT ( 'NONE',  ( -0.1264236179284866091, 0.02792721287312346923, 0.1264236179284866091 ) ) ;
#17538=CARTESIAN_POINT ( 'NONE',  ( -0.1787899950787401604, -0.2391732282926934683, -0.07405724077823318263 ) ) ;
#17544=CARTESIAN_POINT ( 'NONE',  ( -0.06523048226347956391, -0.8469488188976374010, 0.1574803149606297803 ) ) ;
#17546=CARTESIAN_POINT ( 'NONE',  ( -1.100456976456230270E-17, -1.664413888323202695, -0.1797182628040039365 ) ) ;
#17549=CARTESIAN_POINT ( 'NONE',  ( 0.1631888523360092158, 0.09129006187719292120, -0.1912159430412007366 ) ) ;
#17555=CARTESIAN_POINT ( 'NONE',  ( -0.1787899950787401604, -0.1604330708123782034, 0.07405724077823318263 ) ) ;
#17557=CARTESIAN_POINT ( 'NONE',  ( 0.1787899950787401604, -1.085629921206079374, 0.07405724077823318263 ) ) ;
#17578=CARTESIAN_POINT ( 'NONE',  ( -0.1264236179284866091, -0.07923228341080333637, 0.1264236179284866091 ) ) ;
#17584=CARTESIAN_POINT ( 'NONE',  ( -0.2471922904502827922, 0.06732389326667123641, -0.09794877975412334681 ) ) ;
#17587=CARTESIAN_POINT ( 'NONE',  ( -1.094772975963752103E-17, -1.286049165079631962, -0.1787899950787401882 ) ) ;
#17588=ORIENTED_EDGE ( 'NONE', *, *, #13812, .F. ) ;
#17589=CARTESIAN_POINT ( 'NONE',  ( 0.07405724077823318263, -0.06692913380450424277, 0.1787899950787401604 ) ) ;
#17595=CARTESIAN_POINT ( 'NONE',  ( -0.2471920270788468266, -0.07566776403313510424, 0.08167830084061132589 ) ) ;
#17597=CARTESIAN_POINT ( 'NONE',  ( -0.07405724077823318263, -1.494094488135213394, 0.1787899950787401604 ) ) ;
#17598=CARTESIAN_POINT ( 'NONE',  ( -1.094772975963752103E-17, -0.7239173227808818334, -0.1787899950787401882 ) ) ;
#17605=CARTESIAN_POINT ( 'NONE',  ( 2.700008691033534577E-17, 0.1102362204724409434, 0.2204724409448818867 ) ) ;
#17608=CARTESIAN_POINT ( 'NONE',  ( 0.1574803149606300301, -0.7878937006798749643, 0.06523048226347956391 ) ) ;
#17610=CARTESIAN_POINT ( 'NONE',  ( 0.07405724077823318263, -0.01279527553678768380, -0.1787899950787401604 ) ) ;
#17626=CARTESIAN_POINT ( 'NONE',  ( 0.1787899950787401882, -0.05954724404072461036, -2.189545951927503898E-17 ) ) ;
#17636=CARTESIAN_POINT ( 'NONE',  ( -0.1787899950787401604, -1.735236220418678643, 0.07405724077823318263 ) ) ;
#17644=CARTESIAN_POINT ( 'NONE',  ( 0.000000000000000000, 0.09842519685039370636, 0.000000000000000000 ) ) ;
#17645=CARTESIAN_POINT ( 'NONE',  ( 0.1264236179284866091, -0.8578995587804193468, -0.1264236179284866091 ) ) ;
#17647=CARTESIAN_POINT ( 'NONE',  ( -0.1429330575240212731, -0.08956165177108092734, 0.08068231488144075869 ) ) ;
#17659=CARTESIAN_POINT ( 'NONE',  ( 0.1270800023317771588, -0.7736658568271397307, 0.1270800023317771588 ) ) ;
#17660=CARTESIAN_POINT ( 'NONE',  ( 0.2471922904502826257, 0.08342621139837362587, 0.06611980121264769694 ) ) ;
#17663=CARTESIAN_POINT ( 'NONE',  ( 0.1574803149606300301, -0.5959645669291335768, -0.06523048226347956391 ) ) ;
#17664=CARTESIAN_POINT ( 'NONE',  ( -0.1596048934580996670, 0.1255079988737376195, -0.03370813687491143462 ) ) ;
#17679=CARTESIAN_POINT ( 'NONE',  ( -0.1270800023317771588, 0.03342075734608830617, -0.1270800023317771588 ) ) ;
#17680=CARTESIAN_POINT ( 'NONE',  ( -0.1787899950787401604, -1.070866141678519456, -0.07405724077823318263 ) ) ;
#17681=CARTESIAN_POINT ( 'NONE',  ( 0.1113553986120547346, -1.499015748031496065, -0.1113553986120547346 ) ) ;
#17702=CARTESIAN_POINT ( 'NONE',  ( -0.1787899950787401882, -0.2919546768906559064, 0.000000000000000000 ) ) ;
#17704=DIRECTION ( 'NONE',  ( 0.000000000000000000, 1.000000000000000000, 0.000000000000000000 ) ) ;
#17709=CARTESIAN_POINT ( 'NONE',  ( -0.1787899950787401604, -1.223425196796630532, 0.07405724077823318263 ) ) ;
#17710=CARTESIAN_POINT ( 'NONE',  ( -0.1787899950787401882, -1.378444881836000002, 0.000000000000000000 ) ) ;
#17714=CARTESIAN_POINT ( 'NONE',  ( 0.07444174185955046430, -0.6432524710003691970, -0.1797182628040039087 ) ) ;
#17719=CARTESIAN_POINT ( 'NONE',  ( 0.1574803149606299191, -0.1653543307086614012, -1.928577636452523993E-17 ) ) ;
#17725=CONICAL_SURFACE ( 'NONE', #36855, 0.2471922904502826812, 0.5235987755982992597 ) ;
#17730=CARTESIAN_POINT ( 'NONE',  ( 0.07405724077823318263, -0.06692913380450424277, 0.1787899950787401604 ) ) ;
#17732=CARTESIAN_POINT ( 'NONE',  ( 0.1113553986120547346, -1.459645669183811112, 0.1113553986120547346 ) ) ;
#17733=CARTESIAN_POINT ( 'NONE',  ( 0.1787899950787401604, -0.5738188975840317063, -0.07405724077823318263 ) ) ;
#17734=CARTESIAN_POINT ( 'NONE',  ( -0.1113553986120547346, -1.085629921259842590, 0.1113553986120547346 ) ) ;
#17752=AXIS2_PLACEMENT_3D ( 'NONE', #12028, #4805, #26653 ) ;
#17753=CARTESIAN_POINT ( 'NONE',  ( 0.1465245066989980804, -0.09658349877441907427, 0.2008369897434355567 ) ) ;
#17757=CARTESIAN_POINT ( 'NONE',  ( -0.1574803149606300301, -0.2563976376877486474, -0.06523048226347956391 ) ) ;
#17769=CARTESIAN_POINT ( 'NONE',  ( -0.1264236179284866091, -0.3548228345919058890, 0.1264236179284866091 ) ) ;
#17770=CARTESIAN_POINT ( 'NONE',  ( 0.07405724077823318263, -0.8789370078202529690, -0.1787899950787401604 ) ) ;
#17776=CARTESIAN_POINT ( 'NONE',  ( -1.094772975963752103E-17, -0.1836869603552232222, -0.1787899950787401882 ) ) ;
#17784=CARTESIAN_POINT ( 'NONE',  ( -0.07444174185955065859, -1.701323337142099934, -0.1797182628040039087 ) ) ;
#17786=CARTESIAN_POINT ( 'NONE',  ( 0.07405724077823318263, -0.4458661416785199560, -0.1787899950787401604 ) ) ;
#17789=CARTESIAN_POINT ( 'NONE',  ( 0.2272550450523252441, 0.05212746764700336433, -0.1542273094304812131 ) ) ;
#17795=CARTESIAN_POINT ( 'NONE',  ( 0.07405724077823318263, -0.07185039364702387743, 0.1787899950787401604 ) ) ;
#17798=CARTESIAN_POINT ( 'NONE',  ( -0.1264236179284866091, -1.029035433017102319, -0.1264236179284866091 ) ) ;
#17820=CARTESIAN_POINT ( 'NONE',  ( 0.07405724077823318263, -0.05708661411946481384, -0.1787899950787401604 ) ) ;
#17826=CARTESIAN_POINT ( 'NONE',  ( -0.2471922904502827090, 0.08082342248659966921, -0.07163232281567466497 ) ) ;
#17828=CARTESIAN_POINT ( 'NONE',  ( 0.1787899950787401604, -1.372171212323726852, -0.07405724077823318263 ) ) ;
#17830=CARTESIAN_POINT ( 'NONE',  ( -0.1787899950787401604, -0.2736220471903310081, 0.07405724077823318263 ) ) ;
#17836=CARTESIAN_POINT ( 'NONE',  ( -0.2471920410536367907, -0.09140649424435846881, 0.04498895533817294512 ) ) ;
#17839=CARTESIAN_POINT ( 'NONE',  ( -0.1787899950787401604, -1.617125984198204414, 0.07405724077823318263 ) ) ;
#17861=CARTESIAN_POINT ( 'NONE',  ( 2.892866454678787531E-17, -1.031496062884598386, 0.1574803149606299191 ) ) ;
#17866=CARTESIAN_POINT ( 'NONE',  ( -1.094772975963752103E-17, -0.08907480309584270284, -0.1787899950787401882 ) ) ;
#17871=CARTESIAN_POINT ( 'NONE',  ( 0.1435836963516304854, -0.09660391682274863112, -0.2025327002555687705 ) ) ;
#17874=CARTESIAN_POINT ( 'NONE',  ( -0.1574803149606299191, 0.06102362215477106361, 0.000000000000000000 ) ) ;
#17882=CARTESIAN_POINT ( 'NONE',  ( -1.094772975963752103E-17, -0.7742381414575847387, -0.1787899950787401882 ) ) ;
#17884=CARTESIAN_POINT ( 'NONE',  ( -0.1007914167158820845, -0.08956157794326476129, 0.1244328764867059095 ) ) ;
#17898=CARTESIAN_POINT ( 'NONE',  ( 0.07444174185955046430, -0.8794729434413131042, -0.1797182628040039087 ) ) ;
#17902=CARTESIAN_POINT ( 'NONE',  ( -0.08069314021478943277, 0.1221948107111021781, -0.1379473356501541015 ) ) ;
#17911=CARTESIAN_POINT ( 'NONE',  ( -0.1787899950787401882, -0.6304133857730078727, 0.000000000000000000 ) ) ;
#17919=CARTESIAN_POINT ( 'NONE',  ( -0.1787899950787401604, -1.262795275536788386, 0.07405724077823318263 ) ) ;
#17920=CARTESIAN_POINT ( 'NONE',  ( -0.1113553986120547346, -1.518700787401574770, 0.1113553986120547346 ) ) ;
#17929=CARTESIAN_POINT ( 'NONE',  ( -0.2471922904502825424, 0.07573437638786091608, 0.08155181604443949295 ) ) ;
#17934=CARTESIAN_POINT ( 'NONE',  ( 0.1264236179284866091, -0.3460885351583728453, -0.1264236179284866091 ) ) ;
#17935=CARTESIAN_POINT ( 'NONE',  ( -0.04622344188396850656, -0.09842519685039370636, 0.1526493060429974513 ) ) ;
#17941=CARTESIAN_POINT ( 'NONE',  ( -0.07405724077823318263, -1.139763779473794925, 0.1787899950787401604 ) ) ;
#17942=CARTESIAN_POINT ( 'NONE',  ( -0.1787899950787401604, -1.336614173174582865, 0.07405724077823318263 ) ) ;
#17950=CARTESIAN_POINT ( 'NONE',  ( -9.642888182262618425E-18, -0.07677165354330708902, -0.1574803149606299191 ) ) ;
#17963=CARTESIAN_POINT ( 'NONE',  ( 0.1787899950787401882, -0.05954724404072461036, -2.189545951927503898E-17 ) ) ;
#17967=CARTESIAN_POINT ( 'NONE',  ( -0.1574803149606299191, -1.592519684931842372, 0.000000000000000000 ) ) ;
#17968=CARTESIAN_POINT ( 'NONE',  ( -0.07405724077823318263, -0.7854330708123791194, 0.1787899950787401604 ) ) ;
#17970=CARTESIAN_POINT ( 'NONE',  ( 0.06523048226347956391, -0.9995078740157482544, 0.1574803149606297803 ) ) ;
#17987=CARTESIAN_POINT ( 'NONE',  ( -0.06523048226347956391, -0.1678149605223941132, 0.1574803149606297803 ) ) ;
#17990=AXIS2_PLACEMENT_3D ( 'NONE', #24374, #17404, #2084 ) ;
#17999=CARTESIAN_POINT ( 'NONE',  ( 0.1264236179284866091, -0.6845472440407243120, -0.1264236179284866091 ) ) ;
#18000=EDGE_LOOP ( 'NONE', ( #40259, #36438, #22743, #25164, #10477, #8132 ) ) ;
#18002=CARTESIAN_POINT ( 'NONE',  ( -0.1787899950787401604, -0.4015748030958427028, -0.07405724077823318263 ) ) ;
#18003=CARTESIAN_POINT ( 'NONE',  ( 0.07405724077823318263, -0.9576771653005667906, -0.1787899950787401604 ) ) ;
#18006=CARTESIAN_POINT ( 'NONE',  ( -0.1797182628040039365, -0.1191382977720218533, 0.000000000000000000 ) ) ;
#18008=CARTESIAN_POINT ( 'NONE',  ( 0.1787899950787401882, -0.1147893225599474487, -2.189545951927503898E-17 ) ) ;
#18009=CARTESIAN_POINT ( 'NONE',  ( -0.07405724077823318263, -0.2834645668753703052, -0.1787899950787401604 ) ) ;
#18010=CARTESIAN_POINT ( 'NONE',  ( -0.1264236179284866091, -0.08907480309584270284, -0.1264236179284866091 ) ) ;
#18011=CARTESIAN_POINT ( 'NONE',  ( 0.2471911249972296165, -0.08424752482839464873, -0.06442904123614238976 ) ) ;
#18018=CARTESIAN_POINT ( 'NONE',  ( 0.1797182628040039087, -1.676717037929501775, 0.07444174185955046430 ) ) ;
#18022=CARTESIAN_POINT ( 'NONE',  ( 3.284318927891251994E-17, -0.4630905511273386010, 0.1787899950787401882 ) ) ;
#18031=CARTESIAN_POINT ( 'NONE',  ( -0.07405724077823318263, -0.05216535427694517224, -0.1787899950787401604 ) ) ;
#18034=CARTESIAN_POINT ( 'NONE',  ( 3.284318927891251994E-17, -1.093011810969858333, 0.1787899950787401882 ) ) ;
#18042=CARTESIAN_POINT ( 'NONE',  ( -9.642888182262618425E-18, -1.129921259734992134, -0.1574803149606299191 ) ) ;
#18052=CARTESIAN_POINT ( 'NONE',  ( 0.1787899950787401604, -0.02755905506434671789, 0.07405724077823318263 ) ) ;
#18060=CARTESIAN_POINT ( 'NONE',  ( -0.07405724077823318263, -1.347564913111128471, 0.1787899950787401604 ) ) ;
#18062=CARTESIAN_POINT ( 'NONE',  ( 0.1264236179284866091, -0.2121062991588350544, -0.1264236179284866091 ) ) ;
#18071=CARTESIAN_POINT ( 'NONE',  ( 3.284318927891251994E-17, -1.649114173174582643, 0.1787899950787401882 ) ) ;
#18072=CARTESIAN_POINT ( 'NONE',  ( -0.07405724077823318263, -0.7066929133320629663, 0.1787899950787401604 ) ) ;
#18074=DIRECTION ( 'NONE',  ( 0.000000000000000000, -1.000000000000000000, 0.000000000000000000 ) ) ;
#18075=CARTESIAN_POINT ( 'NONE',  ( 0.07444174185955065859, -1.287937510370446903, 0.1797182628040039087 ) ) ;
#18084=CARTESIAN_POINT ( 'NONE',  ( 0.06523048226347956391, -0.7780511809948342794, -0.1574803149606300301 ) ) ;
#18105=CARTESIAN_POINT ( 'NONE',  ( -0.1264236179284866091, 0.03395669296714932950, -0.1264236179284866091 ) ) ;
#18114=CARTESIAN_POINT ( 'NONE',  ( 0.06523048226347956391, 0.07332677176107038619, 0.1574803149606297803 ) ) ;
#18120=CARTESIAN_POINT ( 'NONE',  ( 0.1787899950787401604, -0.8209901099615228848, -0.07405724077823318263 ) ) ;
#18122=CARTESIAN_POINT ( 'NONE',  ( -0.06523048226347956391, -0.01033464556176428781, 0.1574803149606297803 ) ) ;
#18130=EDGE_CURVE ( 'NONE', #26779, #43256, #16778, .T. ) ;
#18132=ORIENTED_EDGE ( 'NONE', *, *, #16320, .T. ) ;
#18136=CARTESIAN_POINT ( 'NONE',  ( -1.100456976456230270E-17, -0.8770123135200531550, -0.1797182628040039365 ) ) ;
#18142=CARTESIAN_POINT ( 'NONE',  ( 2.892866454678787531E-17, -0.6082677165354331006, 0.1574803149606299191 ) ) ;
#18144=CARTESIAN_POINT ( 'NONE',  ( 2.892866454678787531E-17, 0.02165354330708661734, 0.1574803149606299191 ) ) ;
#18149=CARTESIAN_POINT ( 'NONE',  ( 0.1574803149606300301, -0.6304133857192448787, 0.06523048226347956391 ) ) ;
#18154=CARTESIAN_POINT ( 'NONE',  ( -0.07405724077823318263, -0.6771653542769455747, -0.1787899950787401604 ) ) ;
#18161=CARTESIAN_POINT ( 'NONE',  ( -0.1787899950787401604, -1.144685039316316599, 0.07405724077823318263 ) ) ;
#18162=CARTESIAN_POINT ( 'NONE',  ( -0.1574803149606300301, -1.447342519685039797, -0.06523048226347956391 ) ) ;
#18163=DIRECTION ( 'NONE',  ( 0.000000000000000000, -1.000000000000000000, 0.000000000000000000 ) ) ;
#18167=ORIENTED_EDGE ( 'NONE', *, *, #31349, .T. ) ;
#18168=CARTESIAN_POINT ( 'NONE',  ( -0.1113553986120547346, -0.3277559054042838982, 0.1113553986120547346 ) ) ;
#18169=CARTESIAN_POINT ( 'NONE',  ( -0.1264236179284866091, -1.427657480261196987, -0.1264236179284866091 ) ) ;
#18176=CARTESIAN_POINT ( 'NONE',  ( 0.06218625040858925118, 0.08128102204192401425, -0.2495298224528492981 ) ) ;
#18178=CARTESIAN_POINT ( 'NONE',  ( 0.07405724077823318263, -0.4765019209851441007, 0.1787899950787401604 ) ) ;
#18179=CARTESIAN_POINT ( 'NONE',  ( -0.1729392868700769803, -0.09842519685039370636, -0.02639094656065850072 ) ) ;
#18191=CARTESIAN_POINT ( 'NONE',  ( 0.1787899950787401604, -1.203740157426551383, -0.07405724077823318263 ) ) ;
#18192=CARTESIAN_POINT ( 'NONE',  ( -0.1787899950787401604, -1.420275590497418250, -0.07405724077823318263 ) ) ;
#18196=CARTESIAN_POINT ( 'NONE',  ( -0.1797182628040039365, -0.6309493213940688960, 0.000000000000000000 ) ) ;
#18200=CARTESIAN_POINT ( 'NONE',  ( -9.642888182262618425E-18, -0.1161417322834645688, -0.1574803149606299191 ) ) ;
#18205=CARTESIAN_POINT ( 'NONE',  ( -0.1574803149606299191, -0.06692913385826770867, 0.000000000000000000 ) ) ;
#18212=CARTESIAN_POINT ( 'NONE',  ( -0.1787899950787401604, -1.533464566875370805, 0.07405724077823318263 ) ) ;
#18213=CARTESIAN_POINT ( 'NONE',  ( 0.06523048226347956391, -1.526082677057828629, -0.1574803149606300301 ) ) ;
#18214=CARTESIAN_POINT ( 'NONE',  ( -0.07405724077823318263, -0.7214566928596228834, -0.1787899950787401604 ) ) ;
#18216=CARTESIAN_POINT ( 'NONE',  ( -9.642888182262618425E-18, -0.9822834645669291653, -0.1574803149606299191 ) ) ;
#18236=CARTESIAN_POINT ( 'NONE',  ( 0.1577183631698106381, -0.09851384455655413930, -0.1232999193531017779 ) ) ;
#18246=CARTESIAN_POINT ( 'NONE',  ( 0.1787899950787401604, -0.3818897637257640532, 0.07405724077823318263 ) ) ;
#18247=CARTESIAN_POINT ( 'NONE',  ( -0.1787899950787401604, -0.9084645668753701386, -0.07405724077823318263 ) ) ;
#18252=CARTESIAN_POINT ( 'NONE',  ( 0.07444174185955065859, -0.2249453843861952684, 0.1797182628040039087 ) ) ;
#18253=CARTESIAN_POINT ( 'NONE',  ( 3.284318927891251994E-17, -0.08526176350482933541, 0.1787899950787401882 ) ) ;
#18254=CARTESIAN_POINT ( 'NONE',  ( -0.1787899950787401882, -0.2367125983714334636, 0.000000000000000000 ) ) ;
#18255=CARTESIAN_POINT ( 'NONE',  ( 0.1787899950787401604, -0.06200787396198446239, -0.07405724077823318263 ) ) ;
#18262=CARTESIAN_POINT ( 'NONE',  ( -0.1435836963511328279, -0.09660391682274867275, 0.2025327002559215717 ) ) ;
#18268=CARTESIAN_POINT ( 'NONE',  ( -0.07405724077823318263, -0.2736220471903310081, 0.1787899950787401604 ) ) ;
#18272=CARTESIAN_POINT ( 'NONE',  ( -0.1787899950787401604, -1.026574803095842370, -0.07405724077823318263 ) ) ;
#18291=ORIENTED_EDGE ( 'NONE', *, *, #25596, .T. ) ;
#18293=CARTESIAN_POINT ( 'NONE',  ( -1.094772975963752103E-17, 0.06348425202226751218, -0.1787899950787401882 ) ) ;
#18299=ORIENTED_EDGE ( 'NONE', *, *, #20943, .F. ) ;
#18301=CARTESIAN_POINT ( 'NONE',  ( 0.1264236179284866091, -1.261442865867033580, 0.1264236179284866091 ) ) ;
#18303=CARTESIAN_POINT ( 'NONE',  ( -0.1787899950787401604, -0.3523622046706461619, 0.07405724077823318263 ) ) ;
#18313=CARTESIAN_POINT ( 'NONE',  ( -0.07405724077823318263, -1.690944881836001334, 0.1787899950787401604 ) ) ;
#18314=CARTESIAN_POINT ( 'NONE',  ( 0.1787899950787401604, -1.631889763725764553, -0.07405724077823318263 ) ) ;
#18318=CARTESIAN_POINT ( 'NONE',  ( 0.1797182628040039365, -1.319925699346824688, -2.200913952912460540E-17 ) ) ;
#18343=CARTESIAN_POINT ( 'NONE',  ( 0.07405724077823318263, -0.2096456692375751329, -0.1787899950787401604 ) ) ;
#18350=CARTESIAN_POINT ( 'NONE',  ( 0.1113553986120547346, 0.04625984262721204859, -0.1113553986120547346 ) ) ;
#18360=CARTESIAN_POINT ( 'NONE',  ( 0.1264236179284866091, -0.8185294800402619364, -0.1264236179284866091 ) ) ;
#18371=CARTESIAN_POINT ( 'NONE',  ( 0.1787899950787401604, -0.4999999999462365619, 0.07405724077823318263 ) ) ;
#18374=CARTESIAN_POINT ( 'NONE',  ( -0.1270800023317771588, -0.8228784552523366047, 0.1270800023317771588 ) ) ;
#18384=CARTESIAN_POINT ( 'NONE',  ( -0.06523048226347956391, -0.6156496061916855167, -0.1574803149606300301 ) ) ;
#18387=CARTESIAN_POINT ( 'NONE',  ( -0.1787899950787401882, -0.8272637794737952577, 0.000000000000000000 ) ) ;
#18395=CARTESIAN_POINT ( 'NONE',  ( 0.1113553986120547346, -1.626968503937007871, 0.1113553986120547346 ) ) ;
#18400=CARTESIAN_POINT ( 'NONE',  ( 0.06523048226347977208, 0.1028543307086613318, 0.1574803149606297803 ) ) ;
#18409=CARTESIAN_POINT ( 'NONE',  ( 0.1787899950787401882, -0.3903798737410496544, -2.189545951927503898E-17 ) ) ;
#18410=CARTESIAN_POINT ( 'NONE',  ( -0.1674188814857066887, -0.09842519685039370636, 0.03545433526083362208 ) ) ;
#18412=CIRCLE ( 'NONE', #32979, 0.2007874015748031815 ) ;
#18419=CARTESIAN_POINT ( 'NONE',  ( 0.1264236179284866091, -1.353838582623401621, -0.1264236179284866091 ) ) ;
#18421=CARTESIAN_POINT ( 'NONE',  ( 0.07444174185955065859, -0.5792760930476124059, 0.1797182628040039087 ) ) ;
#18424=CARTESIAN_POINT ( 'NONE',  ( -0.06523048226347956391, -0.3105314960629923515, -0.1574803149606300301 ) ) ;
#18437=ORIENTED_EDGE ( 'NONE', *, *, #31349, .F. ) ;
#18441=CARTESIAN_POINT ( 'NONE',  ( -0.1264236179284866091, -1.570374015694267600, 0.1264236179284866091 ) ) ;
#18442=CARTESIAN_POINT ( 'NONE',  ( 0.1574803149606299191, -1.454724409341291436, -1.928577636452523993E-17 ) ) ;
#18443=CARTESIAN_POINT ( 'NONE',  ( -0.1787899950787401604, -0.6722440944344262315, 0.07405724077823318263 ) ) ;
#18446=CARTESIAN_POINT ( 'NONE',  ( 0.1113553986120547346, -1.075787401574803015, 0.1113553986120547346 ) ) ;
#18451=ORIENTED_EDGE ( 'NONE', *, *, #25927, .F. ) ;
#18454=EDGE_CURVE ( 'NONE', #35946, #24004, #36775, .T. ) ;
#18456=CARTESIAN_POINT ( 'NONE',  ( 0.1574803149606299191, -1.336614173120818760, -1.928577636452523993E-17 ) ) ;
#18462=CARTESIAN_POINT ( 'NONE',  ( 0.1574803149606299191, -0.07677165343578011558, -1.928577636452523993E-17 ) ) ;
#18466=ORIENTED_EDGE ( 'NONE', *, *, #19582, .T. ) ;
#18479=CARTESIAN_POINT ( 'NONE',  ( -0.1787899950787401882, -0.4384842519147402196, 0.000000000000000000 ) ) ;
#18480=CARTESIAN_POINT ( 'NONE',  ( 0.1787899950787401604, -0.8887795275052913224, 0.07405724077823318263 ) ) ;
#18484=CARTESIAN_POINT ( 'NONE',  ( -0.1270800023317771588, -0.2027997150948566696, -0.1270800023317771588 ) ) ;
#18485=CARTESIAN_POINT ( 'NONE',  ( 0.1264236179284866091, -0.1098680627174277585, -0.1264236179284866091 ) ) ;
#18486=CARTESIAN_POINT ( 'NONE',  ( -0.1264236179284866091, -0.07923228341080333637, 0.1264236179284866091 ) ) ;
#18490=CARTESIAN_POINT ( 'NONE',  ( -0.07405724077823318263, -0.4261811023084413064, 0.1787899950787401604 ) ) ;
#18493=CARTESIAN_POINT ( 'NONE',  ( -0.2275913475554304233, -0.05179116514389500714, 0.1540331450897821919 ) ) ;
#18498=CARTESIAN_POINT ( 'NONE',  ( 0.07405724077823318263, -0.2145669290800947537, -0.1787899950787401604 ) ) ;
#18501=CARTESIAN_POINT ( 'NONE',  ( -0.1787899950787401604, -1.144685039316316599, -0.07405724077823318263 ) ) ;
#18510=CARTESIAN_POINT ( 'NONE',  ( 0.06523048226347956391, -1.171751968396410382, -0.1574803149606300301 ) ) ;
#18523=CARTESIAN_POINT ( 'NONE',  ( -1.094772975963752103E-17, -0.05462598419820496182, -0.1787899950787401882 ) ) ;
#18529=CARTESIAN_POINT ( 'NONE',  ( -0.1787899950787401604, -1.318037354056011079, -0.07405724077823318263 ) ) ;
#18531=CARTESIAN_POINT ( 'NONE',  ( 0.1787899950787401604, -0.2933070865604095467, -0.07405724077823318263 ) ) ;
#18542=CARTESIAN_POINT ( 'NONE',  ( -0.07405724077823318263, -1.661417322780881500, -0.1787899950787401604 ) ) ;
#18546=CARTESIAN_POINT ( 'NONE',  ( -0.1797182628040039087, -1.420811526118478829, -0.07444174185955065859 ) ) ;
#18550=CARTESIAN_POINT ( 'NONE',  ( -0.09075913361134779755, 0.1299212598425197318, 0.1419506277346105627 ) ) ;
#18567=CARTESIAN_POINT ( 'NONE',  ( 0.07444174185955065859, 0.1293853242752222577, 0.1797182628040039087 ) ) ;
#18568=CARTESIAN_POINT ( 'NONE',  ( -0.1574803149606299191, -1.041338582569637738, 0.000000000000000000 ) ) ;
#18572=CARTESIAN_POINT ( 'NONE',  ( 0.1787899950787401604, -0.2145669290800947537, -0.07405724077823318263 ) ) ;
#18575=CARTESIAN_POINT ( 'NONE',  ( -0.1113553986120547346, 0.09547244094488190058, 0.1113553986120547346 ) ) ;
#18579=CARTESIAN_POINT ( 'NONE',  ( 0.1574803149606300301, 0.1225393701862672879, -0.06523048226347956391 ) ) ;
#18586=CARTESIAN_POINT ( 'NONE',  ( 0.1787899950787401604, -0.8259113698040420060, 0.07405724077823318263 ) ) ;
#18588=CARTESIAN_POINT ( 'NONE',  ( -0.1787899950787401882, 0.1176181102899840625, 0.000000000000000000 ) ) ;
#18597=CARTESIAN_POINT ( 'NONE',  ( -0.07444174185955065859, -0.9778981402917082955, 0.1797182628040039087 ) ) ;
#18609=CLOSED_SHELL ( 'NONE', ( #44137, #33806, #26315, #31454, #12907, #7575, #1235, #26590, #193, #10387, #6615, #28218, #44450, #6240, #21210, #9646, #19421, #24622, #39481, #44938, #20166, #3636, #4262, #23528, #32286, #42455, #12207, #24359, #40977, #41083, #39539, #36631, #2208, #44402, #7208, #44707, #15883, #20131, #1609, #43994, #3736, #18876, #13479, #5635 ) ) ;
#18612=CARTESIAN_POINT ( 'NONE',  ( 0.07405724077823318263, -0.8149606298674965110, 0.1787899950787401604 ) ) ;
#18617=EDGE_CURVE ( 'NONE', #6678, #30540, #46892, .T. ) ;
#18619=CARTESIAN_POINT ( 'NONE',  ( 2.892866454678787531E-17, -1.671259842519685179, 0.1574803149606299191 ) ) ;
#18626=CARTESIAN_POINT ( 'NONE',  ( 0.1113553986120547346, 0.1151574803149606335, -0.1113553986120547346 ) ) ;
#18630=CARTESIAN_POINT ( 'NONE',  ( 0.06523048226347956391, -0.03001968493184305545, -0.1574803149606300301 ) ) ;
#18633=CARTESIAN_POINT ( 'NONE',  ( 0.08443540605192632886, 0.09133345722616725837, -0.2366842664529266727 ) ) ;
#18635=CARTESIAN_POINT ( 'NONE',  ( -0.1264236179284866091, -0.3756160942134905700, -0.1264236179284866091 ) ) ;
#18636=CARTESIAN_POINT ( 'NONE',  ( -0.1979409878709763870, -0.08955984950924253396, 0.1204397522454633829 ) ) ;
#18638=CARTESIAN_POINT ( 'NONE',  ( 2.892866454678787531E-17, 0.03149606309965303358, 0.1574803149606299191 ) ) ;
#18646=CARTESIAN_POINT ( 'NONE',  ( -0.1264236179284866091, -1.270177165300566902, -0.1264236179284866091 ) ) ;
#18647=CARTESIAN_POINT ( 'NONE',  ( -1.094772975963752103E-17, -1.467027559001354398, -0.1787899950787401882 ) ) ;
#18662=CARTESIAN_POINT ( 'NONE',  ( -0.1574803149606297803, -0.5270669290263310103, 0.06523048226347956391 ) ) ;
#18670=CARTESIAN_POINT ( 'NONE',  ( -1.094772975963752103E-17, -1.545767716481669218, -0.1787899950787401882 ) ) ;
#18671=CARTESIAN_POINT ( 'NONE',  ( 0.1264236179284866091, -0.8174212597887557941, 0.1264236179284866091 ) ) ;
#18672=CARTESIAN_POINT ( 'NONE',  ( -0.1113553986120547346, -1.134842519685039353, -0.1113553986120547346 ) ) ;
#18680=CARTESIAN_POINT ( 'NONE',  ( -0.1574803149606299191, -1.316929133750740055, 0.000000000000000000 ) ) ;
#18688=CARTESIAN_POINT ( 'NONE',  ( 0.08400343811432031682, 0.09129006187721050436, 0.2369336632579849278 ) ) ;
#18696=CARTESIAN_POINT ( 'NONE',  ( -0.2364432464758906005, -0.09842519685039370636, -0.06084591350176535296 ) ) ;
#18702=CARTESIAN_POINT ( 'NONE',  ( 0.1787899950787401604, -0.9675196849856075865, -0.07405724077823318263 ) ) ;
#18704=CARTESIAN_POINT ( 'NONE',  ( -0.1787899950787401604, -0.4409448818359998357, -0.07405724077823318263 ) ) ;
#18706=CARTESIAN_POINT ( 'NONE',  ( 0.07405724077823318263, -0.8937007873478103326, 0.1787899950787401604 ) ) ;
#18709=CARTESIAN_POINT ( 'NONE',  ( 0.1270800023317771588, -0.2224847544649354303, 0.1270800023317771588 ) ) ;
#18711=CARTESIAN_POINT ( 'NONE',  ( -0.06523048226347956391, 0.1225393700787401341, -0.1574803149606300301 ) ) ;
#18712=CARTESIAN_POINT ( 'NONE',  ( -0.07405724077823318263, -0.01279527553678766298, -0.1787899950787401604 ) ) ;
#18726=CARTESIAN_POINT ( 'NONE',  ( -0.1113553986120547346, -0.9675196849318424830, -0.1113553986120547346 ) ) ;
#18727=CARTESIAN_POINT ( 'NONE',  ( -0.07405724077823318263, -0.2490157479777327099, -0.1787899950787401604 ) ) ;
#18729=CARTESIAN_POINT ( 'NONE',  ( -0.1264236179284866091, -1.265255905458047225, -0.1264236179284866091 ) ) ;
#18747=ORIENTED_EDGE ( 'NONE', *, *, #21262, .F. ) ;
#18757=CARTESIAN_POINT ( 'NONE',  ( -0.1787899950787401604, -1.396777511536325234, -0.07405724077823318263 ) ) ;
#18758=ORIENTED_EDGE ( 'NONE', *, *, #32814, .F. ) ;
#18760=CARTESIAN_POINT ( 'NONE',  ( -1.094772975963752103E-17, -0.2465551180564728440, -0.1787899950787401882 ) ) ;
#18772=AXIS2_PLACEMENT_3D ( 'NONE', #26279, #22416, #11888 ) ;
#18773=CARTESIAN_POINT ( 'NONE',  ( -0.1787899950787401604, -1.695866141678520567, 0.07405724077823318263 ) ) ;
#18774=CARTESIAN_POINT ( 'NONE',  ( 0.1787899950787401882, -1.752460629867496067, -2.189545951927503898E-17 ) ) ;
#18779=CARTESIAN_POINT ( 'NONE',  ( -0.1270800023317771588, -1.344531998559423069, -0.1270800023317771588 ) ) ;
#18787=CARTESIAN_POINT ( 'NONE',  ( -0.1787899950787401604, 0.1496062992663619862, -0.07405724077823318263 ) ) ;
#18797=CARTESIAN_POINT ( 'NONE',  ( 0.07444174185955065859, 0.01127508805474972294, 0.1797182628040039087 ) ) ;
#18805=CARTESIAN_POINT ( 'NONE',  ( -0.07405724077823318263, -0.1653543306548978520, -0.1787899950787401604 ) ) ;
#18808=CARTESIAN_POINT ( 'NONE',  ( -0.08438807215028237829, -0.09131796649078639805, 0.2367113086201506622 ) ) ;
#18811=CARTESIAN_POINT ( 'NONE',  ( 0.06523048226347956391, 0.04872047254847188674, -0.1574803149606300301 ) ) ;
#18813=AXIS2_PLACEMENT_3D ( 'NONE', #17466, #17704, #43335 ) ;
#18820=CARTESIAN_POINT ( 'NONE',  ( 0.1264236179284866091, -0.9760097950008916889, -0.1264236179284866091 ) ) ;
#18822=CARTESIAN_POINT ( 'NONE',  ( -0.1264236179284866091, 0.1520669291876218521, -0.1264236179284866091 ) ) ;
#18829=CARTESIAN_POINT ( 'NONE',  ( 0.07405724077823318263, -0.5295275590013543976, -0.1787899950787401604 ) ) ;
#18834=CARTESIAN_POINT ( 'NONE',  ( -0.1270800023317771588, -0.9409886914728091689, 0.1270800023317771588 ) ) ;
#18843=DIRECTION ( 'NONE',  ( 0.000000000000000000, -1.000000000000000000, 0.000000000000000000 ) ) ;
#18846=CARTESIAN_POINT ( 'NONE',  ( -1.094772975963752103E-17, -0.7583661416785196785, -0.1787899950787401882 ) ) ;
#18849=CARTESIAN_POINT ( 'NONE',  ( 0.1574803149606299191, 0.1200787401574803237, 2.850509043694854679E-09 ) ) ;
#18851=CARTESIAN_POINT ( 'NONE',  ( 2.892866454678787531E-17, -1.631889763779527547, 0.1574803149606299191 ) ) ;
#18857=CARTESIAN_POINT ( 'NONE',  ( -9.642888182262618425E-18, 0.1200787401574803237, -0.1574803149606299191 ) ) ;
#18862=CARTESIAN_POINT ( 'NONE',  ( 0.1574803149606300301, -0.03986220461688239070, 0.06523048226347956391 ) ) ;
#18866=CARTESIAN_POINT ( 'NONE',  ( 0.000000000000000000, -0.09842519685039370636, 0.000000000000000000 ) ) ;
#18867=CARTESIAN_POINT ( 'NONE',  ( 0.07405724077823318263, -0.4617381414575855159, -0.1787899950787401604 ) ) ;
#18868=CARTESIAN_POINT ( 'NONE',  ( -0.2298521815382791322, -0.08955978675932835253, 0.05126285459619552010 ) ) ;
#18875=CARTESIAN_POINT ( 'NONE',  ( 0.1264236179284866091, -1.733883810748923171, 0.1264236179284866091 ) ) ;
#18876=ADVANCED_FACE ( 'NONE', ( #16217 ), #17725, .T. ) ;
#18882=CARTESIAN_POINT ( 'NONE',  ( 0.1787899950787401604, -1.282480314906867314, -0.07405724077823318263 ) ) ;
#18883=CARTESIAN_POINT ( 'NONE',  ( -0.1787899950787401604, -1.494094488135213394, 0.07405724077823318263 ) ) ;
#18892=CARTESIAN_POINT ( 'NONE',  ( -0.1113553986120547346, -0.2687007874015748254, -0.1113553986120547346 ) ) ;
#18895=CARTESIAN_POINT ( 'NONE',  ( -0.1287886813449822809, -0.09210284872765374387, -0.1240405425130319400 ) ) ;
#18900=CARTESIAN_POINT ( 'NONE',  ( -0.1695021356517113220, -0.08955111078152680482, -0.02025256367261695639 ) ) ;
#18907=CARTESIAN_POINT ( 'NONE',  ( -0.1787899950787401604, -1.572834645615527327, 0.07405724077823318263 ) ) ;
#18908=CARTESIAN_POINT ( 'NONE',  ( 0.1264236179284866091, -0.6993110235682834519, 0.1264236179284866091 ) ) ;
#18909=CARTESIAN_POINT ( 'NONE',  ( -0.06523048226347956391, -1.201279527559055538, 0.1574803149606297803 ) ) ;
#18916=CARTESIAN_POINT ( 'NONE',  ( -0.06523048226347956391, -1.309547243986961540, 0.1574803149606297803 ) ) ;
#18924=CARTESIAN_POINT ( 'NONE',  ( 0.09072581850463573572, 0.09340956239926197224, 0.2330524951300412539 ) ) ;
#18932=CARTESIAN_POINT ( 'NONE',  ( -0.2183122970338342572, -0.09842519685039370636, -0.1145706962327193018 ) ) ;
#18939=CARTESIAN_POINT ( 'NONE',  ( 0.1264236179284866091, -0.8469488188438739629, -0.1264236179284866091 ) ) ;
#18940=CARTESIAN_POINT ( 'NONE',  ( -0.1264236179284866091, -1.058562992072220377, 0.1264236179284866091 ) ) ;
#18944=CARTESIAN_POINT ( 'NONE',  ( -0.07444174185955065859, -0.3627406599767461493, -0.1797182628040039087 ) ) ;
#18957=CARTESIAN_POINT ( 'NONE',  ( 2.892866454678787531E-17, -0.9527559054042835651, 0.1574803149606299191 ) ) ;
#18958=CARTESIAN_POINT ( 'NONE',  ( -0.1264236179284866091, -0.2859251967966303098, -0.1264236179284866091 ) ) ;
#18960=CARTESIAN_POINT ( 'NONE',  ( 0.1264236179284866091, -1.245570866087968520, 0.1264236179284866091 ) ) ;
#18970=CARTESIAN_POINT ( 'NONE',  ( -0.07620458454312968588, -0.09842501845840670449, -0.1617485411237021276 ) ) ;
#18986=AXIS2_PLACEMENT_3D ( 'NONE', #27348, #46445, #42382 ) ;
#18990=CARTESIAN_POINT ( 'NONE',  ( -0.1787899950787401604, -1.431226330433964078, 0.07405724077823318263 ) ) ;
#18992=CARTESIAN_POINT ( 'NONE',  ( -1.094772975963752103E-17, -0.4434055117572598959, -0.1787899950787401882 ) ) ;
#18999=CARTESIAN_POINT ( 'NONE',  ( 0.1787899950787401604, -1.759842519631276581, 0.07405724077823318263 ) ) ;
#19000=CARTESIAN_POINT ( 'NONE',  ( -0.07405724077823318263, -1.700787401521039355, -0.1787899950787401604 ) ) ;
#19003=CARTESIAN_POINT ( 'NONE',  ( -0.1574803149606297803, -0.6943897637795268807, 0.06523048226347956391 ) ) ;
#19005=CARTESIAN_POINT ( 'NONE',  ( -1.100456976456230270E-17, -1.388823337142100378, -0.1797182628040039365 ) ) ;
#19013=CARTESIAN_POINT ( 'NONE',  ( -0.1574803149606299191, -0.8051181101286928321, 0.000000000000000000 ) ) ;
#19027=CARTESIAN_POINT ( 'NONE',  ( -0.1270800023317771588, -0.07484695918934468339, 0.1270800023317771588 ) ) ;
#19028=CARTESIAN_POINT ( 'NONE',  ( 0.07405724077823318263, -1.277559055064345861, -0.1787899950787401604 ) ) ;
#19037=CARTESIAN_POINT ( 'NONE',  ( -0.1787899950787401882, -0.1579724408911182820, 0.000000000000000000 ) ) ;
#19044=CARTESIAN_POINT ( 'NONE',  ( 0.1574803149606299191, 0.001968504044534917247, -1.928577636452523993E-17 ) ) ;
#19047=EDGE_CURVE ( 'NONE', #4670, #45034, #6099, .T. ) ;
#19051=CARTESIAN_POINT ( 'NONE',  ( 0.07405724077823318263, -0.9735491650796336272, -0.1787899950787401604 ) ) ;
#19055=EDGE_LOOP ( 'NONE', ( #18747, #38030, #33793, #30251, #13575, #9068 ) ) ;
#19064=CARTESIAN_POINT ( 'NONE',  ( 0.1797182628040039087, -0.9680556206066676106, 0.07444174185955046430 ) ) ;
#19072=CARTESIAN_POINT ( 'NONE',  ( -0.1113553986120547346, -0.6820866140657008136, 0.1113553986120547346 ) ) ;
#19077=CARTESIAN_POINT ( 'NONE',  ( 0.1787899950787401604, -0.6919291338045056028, 0.07405724077823318263 ) ) ;
#19084=CARTESIAN_POINT ( 'NONE',  ( -0.1113553986120547346, -1.715551181102362266, 0.1113553986120547346 ) ) ;
#19095=CARTESIAN_POINT ( 'NONE',  ( 2.892866454678787531E-17, -0.3228346455617642219, 0.1574803149606299191 ) ) ;
#19096=CARTESIAN_POINT ( 'NONE',  ( -0.1264236179284866091, -1.467027559001354398, -0.1264236179284866091 ) ) ;
#19105=CARTESIAN_POINT ( 'NONE',  ( 0.1235961452251413406, 0.09842519685039370636, -0.2140748031496062798 ) ) ;
#19107=CARTESIAN_POINT ( 'NONE',  ( 0.1264236179284866091, -0.5035688501190023203, -0.1264236179284866091 ) ) ;
#19108=CARTESIAN_POINT ( 'NONE',  ( -0.1499592427265324934, -0.08955956716458957079, -0.1972459155580799095 ) ) ;
#19119=CARTESIAN_POINT ( 'NONE',  ( -0.1787899950787401604, -1.380905511757260173, 0.07405724077823318263 ) ) ;
#19121=CARTESIAN_POINT ( 'NONE',  ( -0.07405724077823318263, -1.607283464513165949, 0.1787899950787401604 ) ) ;
#19135=CARTESIAN_POINT ( 'NONE',  ( -0.08562028147892762620, -0.08956352913554484207, 0.1336771782244998708 ) ) ;
#19138=B_SPLINE_CURVE_WITH_KNOTS ( 'NONE', 3,
 ( #15355, #14882, #12004, #26624, #4074, #8379, #18924, #19405, #18688, #22526, #25901, #15844, #33584, #1185, #11289, #44319, #37621, #37143, #30467 ),
 .UNSPECIFIED., .F., .F.,
 ( 4, 1, 1, 1, 2, 2, 1, 1, 1, 1, 2, 2, 4 ),
 ( 0.000000000000000000, 0.1249999999999984457, 0.1874999999999978351, 0.2187499999999978351, 0.2343749999999978351, 0.2499999999999978351, 0.3749999999999991673, 0.4375000000000000555, 0.4687500000000004996, 0.4843750000000006106, 0.4921875000000007216, 0.5000000000000007772, 1.000000000000000000 ),
 .UNSPECIFIED. ) ;
#19141=CARTESIAN_POINT ( 'NONE',  ( -0.08400343811428674645, 0.09129006187720335730, -0.2369336632580043012 ) ) ;
#19142=CARTESIAN_POINT ( 'NONE',  ( -9.642888182262618425E-18, -0.03740157480314960925, -0.1574803149606299191 ) ) ;
#19143=CARTESIAN_POINT ( 'NONE',  ( 0.07405724077823318263, -1.562992125930488196, 0.1787899950787401604 ) ) ;
#19144=CARTESIAN_POINT ( 'NONE',  ( -0.07405724077823318263, -0.8641732282926931630, 0.1787899950787401604 ) ) ;
#19145=CARTESIAN_POINT ( 'NONE',  ( -0.1574803149606300301, -1.250492125984252079, -0.06523048226347956391 ) ) ;
#19172=CARTESIAN_POINT ( 'NONE',  ( -0.1749533961349706845, -0.09842519685039370636, 0.1544953252376329023 ) ) ;
#19178=CARTESIAN_POINT ( 'NONE',  ( -0.1787899950787401604, -0.9133858267178897039, -0.07405724077823318263 ) ) ;
#19180=CARTESIAN_POINT ( 'NONE',  ( 0.07405724077823318263, -1.090551181048598606, 0.1787899950787401604 ) ) ;
#19183=CARTESIAN_POINT ( 'NONE',  ( 0.07444174185955046430, -0.3676619198192658255, -0.1797182628040039087 ) ) ;
#19184=CARTESIAN_POINT ( 'NONE',  ( 0.1574803149606299191, 0.1102362204724409434, -1.928577636452523993E-17 ) ) ;
#19199=CARTESIAN_POINT ( 'NONE',  ( -0.1787899950787401882, -0.4384842519147402196, 0.000000000000000000 ) ) ;
#19201=CARTESIAN_POINT ( 'NONE',  ( 0.1264236179284866091, -1.275098425143086578, -0.1264236179284866091 ) ) ;
#19209=CARTESIAN_POINT ( 'NONE',  ( -9.642888182262618425E-18, -1.208661417215307177, -0.1574803149606299191 ) ) ;
#19214=CARTESIAN_POINT ( 'NONE',  ( 0.03520570031223819313, -0.09841564447026268647, -0.1752971770356033798 ) ) ;
#19219=VERTEX_POINT ( 'NONE', #4622 ) ;
#19225=CARTESIAN_POINT ( 'NONE',  ( -0.2281991160478161473, -0.09851385135380275049, -0.09075334354666182712 ) ) ;
#19232=CARTESIAN_POINT ( 'NONE',  ( 0.07405724077823318263, -1.500123968229239768, 0.1787899950787401604 ) ) ;
#19234=CARTESIAN_POINT ( 'NONE',  ( 0.07405724077823318263, -0.3671259841982050798, -0.1787899950787401604 ) ) ;
#19236=ORIENTED_EDGE ( 'NONE', *, *, #3121, .F. ) ;
#19241=CARTESIAN_POINT ( 'NONE',  ( -0.1264236179284866091, -1.781988188922614347, -0.1264236179284866091 ) ) ;
#19242=CARTESIAN_POINT ( 'NONE',  ( -0.1264236179284866091, -1.619586614119464585, -0.1264236179284866091 ) ) ;
#19248=CARTESIAN_POINT ( 'NONE',  ( 0.06523048226347956391, -0.7091535433070863537, -0.1574803149606300301 ) ) ;
#19250=CARTESIAN_POINT ( 'NONE',  ( 0.1797182628040039087, -1.435575305646038524, -0.07444174185955065859 ) ) ;
#19270=CARTESIAN_POINT ( 'NONE',  ( 0.1574803149606300301, -0.04478346456692917921, -0.06523048226347956391 ) ) ;
#19272=CARTESIAN_POINT ( 'NONE',  ( -0.07444174185955065859, -0.04778003005548651927, -0.1797182628040039087 ) ) ;
#19273=CARTESIAN_POINT ( 'NONE',  ( 0.1787899950787401604, -1.243110236166709459, -0.07405724077823318263 ) ) ;
#19274=CARTESIAN_POINT ( 'NONE',  ( 0.000000000000000000, -0.09842519685039370636, 0.1574803149606299191 ) ) ;
#19282=ORIENTED_EDGE ( 'NONE', *, *, #18617, .T. ) ;
#19288=CARTESIAN_POINT ( 'NONE',  ( 0.06523048226347956391, -0.03001968493184305545, -0.1574803149606300301 ) ) ;
#19294=CARTESIAN_POINT ( 'NONE',  ( -1.094772975963752103E-17, -1.010458613898529645, -0.1787899950787401882 ) ) ;
#19296=CARTESIAN_POINT ( 'NONE',  ( 0.07405724077823318263, 0.06594488194352733645, -0.1787899950787401604 ) ) ;
#19297=EDGE_LOOP ( 'NONE', ( #25180, #33063, #38797 ) ) ;
#19304=CARTESIAN_POINT ( 'NONE',  ( 0.07405724077823318263, -0.5049212597887556830, 0.1787899950787401604 ) ) ;
#19310=CARTESIAN_POINT ( 'NONE',  ( -1.100456976456230270E-17, -0.9951225497405256082, -0.1797182628040039365 ) ) ;
#19319=CARTESIAN_POINT ( 'NONE',  ( 2.892866454678787531E-17, -0.05708661417322834220, 0.1574803149606299191 ) ) ;
#19321=CARTESIAN_POINT ( 'NONE',  ( 0.1574803149606300301, -0.6648622046168815025, -0.06523048226347956391 ) ) ;
#19327=CARTESIAN_POINT ( 'NONE',  ( -1.094772975963752103E-17, -0.7977362204186770889, -0.1787899950787401882 ) ) ;
#19330=CARTESIAN_POINT ( 'NONE',  ( 2.892866454678787531E-17, -1.464566929026330788, 0.1574803149606299191 ) ) ;
#19334=CARTESIAN_POINT ( 'NONE',  ( 0.06523048226347956391, -1.668799212598424342, 0.1574803149606297803 ) ) ;
#19340=CARTESIAN_POINT ( 'NONE',  ( -0.07405724077823318263, -1.469488188922614791, -0.1787899950787401604 ) ) ;
#19346=CARTESIAN_POINT ( 'NONE',  ( 0.1787899950787401604, -0.5060294800402627136, -0.07405724077823318263 ) ) ;
#19347=CARTESIAN_POINT ( 'NONE',  ( -0.1687763848766232477, -0.08955970710929901657, 0.1556180494977049134 ) ) ;
#19348=CARTESIAN_POINT ( 'NONE',  ( 2.892866454678787531E-17, 0.03149606309965303358, 0.1574803149606299191 ) ) ;
#19351=CARTESIAN_POINT ( 'NONE',  ( 0.1264236179284866091, -1.812623968229240212, 0.1264236179284866091 ) ) ;
#19354=CARTESIAN_POINT ( 'NONE',  ( 0.2471922899045338740, -0.07845124750586851547, 0.07638293795143560883 ) ) ;
#19357=CARTESIAN_POINT ( 'NONE',  ( 0.07405724077823318263, -1.292322834591905778, 0.1787899950787401604 ) ) ;
#19358=CARTESIAN_POINT ( 'NONE',  ( 0.07405724077823318263, -1.562992125930488196, 0.1787899950787401604 ) ) ;
#19367=CARTESIAN_POINT ( 'NONE',  ( -0.06523048226347956391, -0.3351377952755906775, 0.1574803149606297803 ) ) ;
#19377=CARTESIAN_POINT ( 'NONE',  ( -0.1686160743781814630, -0.08918665060197839001, 0.1880811715468738432 ) ) ;
#19380=CARTESIAN_POINT ( 'NONE',  ( -0.1062059389003459364, -0.08956135442286349002, 0.1200209881557332131 ) ) ;
#19388=CARTESIAN_POINT ( 'NONE',  ( 0.07405724077823318263, -1.705708661363559253, -0.1787899950787401604 ) ) ;
#19389=CARTESIAN_POINT ( 'NONE',  ( 0.06523048226347956391, -1.014271653435780296, -0.1574803149606300301 ) ) ;
#19390=CARTESIAN_POINT ( 'NONE',  ( 0.1264236179284866091, -0.8863188975840314843, -0.1264236179284866091 ) ) ;
#19391=CARTESIAN_POINT ( 'NONE',  ( -0.1113553986120547346, -1.243110236220472453, 0.1113553986120547346 ) ) ;
#19405=CARTESIAN_POINT ( 'NONE',  ( 0.08994717584591196968, 0.09317026862873967197, 0.2335020446786578718 ) ) ;
#19412=CARTESIAN_POINT ( 'NONE',  ( -0.09071607244976082063, -0.09842519685039370636, -0.2375934515383263668 ) ) ;
#19419=CARTESIAN_POINT ( 'NONE',  ( -0.1787899950787401604, -0.8346456692375755493, -0.07405724077823318263 ) ) ;
#19420=CARTESIAN_POINT ( 'NONE',  ( -0.1264236179284866091, -1.097933070812378009, 0.1264236179284866091 ) ) ;
#19421=ADVANCED_FACE ( 'NONE', ( #34365 ), #41325, .F. ) ;
#19424=CARTESIAN_POINT ( 'NONE',  ( -1.100456976456230270E-17, -0.3652012898980063205, -0.1797182628040039365 ) ) ;
#19437=CARTESIAN_POINT ( 'NONE',  ( 0.1264236179284866091, -0.4237204723871811352, 0.1264236179284866091 ) ) ;
#19439=CARTESIAN_POINT ( 'NONE',  ( -1.094772975963752103E-17, -1.191437007820251859, -0.1787899950787401882 ) ) ;
#19448=CARTESIAN_POINT ( 'NONE',  ( 0.03096532509380343218, -0.09840740886148355293, -0.1761182458273901907 ) ) ;
#19466=CARTESIAN_POINT ( 'NONE',  ( -0.07405724077823318263, -1.426305070591442625, 0.1787899950787401604 ) ) ;
#19468=ORIENTED_EDGE ( 'NONE', *, *, #42296, .F. ) ;
#19470=CARTESIAN_POINT ( 'NONE',  ( 0.07405724077823318263, -0.4606299212060784853, 0.1787899950787401604 ) ) ;
#19478=CARTESIAN_POINT ( 'NONE',  ( -1.094772975963752103E-17, -1.786909448765134023, -0.1787899950787401882 ) ) ;
#19480=CARTESIAN_POINT ( 'NONE',  ( 0.1773397566031712225, -0.09842519685039370636, 0.01193638218527439190 ) ) ;
#19486=CARTESIAN_POINT ( 'NONE',  ( -0.06523048226347956391, -0.7436023622047251980, -0.1574803149606300301 ) ) ;
#19488=CARTESIAN_POINT ( 'NONE',  ( 0.1797182628040039365, -1.556146171787769594, -2.200913952912460540E-17 ) ) ;
#19490=CARTESIAN_POINT ( 'NONE',  ( 0.06523048226347956391, -0.4630905510735751074, -0.1574803149606300301 ) ) ;
#19501=CARTESIAN_POINT ( 'NONE',  ( -1.094772975963752103E-17, 0.02411417328210995956, -0.1787899950787401882 ) ) ;
#19510=CARTESIAN_POINT ( 'NONE',  ( -0.07444174185955065859, -0.03301625052792742793, 0.1797182628040039087 ) ) ;
#19511=CARTESIAN_POINT ( 'NONE',  ( -1.094772975963752103E-17, -1.156988188922614125, -0.1787899950787401882 ) ) ;
#19521=CARTESIAN_POINT ( 'NONE',  ( -0.1178667752584066641, -0.09842519685039365085, -0.2173826564421876550 ) ) ;
#19524=CARTESIAN_POINT ( 'NONE',  ( 0.1574803149606299191, -0.07677165343578011558, -1.928577636452523993E-17 ) ) ;
#19529=LINE ( 'NONE', #34399, #35631 ) ;
#19531=DIRECTION ( 'NONE',  ( 0.000000000000000000, 0.000000000000000000, 1.000000000000000000 ) ) ;
#19532=CARTESIAN_POINT ( 'NONE',  ( -0.1787899950787401604, -0.9194153068119157446, 0.07405724077823318263 ) ) ;
#19534=CARTESIAN_POINT ( 'NONE',  ( 0.1787899950787401604, 0.06102362210100767403, -0.07405724077823318263 ) ) ;
#19543=CARTESIAN_POINT ( 'NONE',  ( -0.07405724077823318263, -0.6279527558517482566, 0.1787899950787401604 ) ) ;
#19548=CARTESIAN_POINT ( 'NONE',  ( -0.1797182628040039087, -1.027110738716904725, -0.07444174185955065859 ) ) ;
#19557=CARTESIAN_POINT ( 'NONE',  ( -0.07405724077823318263, 0.1102362205262043815, -0.1787899950787401604 ) ) ;
#19563=CARTESIAN_POINT ( 'NONE',  ( -0.1787899950787401604, -0.9872047243556864027, -0.07405724077823318263 ) ) ;
#19569=CARTESIAN_POINT ( 'NONE',  ( 0.1113553986120547346, -1.617125984144440753, 0.1113553986120547346 ) ) ;
#19575=CARTESIAN_POINT ( 'NONE',  ( -0.1113553986120547346, -1.764763779527559029, -0.1113553986120547346 ) ) ;
#19580=CARTESIAN_POINT ( 'NONE',  ( 3.284318927891251994E-17, -1.570374015694267600, 0.1787899950787401882 ) ) ;
#19582=EDGE_CURVE ( 'NONE', #802, #6080, #39054, .T. ) ;
#19589=CARTESIAN_POINT ( 'NONE',  ( 0.1264236179284866091, -0.6315216060245139040, 0.1264236179284866091 ) ) ;
#19590=CARTESIAN_POINT ( 'NONE',  ( -0.03820435495970567197, -0.08955995172511357905, 0.2191518663821425128 ) ) ;
#19591=CARTESIAN_POINT ( 'NONE',  ( 0.1113553986120547346, 0.03641732294217271682, 0.1113553986120547346 ) ) ;
#19593=EDGE_CURVE ( 'NONE', #11736, #38566, #18412, .T. ) ;
#19597=CARTESIAN_POINT ( 'NONE',  ( -0.07405724077823318263, -1.795399558780420124, -0.1787899950787401604 ) ) ;
#19600=CARTESIAN_POINT ( 'NONE',  ( 3.284318927891251994E-17, -1.412893700733637958, 0.1787899950787401882 ) ) ;
#19601=CARTESIAN_POINT ( 'NONE',  ( -1.094772975963752103E-17, -1.585137795221826629, -0.1787899950787401882 ) ) ;
#19609=CARTESIAN_POINT ( 'NONE',  ( 0.06523048226347956391, -0.4089566929133856554, 0.1574803149606297803 ) ) ;
#19615=CARTESIAN_POINT ( 'NONE',  ( -0.06523048226347956391, -0.5615157479239690774, 0.1574803149606297803 ) ) ;
#19618=CARTESIAN_POINT ( 'NONE',  ( -0.1348413527256734357, -0.08956084189530488793, 0.09142978980987383208 ) ) ;
#19619=CARTESIAN_POINT ( 'NONE',  ( -0.1264236179284866091, -0.4778543306548976854, -0.1264236179284866091 ) ) ;
#19627=CARTESIAN_POINT ( 'NONE',  ( -0.1787899950787401604, -0.9084645668753701386, 0.07405724077823318263 ) ) ;
#19628=CARTESIAN_POINT ( 'NONE',  ( -0.06523048226347956391, -1.255413385826771533, -0.1574803149606300301 ) ) ;
#19637=CARTESIAN_POINT ( 'NONE',  ( -0.1574803149606297803, -1.393208661309796925, 0.06523048226347956391 ) ) ;
#19653=CARTESIAN_POINT ( 'NONE',  ( 0.04598081178002756675, -0.09851382463604664574, 0.1460396181123653492 ) ) ;
#19659=CARTESIAN_POINT ( 'NONE',  ( -0.1787899950787401882, -0.9502952755367874982, 0.000000000000000000 ) ) ;
#19660=CARTESIAN_POINT ( 'NONE',  ( 3.284318927891251994E-17, -1.053641732229700700, 0.1787899950787401882 ) ) ;
#19664=CARTESIAN_POINT ( 'NONE',  ( 0.1270800023317771588, -0.4094926284806834071, -0.1270800023317771588 ) ) ;
#19665=CARTESIAN_POINT ( 'NONE',  ( 0.1574803149606299191, -1.809055118002708795, -1.928577636452523993E-17 ) ) ;
#19666=CARTESIAN_POINT ( 'NONE',  ( 2.892866454678787531E-17, 0.1003937007874015908, 0.1574803149606299191 ) ) ;
#19667=CARTESIAN_POINT ( 'NONE',  ( 0.1787899950787401882, -0.1825787401037169411, -2.189545951927503898E-17 ) ) ;
#19674=CARTESIAN_POINT ( 'NONE',  ( 0.1787899950787401882, -0.4581692912848189247, -2.189545951927503898E-17 ) ) ;
#19676=CARTESIAN_POINT ( 'NONE',  ( -0.1264236179284866091, -1.186515747977732183, -0.1264236179284866091 ) ) ;
#19685=CARTESIAN_POINT ( 'NONE',  ( 0.07255072011368295104, -0.09842519689660865490, -0.1635392243539251500 ) ) ;
#19690=EDGE_CURVE ( 'NONE', #6678, #30877, #9804, .T. ) ;
#19693=B_SPLINE_SURFACE_WITH_KNOTS ( 'NONE', 1, 3, ( 
 ( #15658, #41716, #8918, #15895, #23546, #528, #15416, #1240, #26444, #30067, #44604, #8200, #11820, #22823, #19225, #30297, #24484, #30984, #20164, #9872, #17051, #45551, #19928, #42197, #1959, #41949, #16363, #27406, #28096, #12771, #20874, #24018, #9403, #45794, #24715, #9155, #2190, #34564, #13243, #23772, #6249, #13467, #1716, #39077, #2657, #17288, #13000, #38620, #31693, #38382, #35043, #35516, #39315, #31923, #5555, #16592, #34817, #5797, #20403, #31217, #27643, #24255, #46507, #16812, #42658, #31450, #13688, #46034, #27871, #42430, #9637, #28324, #38852, #46273, #6017, #2421, #42893, #20639, #10103, #35284, #18236, #3849, #25193, #29066, #39555, #32880, #43624, #36462, #33121, #40257, #21108, #21595, #3133, #28822, #44102, #10595, #2882, #3619, #2524, #10348, #29551, #39779, #35747, #40021, #43865, #6728, #14646, #17518, #29318, #14179, #25685, #32155, #28577, #6971, #46743, #25446, #32647, #24957, #21346, #47232, #46985, #7215, #21839, #37628, #22293, #8147, #30473, #12492, #8625, #29777, #37151, #36928, #44558, #26394, #4080, #4299, #44797, #23262, #33357, #1191, #11776, #19653, #7676, #15132, #40719, #15362, #45029, #44326, #4786, #11529 ),
 ( #19412, #37878, #40957, #949, #26149, #34062, #15608, #23015, #5031, #26867, #45272, #22771, #18932, #30012, #30706, #37380, #18696, #15850, #12244, #7918, #41428, #4535, #40489, #26631, #34297, #22533, #1422, #16081, #478, #704, #33591, #19172, #33829, #30246, #12010, #41183, #8386, #9589, #2370, #45747, #19887, #42145, #12955, #30944, #27595, #9826, #6199, #45505, #9353, #13420, #39031, #24210, #17005, #28052, #20823, #42391, #20122, #35462, #31874, #34769, #24431, #38577, #45987, #16770, #31644, #38105, #27359, #46220, #38810, #5269, #27118, #1911, #9111, #1668, #23503, #34515, #35236, #16316, #42612, #31174, #16547, #5508, #46453, #12729, #23974, #41665, #20360, #41902, #2606, #20589, #8870, #17238, #23731, #38335, #5746, #34999, #2144, #31411, #13195, #27831, #5970, #40198, #43333, #29261, #6439, #32351, #32820, #14121, #11005, #14359, #28763, #22005, #32587, #13876, #18179, #25132, #32098, #28518, #18410, #33059, #25623, #24903, #6908, #47176, #47413, #28275, #39722, #14587, #39499, #21531, #43564, #36168, #3322, #17935, #29007, #10049, #10776, #7395, #25387, #36630, #39964, #7156, #36408, #4467, #26082, #22472, #419, #44493, #41359, #29493 ),
 ( #7854, #44966, #11710, #19108, #37318, #4723, #11238, #15071, #37563, #44733, #25849, #14826, #37090, #29718, #22229, #44037, #7613, #8322, #40431, #1129, #4238, #18868, #40657, #4963, #36862, #29948, #4017, #40896, #18636, #15788, #41125, #33296, #19347, #30417, #12177, #33527, #15296, #11949, #44264, #26335, #26801, #19590, #8562, #11464, #8089, #22712, #33773, #884, #15544, #30188, #26570, #23196, #22953, #37810, #5441, #13361, #1365, #8800, #34452, #9045, #38754, #23433, #31340, #38041, #16711, #45923, #30884, #13138, #9527, #27773, #1598, #20533, #16483, #2312, #16252, #20058, #5198, #27989, #31113, #16942, #27047, #41840, #35168, #34701, #31582, #34937, #38274, #42556, #20294, #45444, #46165, #1845, #19824, #45203, #38971, #6136, #9762, #12666, #27530, #2083, #24151, #34234, #45678, #24373, #27291, #23666, #42332, #12895, #42082, #9287, #23907, #16019, #30642, #12427, #38513, #41595, #39911, #39202, #35408, #25076, #46633, #43028, #20990, #17647, #14537, #2547, #6379, #13576, #21469, #17884, #10954, #6622, #35861, #32529, #28214, #28704, #17403, #47114, #7099, #36357, #28949, #14306, #43277, #43510, #21235, #6851, #13817, #9993, #3013, #24603 ) ),
 .UNSPECIFIED., .F., .F., .F.,
 ( 2, 1, 2 ),
 ( 4, 2, 2, 2, 2, 2, 2, 2, 2, 2, 2, 2, 2, 2, 2, 2, 2, 2, 2, 2, 2, 2, 2, 2, 2, 2, 2, 2, 2, 2, 2, 2, 2, 2, 2, 2, 2, 2, 2, 2, 2, 2, 2, 2, 2, 2, 2, 2, 2, 2, 2, 2, 2, 2, 2, 2, 2, 2, 2, 2, 2, 2, 2, 2, 2, 2, 2, 2, 2, 2, 2, 2, 2, 2, 4 ),
 ( -0.01000000000000000021, 0.000000000000000000, 1.000000000000000000 ),
 ( 0.001590707300269399854, 0.003174300033026545165, 0.003966096399405114568, 0.004757892765783690477, 0.005549689132162260313, 0.005945587315351550002, 0.006341485498540830150, 0.007133281864919399987, 0.007925078231297981099, 0.009508670964055120772, 0.01030046733043370015, 0.01109226369681226045, 0.01188406006319083982, 0.01227995824638011997, 0.01267585642956940012, 0.01346765279594797950, 0.01386355097913725964, 0.01425944916232653979, 0.01584304189508370028, 0.01663483826146225017, 0.01742663462784084863, 0.01782253281103009929, 0.01821843099421939852, 0.01901022736059800045, 0.01980202372697655033, 0.02019792191016584956, 0.02059382009335514879, 0.02138561645973369868, 0.02178151464292299791, 0.02217741282611225204, 0.02376100555886940038, 0.02455280192524800231, 0.02534459829162654873, 0.02613639465800515066, 0.02692819102438370055, 0.02732408920757299978, 0.02771998739076224696, 0.02851178375714085236, 0.02930358012351940225, 0.03009537648989799724, 0.03088717285627655060, 0.03128307103946584983, 0.03167896922265514559, 0.03247076558903369548, 0.03326256195541230087, 0.03405435832179084382, 0.03484615468816940065, 0.03563795105454799911, 0.03603384923773730181, 0.03642974742092654900, 0.03722154378730514745, 0.03801334015368370428, 0.03880513652006229580, 0.03959693288644084569, 0.03999283106963014839, 0.04038872925281945109, 0.04118052561919799404, 0.04197232198557655086, 0.04276411835195514932, 0.04355591471833369921, 0.04395181290152299497, 0.04434771108471229767, 0.04513950745109090307, 0.04553540563428010168, 0.04593130381746940438, 0.04672310018384799590, 0.04751489655022660130, 0.04830669291660510262, 0.04870259109979440532, 0.04909848928298370108, 0.04989028564936229954, 0.05068208201574090493, 0.05107798019893020069, 0.05147387838211939931, 0.05226567474849799777 ),
 .UNSPECIFIED. ) ;
#19703=B_SPLINE_CURVE_WITH_KNOTS ( 'NONE', 3,
 ( #4612, #4857, #19480, #27184, #34132, #37946, #5095, #19718, #45346, #8940, #23563, #39331, #35303, #9425, #31709, #2440, #20427, #17069, #46764, #43161, #35061, #42453, #6268 ),
 .UNSPECIFIED., .F., .F.,
 ( 4, 2, 2, 2, 2, 2, 2, 1, 2, 2, 2, 4 ),
 ( 0.000000000000000000, 0.001005003112249313116, 0.002010006224498626232, 0.002512507780623283223, 0.003015009336747939347, 0.004020012448997250729, 0.004522514005121907286, 0.005025015561246563844, 0.005527517117371220402, 0.006030018673495876093, 0.007035021785745188341, 0.008040024897994499722 ),
 .UNSPECIFIED. ) ;
#19705=CARTESIAN_POINT ( 'NONE',  ( -0.07405724077823318263, -1.519809007599318695, -0.1787899950787401604 ) ) ;
#19708=CARTESIAN_POINT ( 'NONE',  ( -0.07405724077823318263, -0.3868110235682837295, 0.1787899950787401604 ) ) ;
#19716=CARTESIAN_POINT ( 'NONE',  ( 0.1264236179284866091, -1.762303149552535642, 0.1264236179284866091 ) ) ;
#19718=CARTESIAN_POINT ( 'NONE',  ( 0.1495489095487642639, -0.09842519685039370636, 0.08573672929712505830 ) ) ;
#19721=CARTESIAN_POINT ( 'NONE',  ( 0.1574803149606299191, -0.7952755905511811330, -1.928577636452523993E-17 ) ) ;
#19723=CARTESIAN_POINT ( 'NONE',  ( -1.100456976456230270E-17, -1.625043809583045284, -0.1797182628040039365 ) ) ;
#19734=CARTESIAN_POINT ( 'NONE',  ( 3.284318927891251994E-17, 0.04379921265218874454, 0.1787899950787401882 ) ) ;
#19744=CARTESIAN_POINT ( 'NONE',  ( 0.06523048226347956391, -0.03986220472440944740, -0.1574803149606300301 ) ) ;
#19746=CARTESIAN_POINT ( 'NONE',  ( 0.1113553986120547346, -1.095472440837354400, -0.1113553986120547346 ) ) ;
#19764=CARTESIAN_POINT ( 'NONE',  ( 0.1113553986120547346, -0.07185039359326043928, -0.1113553986120547346 ) ) ;
#19770=CARTESIAN_POINT ( 'NONE',  ( -0.1264236179284866091, -1.035064913111127805, 0.1264236179284866091 ) ) ;
#19772=CARTESIAN_POINT ( 'NONE',  ( 0.07405724077823318263, -0.02755905506434671789, 0.1787899950787401604 ) ) ;
#19775=FACE_OUTER_BOUND ( 'NONE', #19055, .T. ) ;
#19778=CARTESIAN_POINT ( 'NONE',  ( -0.07405724077823318263, -0.6427165353793066194, -0.1787899950787401604 ) ) ;
#19781=CARTESIAN_POINT ( 'NONE',  ( 0.1270800023317771588, -1.127996565488557090, 0.1270800023317771588 ) ) ;
#19789=CARTESIAN_POINT ( 'NONE',  ( 0.1113553986120547346, -0.7411417321759370402, -0.1113553986120547346 ) ) ;
#19790=CARTESIAN_POINT ( 'NONE',  ( -0.1264236179284866091, 0.1225393701325037388, 0.1264236179284866091 ) ) ;
#19799=CARTESIAN_POINT ( 'NONE',  ( -0.1113553986120547346, -1.636811023514519681, -0.1113553986120547346 ) ) ;
#19801=DIRECTION ( 'NONE',  ( 0.000000000000000000, 1.000000000000000000, 0.000000000000000000 ) ) ;
#19804=CARTESIAN_POINT ( 'NONE',  ( 0.09932472909918407811, -0.09575019180979010835, 0.2280862973329967069 ) ) ;
#19805=CARTESIAN_POINT ( 'NONE',  ( -0.1264236179284866091, 0.1126968504474643862, -0.1264236179284866091 ) ) ;
#19810=CARTESIAN_POINT ( 'NONE',  ( -0.05275482926409180012, 0.07559918600399900823, 0.2549750559894655155 ) ) ;
#19814=CARTESIAN_POINT ( 'NONE',  ( -0.07405724077823318263, -1.508858267662772867, -0.1787899950787401604 ) ) ;
#19823=CARTESIAN_POINT ( 'NONE',  ( 0.1787899950787401604, -0.5503208186229400223, 0.07405724077823318263 ) ) ;
#19824=CARTESIAN_POINT ( 'NONE',  ( 0.02124828133781109935, -0.08956063275447755101, -0.1867302004102397717 ) ) ;
#19828=CARTESIAN_POINT ( 'NONE',  ( 0.1264236179284866091, -1.802781448544200860, -0.1264236179284866091 ) ) ;
#19832=CARTESIAN_POINT ( 'NONE',  ( 0.1787899950787401604, -1.523622047190330564, 0.07405724077823318263 ) ) ;
#19839=CARTESIAN_POINT ( 'NONE',  ( 0.1270800023317771588, -0.7342957780869823203, 0.1270800023317771588 ) ) ;
#19843=CARTESIAN_POINT ( 'NONE',  ( -0.06523048226347956391, -0.3745078740157483099, 0.1574803149606297803 ) ) ;
#19857=CARTESIAN_POINT ( 'NONE',  ( 0.1787899950787401604, -0.6082677164816695514, -0.07405724077823318263 ) ) ;
#19858=CARTESIAN_POINT ( 'NONE',  ( 2.892866454678787531E-17, -0.04724409438066189126, 0.1574803149606299191 ) ) ;
#19866=CARTESIAN_POINT ( 'NONE',  ( -1.094772975963752103E-17, -1.742618110182456714, -0.1787899950787401882 ) ) ;
#19867=CARTESIAN_POINT ( 'NONE',  ( -0.1264236179284866091, -0.8371062991588346103, -0.1264236179284866091 ) ) ;
#19868=CARTESIAN_POINT ( 'NONE',  ( 0.06523048226347956391, -1.417814960629922627, -0.1574803149606300301 ) ) ;
#19875=CARTESIAN_POINT ( 'NONE',  ( 0.1113553986120547346, 0.006889763887054606122, -0.1113553986120547346 ) ) ;
#19883=CARTESIAN_POINT ( 'NONE',  ( -0.1235961452251413406, 0.09842519685039370636, 0.2140748031496062798 ) ) ;
#19887=CARTESIAN_POINT ( 'NONE',  ( -0.05397493303295378131, -0.09842519685039370636, 0.2204705300331200601 ) ) ;
#19891=CARTESIAN_POINT ( 'NONE',  ( 0.1264236179284866091, -1.014271653489543290, 0.1264236179284866091 ) ) ;
#19892=CARTESIAN_POINT ( 'NONE',  ( 0.1787899950787401604, -1.080708661363559919, -0.07405724077823318263 ) ) ;
#19895=CARTESIAN_POINT ( 'NONE',  ( 3.301370929368692659E-17, -0.4242564080082424915, 0.1797182628040039365 ) ) ;
#19896=CARTESIAN_POINT ( 'NONE',  ( 0.06523048226347956391, -1.777066929026330344, 0.1574803149606297803 ) ) ;
#19898=CARTESIAN_POINT ( 'NONE',  ( -0.1574803149606300301, -0.03001968503937006705, -0.06523048226347956391 ) ) ;
#19899=CARTESIAN_POINT ( 'NONE',  ( -0.07405724077823318263, -0.1309055117572600901, -0.1787899950787401604 ) ) ;
#19900=EDGE_CURVE ( 'NONE', #38566, #35894, #24650, .T. ) ;
#19910=CARTESIAN_POINT ( 'NONE',  ( 0.1787899950787401604, -0.4212598424659216856, 0.07405724077823318263 ) ) ;
#19912=CARTESIAN_POINT ( 'NONE',  ( -0.07405724077823318263, -1.331692913332063855, 0.1787899950787401604 ) ) ;
#19920=CARTESIAN_POINT ( 'NONE',  ( 0.08391120367376535272, -0.09842556176169890703, -0.1578933197585290493 ) ) ;
#19924=CARTESIAN_POINT ( 'NONE',  ( -0.05636151600970552150, -0.07780576619187905274, 0.2528927375204715888 ) ) ;
#19928=CARTESIAN_POINT ( 'NONE',  ( -0.2304365790506456846, -0.09851385065409645758, 0.06211564517574902355 ) ) ;
#19934=CARTESIAN_POINT ( 'NONE',  ( 0.1787899950787401882, -1.610852314685931264, -2.189545951927503898E-17 ) ) ;
#19937=CARTESIAN_POINT ( 'NONE',  ( 0.1264236179284866091, -0.6156496062454488438, 0.1264236179284866091 ) ) ;
#19946=CARTESIAN_POINT ( 'NONE',  ( 0.1264236179284866091, 0.1165098900384777536, 0.1264236179284866091 ) ) ;
#19947=CARTESIAN_POINT ( 'NONE',  ( -0.1264236179284866091, -1.806594488135212728, 0.1264236179284866091 ) ) ;
#19952=CARTESIAN_POINT ( 'NONE',  ( -0.1113553986120547346, -0.7805118110236219930, -0.1113553986120547346 ) ) ;
#19954=CARTESIAN_POINT ( 'NONE',  ( -0.1270800023317771588, -1.649650108795643666, 0.1270800023317771588 ) ) ;
#19956=CARTESIAN_POINT ( 'NONE',  ( -0.06523048226347956391, -0.04970472430192177798, 0.1574803149606297803 ) ) ;
#19957=CARTESIAN_POINT ( 'NONE',  ( 0.1113553986120547346, -0.4655511809948346680, -0.1113553986120547346 ) ) ;
#19958=CARTESIAN_POINT ( 'NONE',  ( 0.1787899950787401604, -0.4114173227808823330, -0.07405724077823318263 ) ) ;
#19965=EDGE_CURVE ( 'NONE', #3128, #39269, #10985, .T. ) ;
#19968=CARTESIAN_POINT ( 'NONE',  ( 0.07405724077823318263, 0.02165354336085014916, -0.1787899950787401604 ) ) ;
#19979=CARTESIAN_POINT ( 'NONE',  ( 0.1264236179284866091, -1.329232283410803239, 0.1264236179284866091 ) ) ;
#19995=CARTESIAN_POINT ( 'NONE',  ( 2.892866454678787531E-17, -0.04724409438066189126, 0.1574803149606299191 ) ) ;
#20001=CARTESIAN_POINT ( 'NONE',  ( 0.1787899950787401882, -1.217151527284356272, -2.189545951927503898E-17 ) ) ;
#20003=CARTESIAN_POINT ( 'NONE',  ( -0.1264236179284866091, 0.07332677170730689253, -0.1264236179284866091 ) ) ;
#20009=AXIS2_PLACEMENT_3D ( 'NONE', #21336, #38613, #46265 ) ;
#20010=CARTESIAN_POINT ( 'NONE',  ( -0.1787899950787401604, -0.6377952755367874982, -0.07405724077823318263 ) ) ;
#20016=CARTESIAN_POINT ( 'NONE',  ( 0.1797182628040039087, -1.199354833205092730, -0.07444174185955065859 ) ) ;
#20017=CARTESIAN_POINT ( 'NONE',  ( 0.1641447577951997139, 0.1299212598425197596, -0.05120236303050382243 ) ) ;
#20026=CARTESIAN_POINT ( 'NONE',  ( 0.1787899950787401604, 0.05610236225848785896, 0.07405724077823318263 ) ) ;
#20034=CARTESIAN_POINT ( 'NONE',  ( -0.1574803149606299191, -1.749999999892472458, 0.000000000000000000 ) ) ;
#20036=CARTESIAN_POINT ( 'NONE',  ( -0.1787899950787401604, -0.08169291333206318839, -0.07405724077823318263 ) ) ;
#20042=CARTESIAN_POINT ( 'NONE',  ( -0.1574803149606300301, -1.762303149606299968, -0.06523048226347956391 ) ) ;
#20048=CARTESIAN_POINT ( 'NONE',  ( -0.1787899950787401604, -1.538385826717890703, 0.07405724077823318263 ) ) ;
#20055=CARTESIAN_POINT ( 'NONE',  ( 0.1459804379636932548, 0.1272537536561319516, -0.07636242287093111814 ) ) ;
#20057=CARTESIAN_POINT ( 'NONE',  ( -0.1787899950787401882, -0.5675452280717583342, 0.000000000000000000 ) ) ;
#20058=CARTESIAN_POINT ( 'NONE',  ( 0.1913537776491429088, -0.08956048629241221415, -0.05990061976413484091 ) ) ;
#20070=CARTESIAN_POINT ( 'NONE',  ( 0.1787899950787401882, -1.481791338528913426, -2.189545951927503898E-17 ) ) ;
#20078=CARTESIAN_POINT ( 'NONE',  ( 0.1574803149606299191, -0.4409448818897637734, -1.928577636452523993E-17 ) ) ;
#20081=CARTESIAN_POINT ( 'NONE',  ( 0.000000000000000000, 0.1299212598425196763, 0.000000000000000000 ) ) ;
#20088=CARTESIAN_POINT ( 'NONE',  ( 0.1235961452251413406, 0.09842519685039370636, -0.2140748031496062798 ) ) ;
#20093=CARTESIAN_POINT ( 'NONE',  ( 3.284318927891251994E-17, -0.5418307086076535883, 0.1787899950787401882 ) ) ;
#20100=CARTESIAN_POINT ( 'NONE',  ( -0.1787899950787401604, -1.695866141678520567, -0.07405724077823318263 ) ) ;
#20101=CARTESIAN_POINT ( 'NONE',  ( -0.1787899950787401604, -0.9527559054580476694, -0.07405724077823318263 ) ) ;
#20102=CARTESIAN_POINT ( 'NONE',  ( 2.892866454678787531E-17, -1.435039370078740273, 0.1574803149606299191 ) ) ;
#20114=FACE_OUTER_BOUND ( 'NONE', #41454, .T. ) ;
#20117=CARTESIAN_POINT ( 'NONE',  ( -0.1854001451104914655, 0.08095196624128615792, 0.1783922471788038089 ) ) ;
#20122=CARTESIAN_POINT ( 'NONE',  ( 0.1141172636152937014, -0.09842519685039370636, 0.1860162816150570941 ) ) ;
#20131=ADVANCED_FACE ( 'NONE', ( #26062 ), #8538, .T. ) ;
#20132=CARTESIAN_POINT ( 'NONE',  ( -1.094772975963752103E-17, -1.078248031442299304, -0.1787899950787401882 ) ) ;
#20133=CARTESIAN_POINT ( 'NONE',  ( 0.1264236179284866091, -1.206200787347811110, 0.1264236179284866091 ) ) ;
#20135=CARTESIAN_POINT ( 'NONE',  ( 0.1797182628040039365, -0.5325241245436755921, -2.200913952912460540E-17 ) ) ;
#20137=CARTESIAN_POINT ( 'NONE',  ( -0.1113553986120547346, 0.006889763779527558960, -0.1113553986120547346 ) ) ;
#20138=CARTESIAN_POINT ( 'NONE',  ( -0.1264236179284866091, -0.1678149605761578844, -0.1264236179284866091 ) ) ;
#20146=CARTESIAN_POINT ( 'NONE',  ( 0.1787899950787401604, -0.4606299212060784853, 0.07405724077823318263 ) ) ;
#20148=CARTESIAN_POINT ( 'NONE',  ( -0.1264236179284866091, -1.462106299158834721, -0.1264236179284866091 ) ) ;
#20157=CARTESIAN_POINT ( 'NONE',  ( 0.1159354540250667615, -0.09844533245960994383, -0.1362465444070161402 ) ) ;
#20164=CARTESIAN_POINT ( 'NONE',  ( -0.2423783858011515635, -0.09851385377439449142, -0.009343542218490177159 ) ) ;
#20166=ADVANCED_FACE ( 'NONE', ( #399 ), #3104, .T. ) ;
#20171=CARTESIAN_POINT ( 'NONE',  ( 3.284318927891251994E-17, -1.541954676890655573, 0.1787899950787401882 ) ) ;
#20174=CARTESIAN_POINT ( 'NONE',  ( -1.094772975963752103E-17, -0.6402559054580471143, -0.1787899950787401882 ) ) ;
#20182=CARTESIAN_POINT ( 'NONE',  ( -0.1264236179284866091, -0.8223425196312754704, 0.1264236179284866091 ) ) ;
#20185=CARTESIAN_POINT ( 'NONE',  ( -0.1787899950787401882, -0.05573420444971117355, 0.000000000000000000 ) ) ;
#20189=CARTESIAN_POINT ( 'NONE',  ( -0.1113553986120547346, -0.9379921259842519676, -0.1113553986120547346 ) ) ;
#20191=CARTESIAN_POINT ( 'NONE',  ( -1.100456976456230270E-17, -1.506933573362572831, -0.1797182628040039365 ) ) ;
#20193=CARTESIAN_POINT ( 'NONE',  ( 0.1264236179284866091, -0.3302165353793074520, -0.1264236179284866091 ) ) ;
#20201=CARTESIAN_POINT ( 'NONE',  ( 0.1264236179284866091, 0.009350393754550925460, 0.1264236179284866091 ) ) ;
#20214=CARTESIAN_POINT ( 'NONE',  ( -0.06523048226347956391, -1.112696850286173600, 0.1574803149606297803 ) ) ;
#20215=CARTESIAN_POINT ( 'NONE',  ( 0.1787899950787401604, -1.400590551127339323, -0.07405724077823318263 ) ) ;
#20219=CARTESIAN_POINT ( 'NONE',  ( 0.000000000000000000, 0.09842519685039370636, 0.000000000000000000 ) ) ;
#20227=CARTESIAN_POINT ( 'NONE',  ( -0.09431337879932527590, -0.09445537554013608283, -0.2309807168375144215 ) ) ;
#20231=CARTESIAN_POINT ( 'NONE',  ( -0.1113553986120547346, -0.2490157479239688831, 0.1113553986120547346 ) ) ;
#20237=CARTESIAN_POINT ( 'NONE',  ( 0.1787899950787401882, -1.099041291063883818, -2.189545951927503898E-17 ) ) ;
#20239=CARTESIAN_POINT ( 'NONE',  ( -0.1787899950787401604, -0.1210629920722208208, -0.07405724077823318263 ) ) ;
#20250=CARTESIAN_POINT ( 'NONE',  ( -0.1264236179284866091, -0.6008858267178898149, -0.1264236179284866091 ) ) ;
#20253=CARTESIAN_POINT ( 'NONE',  ( 0.07444174185955065859, -1.130457195409817039, 0.1797182628040039087 ) ) ;
#20269=CARTESIAN_POINT ( 'NONE',  ( 0.1574803149606299191, -1.690944881782236120, -1.928577636452523993E-17 ) ) ;
#20271=CARTESIAN_POINT ( 'NONE',  ( 0.1781957201322358353, -0.09842519685039370636, -0.01456528979491370120 ) ) ;
#20273=CARTESIAN_POINT ( 'NONE',  ( 0.1235961452251413406, -0.09842519685039370636, 0.2140748031496062798 ) ) ;
#20274=CARTESIAN_POINT ( 'NONE',  ( 0.07405724077823318263, 0.06594488194352733645, -0.1787899950787401604 ) ) ;
#20275=DIRECTION ( 'NONE',  ( 0.000000000000000000, 0.000000000000000000, 1.000000000000000000 ) ) ;
#20281=CARTESIAN_POINT ( 'NONE',  ( 3.284318927891251994E-17, -1.688484251914740275, 0.1787899950787401882 ) ) ;
#20290=CARTESIAN_POINT ( 'NONE',  ( 2.892866454678787531E-17, -0.04724409438066189126, 0.1574803149606299191 ) ) ;
#20292=CARTESIAN_POINT ( 'NONE',  ( 0.1787899950787401882, -0.6659704249221517491, -2.189545951927503898E-17 ) ) ;
#20294=CARTESIAN_POINT ( 'NONE',  ( 0.08074247269275255934, -0.08956073568337362401, -0.1736237762710417243 ) ) ;
#20305=CARTESIAN_POINT ( 'NONE',  ( -0.1787899950787401882, -1.540846456639149542, 0.000000000000000000 ) ) ;
#20306=CARTESIAN_POINT ( 'NONE',  ( -9.642888182262618425E-18, 0.09055118120988918384, -0.1574803149606299191 ) ) ;
#20310=CARTESIAN_POINT ( 'NONE',  ( 0.1270800023317771588, -0.7244532584019429677, -0.1270800023317771588 ) ) ;
#20315=CARTESIAN_POINT ( 'NONE',  ( 0.1113553986120547346, -0.4753937007874016185, -0.1113553986120547346 ) ) ;
#20316=DIRECTION ( 'NONE',  ( 0.000000000000000000, 0.000000000000000000, 1.000000000000000000 ) ) ;
#20329=CARTESIAN_POINT ( 'NONE',  ( -0.1549096836786406084, -0.08956169654156308224, -0.08259319978823646824 ) ) ;
#20330=CARTESIAN_POINT ( 'NONE',  ( -0.1264236179284866091, -0.4680118109698582773, 0.1264236179284866091 ) ) ;
#20338=CARTESIAN_POINT ( 'NONE',  ( 0.1787899950787401604, -1.754921259788755128, 0.07405724077823318263 ) ) ;
#20339=CARTESIAN_POINT ( 'NONE',  ( -0.07405724077823318263, -0.9970472440407247561, -0.1787899950787401604 ) ) ;
#20340=CARTESIAN_POINT ( 'NONE',  ( -0.1113553986120547346, -1.410433070866141891, -0.1113553986120547346 ) ) ;
#20347=CARTESIAN_POINT ( 'NONE',  ( -0.1574803149606300301, -1.358759842412158081, -0.06523048226347956391 ) ) ;
#20348=CARTESIAN_POINT ( 'NONE',  ( 2.892866454678787531E-17, -0.007874015640504449659, 0.1574803149606299191 ) ) ;
#20360=CARTESIAN_POINT ( 'NONE',  ( 0.1101299531113933000, -0.09842519685039370636, -0.1631579918895759984 ) ) ;
#20364=DIMENSIONAL_EXPONENTS ( 1.000000000000000000, 0.000000000000000000, 0.000000000000000000, 0.000000000000000000, 0.000000000000000000, 0.000000000000000000, 0.000000000000000000 ) ;
#20367=CARTESIAN_POINT ( 'NONE',  ( 3.284318927891251994E-17, -1.211122047190330786, 0.1787899950787401882 ) ) ;
#20368=CARTESIAN_POINT ( 'NONE',  ( -0.07444174185955065859, -0.5202209749373758463, -0.1797182628040039087 ) ) ;
#20371=CARTESIAN_POINT ( 'NONE',  ( 0.1574803149606299191, -0.04724409448818897572, -1.928577636452523993E-17 ) ) ;
#20378=CARTESIAN_POINT ( 'NONE',  ( 0.1574803149606300301, -0.9798228345381415627, -0.06523048226347956391 ) ) ;
#20379=CARTESIAN_POINT ( 'NONE',  ( 0.1264236179284866091, -0.5713582676627716461, -0.1264236179284866091 ) ) ;
#20380=CARTESIAN_POINT ( 'NONE',  ( -0.07405724077823318263, -1.346456692859623550, -0.1787899950787401604 ) ) ;
#20384=ORIENTED_EDGE ( 'NONE', *, *, #6553, .F. ) ;
#20396=CARTESIAN_POINT ( 'NONE',  ( 0.1945459183828945893, -0.07553294269967773811, 0.1731116344631672688 ) ) ;
#20403=CARTESIAN_POINT ( 'NONE',  ( 0.1267340139221234119, -0.09851384784732598876, 0.1767400091468230294 ) ) ;
#20412=CARTESIAN_POINT ( 'NONE',  ( 0.1787899950787401604, -1.647761763504828947, -0.07405724077823318263 ) ) ;
#20415=CARTESIAN_POINT ( 'NONE',  ( 0.1787899950787401882, -0.5319881889226142357, -2.189545951927503898E-17 ) ) ;
#20416=CARTESIAN_POINT ( 'NONE',  ( 0.2471922904502826812, -0.09842519685039370636, -5.914624404477007554E-17 ) ) ;
#20420=CARTESIAN_POINT ( 'NONE',  ( -1.094772975963752103E-17, -0.3695866141194649179, -0.1787899950787401882 ) ) ;
#20421=CARTESIAN_POINT ( 'NONE',  ( 0.07405724077823318263, -0.7362204723871804690, 0.1787899950787401604 ) ) ;
#20425=CARTESIAN_POINT ( 'NONE',  ( 0.1264236179284866091, 0.03776973255816284264, 0.1264236179284866091 ) ) ;
#20427=CARTESIAN_POINT ( 'NONE',  ( 0.05568348810326462922, -0.09842519685039373412, 0.1550565792168007162 ) ) ;
#20431=CARTESIAN_POINT ( 'NONE',  ( -0.1574803149606297803, -0.9306102362204727863, 0.06523048226347956391 ) ) ;
#20433=CARTESIAN_POINT ( 'NONE',  ( 0.1797182628040039087, -1.519236722968871467, 0.07444174185955046430 ) ) ;
#20435=CARTESIAN_POINT ( 'NONE',  ( -0.1574803149606297803, -0.4483267715460167446, 0.06523048226347956391 ) ) ;
#20443=CARTESIAN_POINT ( 'NONE',  ( -0.1574803149606299191, -0.8838582676090078749, 0.000000000000000000 ) ) ;
#20444=CARTESIAN_POINT ( 'NONE',  ( 0.1264236179284866091, -0.03001968498560653523, 0.1264236179284866091 ) ) ;
#20446=CARTESIAN_POINT ( 'NONE',  ( 3.284318927891251994E-17, -0.9355314960092283583, 0.1787899950787401882 ) ) ;
#20456=CARTESIAN_POINT ( 'NONE',  ( 0.06523048226347956391, -1.068405511703496069, 0.1574803149606297803 ) ) ;
#20468=CARTESIAN_POINT ( 'NONE',  ( -0.07405724077823318263, 0.1200787402112438867, 0.1787899950787401604 ) ) ;
#20476=CARTESIAN_POINT ( 'NONE',  ( 0.1264236179284866091, -1.143332629646561127, 0.1264236179284866091 ) ) ;
#20478=CARTESIAN_POINT ( 'NONE',  ( -0.1264236179284866091, -0.1136811023084411398, 0.1264236179284866091 ) ) ;
#20482=CARTESIAN_POINT ( 'NONE',  ( -9.642888182262618425E-18, 0.05118110246973173183, -0.1574803149606299191 ) ) ;
#20486=CARTESIAN_POINT ( 'NONE',  ( -0.1787899950787401882, -0.6747047243556849594, 0.000000000000000000 ) ) ;
#20490=CARTESIAN_POINT ( 'NONE',  ( -0.1270800023317771588, -1.226421762338950838, -0.1270800023317771588 ) ) ;
#20500=CARTESIAN_POINT ( 'NONE',  ( 0.06523048226347956391, -0.7140748030420803749, 0.1574803149606297803 ) ) ;
#20510=CARTESIAN_POINT ( 'NONE',  ( 0.1113553986120547346, -1.686023621939716444, -0.1113553986120547346 ) ) ;
#20516=CARTESIAN_POINT ( 'NONE',  ( -0.06523048226347956391, -1.791830708661417138, 0.1574803149606297803 ) ) ;
#20524=CARTESIAN_POINT ( 'NONE',  ( 0.1787899950787401882, -1.718011810969858333, -2.189545951927503898E-17 ) ) ;
#20533=CARTESIAN_POINT ( 'NONE',  ( 0.2027848556993381846, -0.08956017357703426052, -0.01042671155077139894 ) ) ;
#20540=ORIENTED_EDGE ( 'NONE', *, *, #4304, .T. ) ;
#20547=CARTESIAN_POINT ( 'NONE',  ( -0.1574803149606299191, -0.4606299212598425341, 0.000000000000000000 ) ) ;
#20548=DIRECTION ( 'NONE',  ( 0.000000000000000000, 1.000000000000000000, 0.000000000000000000 ) ) ;
#20559=CARTESIAN_POINT ( 'NONE',  ( -0.1476731086701386642, -0.08957115901137824299, -0.09624711833952896700 ) ) ;
#20560=CARTESIAN_POINT ( 'NONE',  ( -0.1787899950787401604, -0.5541338582139530011, -0.07405724077823318263 ) ) ;
#20570=CARTESIAN_POINT ( 'NONE',  ( 0.1270800023317771588, 0.1318459541964820958, 0.1270800023317771588 ) ) ;
#20571=CARTESIAN_POINT ( 'NONE',  ( -0.1787899950787401882, -1.068405511757259951, 0.000000000000000000 ) ) ;
#20572=CARTESIAN_POINT ( 'NONE',  ( 0.1574803149606299191, -1.307086614173228467, -1.928577636452523993E-17 ) ) ;
#20585=CARTESIAN_POINT ( 'NONE',  ( 0.06215339161709781957, -0.08126078924485156951, -0.2495487439734428159 ) ) ;
#20588=CARTESIAN_POINT ( 'NONE',  ( -0.07405724077823318263, -0.2599664879142782326, -0.1787899950787401604 ) ) ;
#20589=CARTESIAN_POINT ( 'NONE',  ( 0.06243605173690295468, -0.09842519685039370636, -0.1835744151064638008 ) ) ;
#20597=CARTESIAN_POINT ( 'NONE',  ( -1.094772975963752103E-17, -1.038877952702141672, -0.1787899950787401882 ) ) ;
#20599=CARTESIAN_POINT ( 'NONE',  ( 0.1787899950787401604, -1.282480314906867314, 0.07405724077823318263 ) ) ;
#20602=CARTESIAN_POINT ( 'NONE',  ( -0.1797182628040039087, -0.5497485339924945702, 0.07444174185955065859 ) ) ;
#20607=CARTESIAN_POINT ( 'NONE',  ( 0.06523048226347956391, -0.03986220472440944740, -0.1574803149606300301 ) ) ;
#20616=CARTESIAN_POINT ( 'NONE',  ( 0.1787899950787401604, -0.6574803149068665364, 0.07405724077823318263 ) ) ;
#20617=CARTESIAN_POINT ( 'NONE',  ( 0.1787899950787401882, -1.358759842465921297, -2.189545951927503898E-17 ) ) ;
#20625=CARTESIAN_POINT ( 'NONE',  ( 0.1574803149606300301, -1.255413385719243768, -0.06523048226347956391 ) ) ;
#20627=CARTESIAN_POINT ( 'NONE',  ( 0.1344414905952618366, -0.09842522719093642347, -0.1178619895492928893 ) ) ;
#20632=CARTESIAN_POINT ( 'NONE',  ( 0.1715440989610381162, -0.08785038237333182842, 0.1863907177291471429 ) ) ;
#20639=CARTESIAN_POINT ( 'NONE',  ( 0.1815679472391334703, -0.09851384343985296332, -0.08954567948069468153 ) ) ;
#20640=ORIENTED_EDGE ( 'NONE', *, *, #2007, .F. ) ;
#20644=CARTESIAN_POINT ( 'NONE',  ( 3.284318927891251994E-17, -1.581324755630813206, 0.1787899950787401882 ) ) ;
#20646=CARTESIAN_POINT ( 'NONE',  ( 0.1264236179284866091, -0.5664370078202519698, -0.1264236179284866091 ) ) ;
#20649=CARTESIAN_POINT ( 'NONE',  ( 0.1264236179284866091, -0.2563976377415121966, -0.1264236179284866091 ) ) ;
#20650=CARTESIAN_POINT ( 'NONE',  ( -0.1787899950787401882, -0.7485236219934803259, 0.000000000000000000 ) ) ;
#20651=VECTOR ( 'NONE', #18163, 39.37007874015748143 ) ;
#20655=CARTESIAN_POINT ( 'NONE',  ( 0.1787899950787401882, 0.003320913660525051311, -2.189545951927503898E-17 ) ) ;
#20663=CARTESIAN_POINT ( 'NONE',  ( 0.1113553986120547346, -0.8297244094488188670, -0.1113553986120547346 ) ) ;
#20665=CARTESIAN_POINT ( 'NONE',  ( -0.07444174185955065859, -1.740693415882258011, -0.1797182628040039087 ) ) ;
#20666=CARTESIAN_POINT ( 'NONE',  ( -0.1574803149606297803, -0.4876968502861737664, 0.06523048226347956391 ) ) ;
#20667=CARTESIAN_POINT ( 'NONE',  ( 0.07405724077823318263, -0.3425196849856064762, 0.1787899950787401604 ) ) ;
#20674=CARTESIAN_POINT ( 'NONE',  ( -0.1945459183830246241, -0.07553294269955267148, -0.1731116344631301873 ) ) ;
#20679=CARTESIAN_POINT ( 'NONE',  ( -0.1787899950787401604, -0.1259842519147404416, -0.07405724077823318263 ) ) ;
#20681=CARTESIAN_POINT ( 'NONE',  ( 0.1787899950787401604, -0.8887795275052913224, 0.07405724077823318263 ) ) ;
#20696=ORIENTED_EDGE ( 'NONE', *, *, #13812, .T. ) ;
#20702=CARTESIAN_POINT ( 'NONE',  ( -0.2471922904502826535, 0.09442133267706682986, -0.03395025085956321353 ) ) ;
#20704=CARTESIAN_POINT ( 'NONE',  ( -0.07405724077823318263, -1.126108220197742371, -0.1787899950787401604 ) ) ;
#20706=CARTESIAN_POINT ( 'NONE',  ( 0.1787899950787401604, -0.05708661411946481384, -0.07405724077823318263 ) ) ;
#20708=EDGE_LOOP ( 'NONE', ( #25021, #29416, #42752, #14346 ) ) ;
#20715=CARTESIAN_POINT ( 'NONE',  ( 0.1797182628040039087, -0.1363627072208409285, -0.07444174185955065859 ) ) ;
#20718=CARTESIAN_POINT ( 'NONE',  ( 0.1797182628040039087, -1.238724911945250362, -0.07444174185955065859 ) ) ;
#20725=CARTESIAN_POINT ( 'NONE',  ( 0.000000000000000000, -0.09842519685039370636, 0.000000000000000000 ) ) ;
#20729=CARTESIAN_POINT ( 'NONE',  ( 2.892866454678787531E-17, -0.7165354329633386588, 0.1574803149606299191 ) ) ;
#20731=CARTESIAN_POINT ( 'NONE',  ( -1.094772975963752103E-17, -0.01033464561552785432, -0.1787899950787401882 ) ) ;
#20744=CARTESIAN_POINT ( 'NONE',  ( -0.1264236179284866091, -0.07431102356828367395, 0.1264236179284866091 ) ) ;
#20747=CARTESIAN_POINT ( 'NONE',  ( 0.1350291203832761910, 0.09842519685039370636, 0.2074739718644189046 ) ) ;
#20751=CARTESIAN_POINT ( 'NONE',  ( -1.094772975963752103E-17, -1.747539370024976391, -0.1787899950787401882 ) ) ;
#20756=CIRCLE ( 'NONE', #34558, 0.2007874015748031815 ) ;
#20757=CARTESIAN_POINT ( 'NONE',  ( 0.1574803149606299191, 0.1200787401574803237, 2.850509043694854679E-09 ) ) ;
#20780=CARTESIAN_POINT ( 'NONE',  ( -0.1574803149606300301, -0.5418307086614178036, -0.06523048226347956391 ) ) ;
#20782=CARTESIAN_POINT ( 'NONE',  ( -0.1518774605348951201, 0.1248780621282413877, -0.05777686690714941425 ) ) ;
#20795=CARTESIAN_POINT ( 'NONE',  ( 0.1099100077094851968, 0.1299212598425196763, 0.1429462536667461814 ) ) ;
#20802=CARTESIAN_POINT ( 'NONE',  ( -0.1270800023317771588, 0.1121609148264033490, -0.1270800023317771588 ) ) ;
#20803=CARTESIAN_POINT ( 'NONE',  ( -1.094772975963752103E-17, -0.9995078739619842612, -0.1787899950787401882 ) ) ;
#20804=CARTESIAN_POINT ( 'NONE',  ( -0.06523048226347956391, -1.398129921259843478, 0.1574803149606297803 ) ) ;
#20811=CARTESIAN_POINT ( 'NONE',  ( -9.642888182262618425E-18, -1.405511810916094451, -0.1574803149606299191 ) ) ;
#20818=CARTESIAN_POINT ( 'NONE',  ( -0.1768440709656272092, 0.08559642391439407916, -0.1833320988895476844 ) ) ;
#20822=CARTESIAN_POINT ( 'NONE',  ( -0.1787899950787401604, -0.2107538894890813030, 0.07405724077823318263 ) ) ;
#20823=CARTESIAN_POINT ( 'NONE',  ( 0.09661541192592146277, -0.09842519685039370636, 0.1970456418925724540 ) ) ;
#20833=CARTESIAN_POINT ( 'NONE',  ( 0.1264236179284866091, -1.043799212544661348, -0.1264236179284866091 ) ) ;
#20834=CARTESIAN_POINT ( 'NONE',  ( 0.1264236179284866091, -1.156988188922614125, -0.1264236179284866091 ) ) ;
#20837=CARTESIAN_POINT ( 'NONE',  ( 0.07444174185955046430, -0.5645123135200530440, -0.1797182628040039087 ) ) ;
#20841=CARTESIAN_POINT ( 'NONE',  ( -0.1113553986120547346, -0.06200787401574803237, 0.1113553986120547346 ) ) ;
#20851=CARTESIAN_POINT ( 'NONE',  ( -0.1787899950787401604, -0.5196850393163150450, -0.07405724077823318263 ) ) ;
#20852=CARTESIAN_POINT ( 'NONE',  ( -0.1264236179284866091, -1.412893700733637958, 0.1264236179284866091 ) ) ;
#20860=AXIS2_PLACEMENT_3D ( 'NONE', #25692, #32652, #10835 ) ;
#20874=CARTESIAN_POINT ( 'NONE',  ( -0.1855074086109543274, -0.09851385092611850136, 0.1431435806659169252 ) ) ;
#20878=CARTESIAN_POINT ( 'NONE',  ( -0.07405724077823318263, -1.637919243819790704, -0.1787899950787401604 ) ) ;
#20881=CARTESIAN_POINT ( 'NONE',  ( -0.1264236179284866091, -0.6353346456155275490, -0.1264236179284866091 ) ) ;
#20887=CARTESIAN_POINT ( 'NONE',  ( 0.07405724077823318263, -0.3474409448281265411, 0.1787899950787401604 ) ) ;
#20888=CARTESIAN_POINT ( 'NONE',  ( 0.1264236179284866091, -0.8124999999462361178, 0.1264236179284866091 ) ) ;
#20895=CARTESIAN_POINT ( 'NONE',  ( -0.1787899950787401604, -0.2342519684501733479, 0.07405724077823318263 ) ) ;
#20896=CARTESIAN_POINT ( 'NONE',  ( 0.1264236179284866091, 0.09793307091990532953, -0.1264236179284866091 ) ) ;
#20900=CARTESIAN_POINT ( 'NONE',  ( 0.06523048226347956391, -0.8420275590551181688, 0.1574803149606297803 ) ) ;
#20901=CARTESIAN_POINT ( 'NONE',  ( 0.07444174185955046430, -1.784984754464935541, -0.1797182628040039087 ) ) ;
#20902=CARTESIAN_POINT ( 'NONE',  ( -0.1787899950787401882, -0.3548228345919058890, 0.000000000000000000 ) ) ;
#20911=CARTESIAN_POINT ( 'NONE',  ( 0.07405724077823318263, -0.1112204723871813017, 0.1787899950787401604 ) ) ;
#20914=CARTESIAN_POINT ( 'NONE',  ( -0.1787899950787401604, -0.8690944881352120621, -0.07405724077823318263 ) ) ;
#20932=ORIENTED_EDGE ( 'NONE', *, *, #1297, .T. ) ;
#20938=CARTESIAN_POINT ( 'NONE',  ( 3.284318927891251994E-17, -1.148253889489080803, 0.1787899950787401882 ) ) ;
#20941=CARTESIAN_POINT ( 'NONE',  ( -1.094772975963752103E-17, -0.04970472435568527164, -0.1787899950787401882 ) ) ;
#20943=EDGE_CURVE ( 'NONE', #6112, #2820, #25758, .T. ) ;
#20949=CARTESIAN_POINT ( 'NONE',  ( -1.100456976456230270E-17, -1.270713100921627703, -0.1797182628040039365 ) ) ;
#20957=CARTESIAN_POINT ( 'NONE',  ( -0.1787899950787401604, 0.03641732288840918152, -0.07405724077823318263 ) ) ;
#20972=CARTESIAN_POINT ( 'NONE',  ( 0.1787899950787401604, -0.05708661411946481384, -0.07405724077823318263 ) ) ;
#20975=CARTESIAN_POINT ( 'NONE',  ( 0.1910524284696302755, 0.07767250275969661555, 0.1751288998598690416 ) ) ;
#20976=DIRECTION ( 'NONE',  ( 0.000000000000000000, -1.000000000000000000, 0.000000000000000000 ) ) ;
#20981=CARTESIAN_POINT ( 'NONE',  ( -9.642888182262618425E-18, -0.4212598424121582474, -0.1574803149606299191 ) ) ;
#20982=CARTESIAN_POINT ( 'NONE',  ( -0.07405724077823318263, -1.769685039316315267, 0.1787899950787401604 ) ) ;
#20988=CARTESIAN_POINT ( 'NONE',  ( -0.1264236179284866091, -0.7201042831898681884, 0.1264236179284866091 ) ) ;
#20990=CARTESIAN_POINT ( 'NONE',  ( -0.1505467838310571016, -0.08956164613504763450, 0.06735808213815078216 ) ) ;
#20998=CARTESIAN_POINT ( 'NONE',  ( -9.642888182262618425E-18, 0.001968503937007873988, -0.1574803149606299191 ) ) ;
#21007=CARTESIAN_POINT ( 'NONE',  ( 0.1797182628040039087, -0.7712052269058795595, 0.07444174185955046430 ) ) ;
#21010=CARTESIAN_POINT ( 'NONE',  ( -0.1574803149606297803, -0.6156496062992122820, 0.06523048226347956391 ) ) ;
#21011=CARTESIAN_POINT ( 'NONE',  ( 0.2471922904502825424, 0.04213860324412696534, -0.1312291345420432964 ) ) ;
#21026=AXIS2_PLACEMENT_3D ( 'NONE', #44098, #46981, #17515 ) ;
#21029=EDGE_CURVE ( 'NONE', #2394, #3498, #42161, .T. ) ;
#21032=CARTESIAN_POINT ( 'NONE',  ( 0.1797182628040039365, 0.05802705655868669460, -2.200913952912460540E-17 ) ) ;
#21033=CARTESIAN_POINT ( 'NONE',  ( 0.1787899950787401604, -1.011811023568284451, 0.07405724077823318263 ) ) ;
#21034=CARTESIAN_POINT ( 'NONE',  ( -9.642888182262618425E-18, -1.454724409448818756, -0.1574803149606299191 ) ) ;
#21048=CARTESIAN_POINT ( 'NONE',  ( -0.2471922904502826535, 0.04213860324413871983, 0.1312291345420296129 ) ) ;
#21050=CARTESIAN_POINT ( 'NONE',  ( 0.06756161724125105128, -0.08412760742795728774, -0.2464250160559827429 ) ) ;
#21053=CARTESIAN_POINT ( 'NONE',  ( -0.1264236179284866091, -0.2181357792528606510, -0.1264236179284866091 ) ) ;
#21054=CARTESIAN_POINT ( 'NONE',  ( -9.642888182262618425E-18, 0.001968503937007873988, -0.1574803149606299191 ) ) ;
#21063=CARTESIAN_POINT ( 'NONE',  ( -0.1787899950787401604, -1.144685039316316599, 0.07405724077823318263 ) ) ;
#21064=CARTESIAN_POINT ( 'NONE',  ( -0.1787899950787401882, -1.220964566875370139, 0.000000000000000000 ) ) ;
#21067=CARTESIAN_POINT ( 'NONE',  ( 0.1270800023317771588, -0.5276028647011559158, -0.1270800023317771588 ) ) ;
#21071=CARTESIAN_POINT ( 'NONE',  ( 0.1574803149606300301, -0.08415354330708657571, -0.06523048226347956391 ) ) ;
#21084=CARTESIAN_POINT ( 'NONE',  ( -0.1264236179284866091, -0.6402559054580471143, -0.1264236179284866091 ) ) ;
#21085=CARTESIAN_POINT ( 'NONE',  ( -0.1113553986120547346, -1.016732283464566899, -0.1113553986120547346 ) ) ;
#21087=EDGE_CURVE ( 'NONE', #5618, #3128, #42848, .T. ) ;
#21093=EDGE_CURVE ( 'NONE', #28863, #27412, #21143, .T. ) ;
#21103=CARTESIAN_POINT ( 'NONE',  ( -0.1574803149606300301, -0.1382874014672760277, -0.06523048226347956391 ) ) ;
#21108=CARTESIAN_POINT ( 'NONE',  ( 0.05242207689368432594, -0.09851384127917696409, -0.1861051744488299298 ) ) ;
#21112=CARTESIAN_POINT ( 'NONE',  ( -0.1787899950787401882, -1.709277511536324790, 0.000000000000000000 ) ) ;
#21114=CARTESIAN_POINT ( 'NONE',  ( 0.2471922904502826812, -0.09842519685039370636, -5.914624404477007554E-17 ) ) ;
#21121=CARTESIAN_POINT ( 'NONE',  ( 3.284318927891251994E-17, -0.2711614172690712810, 0.1787899950787401882 ) ) ;
#21122=CARTESIAN_POINT ( 'NONE',  ( -0.1264236179284866091, -0.7140748030958424808, -0.1264236179284866091 ) ) ;
#21126=CARTESIAN_POINT ( 'NONE',  ( -0.1264236179284866091, -0.05081294460719149725, 0.1264236179284866091 ) ) ;
#21127=CARTESIAN_POINT ( 'NONE',  ( 0.1787899950787401882, 0.01427165359707061217, -2.189545951927503898E-17 ) ) ;
#21133=CARTESIAN_POINT ( 'NONE',  ( 0.06523048226347956391, -0.9601377952755901779, 0.1574803149606297803 ) ) ;
#21135=CARTESIAN_POINT ( 'NONE',  ( 0.1797182628040039365, -1.713626486748399680, -2.200913952912460540E-17 ) ) ;
#21140=CARTESIAN_POINT ( 'NONE',  ( -0.1925175471592172338, -0.07678538764761655422, -0.1742829424377035086 ) ) ;
#21142=CARTESIAN_POINT ( 'NONE',  ( 0.1787899950787401604, -0.1456692912848192578, 0.07405724077823318263 ) ) ;
#21143=B_SPLINE_CURVE_WITH_KNOTS ( 'NONE', 3,
 ( #27400, #360, #7788, #40362, #15241, #11646, #36799, #4182, #16123, #41942, #3952, #19924, #29887, #38376, #25791, #33232, #18808, #33465, #30978, #29662, #8912, #37259, #7552 ),
 .UNSPECIFIED., .F., .F.,
 ( 4, 2, 2, 1, 1, 1, 2, 2, 2, 1, 1, 2, 2, 4 ),
 ( 0.000000000000000000, 0.2500000000000059397, 0.3750000000000091593, 0.4375000000000106026, 0.4687500000000113798, 0.4843750000000119349, 0.4921875000000120459, 0.5000000000000121014, 0.6250000000000104361, 0.6875000000000094369, 0.7187500000000087708, 0.7343750000000082157, 0.7500000000000076605, 1.000000000000000000 ),
 .UNSPECIFIED. ) ;
#21145=CARTESIAN_POINT ( 'NONE',  ( -0.07405724077823318263, -0.8740157479777336258, -0.1787899950787401604 ) ) ;
#21165=CARTESIAN_POINT ( 'NONE',  ( 0.1787899950787401882, -0.06446850388324429360, -2.189545951927503898E-17 ) ) ;
#21168=CARTESIAN_POINT ( 'NONE',  ( 0.1787899950787401604, -1.479330708607653699, 0.07405724077823318263 ) ) ;
#21172=CARTESIAN_POINT ( 'NONE',  ( 0.07405724077823318263, -1.303273574528451384, 0.1787899950787401604 ) ) ;
#21174=CARTESIAN_POINT ( 'NONE',  ( -0.1264236179284866091, -0.1530511810485988278, 0.1264236179284866091 ) ) ;
#21181=CARTESIAN_POINT ( 'NONE',  ( -0.1264236179284866091, -1.457185039316315045, 0.1264236179284866091 ) ) ;
#21183=CARTESIAN_POINT ( 'NONE',  ( 0.1264236179284866091, -0.7288385826234015097, -0.1264236179284866091 ) ) ;
#21185=CARTESIAN_POINT ( 'NONE',  ( 0.1270800023317771588, -1.285476880449186954, 0.1270800023317771588 ) ) ;
#21191=CARTESIAN_POINT ( 'NONE',  ( 0.008579867197626878106, 0.1299212598425198151, 0.1749887852363761209 ) ) ;
#21204=ORIENTED_EDGE ( 'NONE', *, *, #26383, .F. ) ;
#21210=ADVANCED_FACE ( 'NONE', ( #46736 ), #16806, .F. ) ;
#21213=CARTESIAN_POINT ( 'NONE',  ( -1.094772975963752103E-17, 0.02903543312462964626, -0.1787899950787401882 ) ) ;
#21223=CARTESIAN_POINT ( 'NONE',  ( 0.1574803149606299191, -0.4311023620971976555, -1.928577636452523993E-17 ) ) ;
#21224=CARTESIAN_POINT ( 'NONE',  ( 0.07405724077823318263, -1.631889763725764553, -0.1787899950787401604 ) ) ;
#21233=CARTESIAN_POINT ( 'NONE',  ( -0.1787899950787401604, -0.8455964091741210442, -0.07405724077823318263 ) ) ;
#21235=CARTESIAN_POINT ( 'NONE',  ( 0.07139542023256004177, -0.08956251728346555085, 0.1284121166753139920 ) ) ;
#21240=CARTESIAN_POINT ( 'NONE',  ( 0.1574803149606300301, -0.005413385826771673418, -0.06523048226347956391 ) ) ;
#21250=CARTESIAN_POINT ( 'NONE',  ( 0.07444174185955046430, -0.9188430221814710697, -0.1797182628040039087 ) ) ;
#21255=CARTESIAN_POINT ( 'NONE',  ( 0.1113553986120547346, -0.5639763779527559029, 0.1113553986120547346 ) ) ;
#21256=CARTESIAN_POINT ( 'NONE',  ( -0.1360083797011654438, 0.1240348912602861897, -0.08737303594299716814 ) ) ;
#21262=EDGE_CURVE ( 'NONE', #22666, #36464, #21786, .T. ) ;
#21272=CARTESIAN_POINT ( 'NONE',  ( 0.1270800023317771588, 0.09247587545632461603, 0.1270800023317771588 ) ) ;
#21273=CARTESIAN_POINT ( 'NONE',  ( -0.1787899950787401882, -1.107775590497417362, 0.000000000000000000 ) ) ;
#21274=CARTESIAN_POINT ( 'NONE',  ( 2.892866454678787531E-17, -1.592519685039370136, 0.1574803149606299191 ) ) ;
#21285=CARTESIAN_POINT ( 'NONE',  ( -0.1916154494608382219, 0.07733267719194408807, -0.1748038395390359157 ) ) ;
#21290=CARTESIAN_POINT ( 'NONE',  ( 0.1787899950787401604, -0.2698090075993175296, -0.07405724077823318263 ) ) ;
#21292=FACE_OUTER_BOUND ( 'NONE', #31277, .T. ) ;
#21298=CARTESIAN_POINT ( 'NONE',  ( 3.284318927891251994E-17, -1.216043307032850462, 0.1787899950787401882 ) ) ;
#21299=CARTESIAN_POINT ( 'NONE',  ( 0.1787899950787401882, -1.319389763725763665, -2.189545951927503898E-17 ) ) ;
#21301=DIRECTION ( 'NONE',  ( 0.000000000000000000, 0.000000000000000000, 1.000000000000000000 ) ) ;
#21302=CARTESIAN_POINT ( 'NONE',  ( -1.100456976456230270E-17, -0.6407918410791082486, -0.1797182628040039365 ) ) ;
#21306=CARTESIAN_POINT ( 'NONE',  ( 0.1113553986120547346, -0.1604330708661417249, -0.1113553986120547346 ) ) ;
#21320=CARTESIAN_POINT ( 'NONE',  ( -9.642888182262618425E-18, -1.562992125876726535, -0.1574803149606299191 ) ) ;
#21321=CARTESIAN_POINT ( 'NONE',  ( 0.1787899950787401882, -0.5369094487651339120, -2.189545951927503898E-17 ) ) ;
#21322=CARTESIAN_POINT ( 'NONE',  ( 0.1574803149606300301, -0.9945866141732289112, 0.06523048226347956391 ) ) ;
#21336=CARTESIAN_POINT ( 'NONE',  ( 0.000000000000000000, -0.09842519685039370636, 0.000000000000000000 ) ) ;
#21337=VECTOR ( 'NONE', #38427, 39.37007874015748143 ) ;
#21339=CARTESIAN_POINT ( 'NONE',  ( 0.06523048226347956391, -0.2662401573727879445, -0.1574803149606300301 ) ) ;
#21346=CARTESIAN_POINT ( 'NONE',  ( -0.1674536925976815027, -0.09851383442626908404, 0.03546406509531940809 ) ) ;
#21348=CIRCLE ( 'NONE', #4495, 0.2471922904502826812 ) ;
#21349=CARTESIAN_POINT ( 'NONE',  ( -0.1264236179284866091, -1.674828692638687277, -0.1264236179284866091 ) ) ;
#21356=CARTESIAN_POINT ( 'NONE',  ( -1.094772975963752103E-17, -0.3302165353793074520, -0.1787899950787401882 ) ) ;
#21358=CARTESIAN_POINT ( 'NONE',  ( -1.094772975963752103E-17, -0.8371062991588346103, -0.1787899950787401882 ) ) ;
#21363=CARTESIAN_POINT ( 'NONE',  ( 0.1787899950787401604, -0.1516987713788451320, -0.07405724077823318263 ) ) ;
#21364=CARTESIAN_POINT ( 'NONE',  ( 0.1787899950787401604, -0.2933070865604095467, -0.07405724077823318263 ) ) ;
#21365=CARTESIAN_POINT ( 'NONE',  ( -0.1787899950787401604, 0.07578740162856664742, 0.07405724077823318263 ) ) ;
#21368=EDGE_CURVE ( 'NONE', #33104, #30751, #3745, .T. ) ;
#21375=CARTESIAN_POINT ( 'NONE',  ( -0.1270800023317771588, -1.777602864701157692, -0.1270800023317771588 ) ) ;
#21383=CARTESIAN_POINT ( 'NONE',  ( -0.1264236179284866091, -0.1284448818360001965, -0.1264236179284866091 ) ) ;
#21386=CARTESIAN_POINT ( 'NONE',  ( 0.1264236179284866091, -1.038877952702141672, -0.1264236179284866091 ) ) ;
#21393=CARTESIAN_POINT ( 'NONE',  ( 0.1113553986120547346, -1.144685039262551163, 0.1113553986120547346 ) ) ;
#21394=LINE ( 'NONE', #13979, #17186 ) ;
#21405=CARTESIAN_POINT ( 'NONE',  ( 0.1787899950787401604, 0.05610236225848794223, -0.07405724077823318263 ) ) ;
#21409=CARTESIAN_POINT ( 'NONE',  ( -0.2471922904502826812, 0.09773636000336974328, -0.01649811039748649497 ) ) ;
#21412=CARTESIAN_POINT ( 'NONE',  ( -0.1264236179284866091, -1.241757826496954875, -0.1264236179284866091 ) ) ;
#21414=CARTESIAN_POINT ( 'NONE',  ( 0.1264236179284866091, -0.2219488188438744347, 0.1264236179284866091 ) ) ;
#21422=CARTESIAN_POINT ( 'NONE',  ( -0.07405724077823318263, -1.612204724355685403, 0.1787899950787401604 ) ) ;
#21425=CARTESIAN_POINT ( 'NONE',  ( 0.1270800023317771588, -1.275634360764147601, -0.1270800023317771588 ) ) ;
#21435=CARTESIAN_POINT ( 'NONE',  ( -0.1264236179284866091, 0.04379921265218866822, 0.1264236179284866091 ) ) ;
#21450=CARTESIAN_POINT ( 'NONE',  ( 0.07405724077823318263, 0.01181102367581074800, 0.1787899950787401604 ) ) ;
#21460=CARTESIAN_POINT ( 'NONE',  ( -0.1787899950787401604, -1.774606299158834277, 0.07405724077823318263 ) ) ;
#21467=CARTESIAN_POINT ( 'NONE',  ( 3.284318927891251994E-17, -0.8726633383079782647, 0.1787899950787401882 ) ) ;
#21469=CARTESIAN_POINT ( 'NONE',  ( -0.1126596323294454804, -0.08956130712551850503, 0.1148527042348372190 ) ) ;
#21487=CARTESIAN_POINT ( 'NONE',  ( 3.301370929368692659E-17, -0.8179571954098169284, 0.1797182628040039365 ) ) ;
#21491=CARTESIAN_POINT ( 'NONE',  ( 0.1574803149606299191, -0.6377952755905511584, -1.928577636452523993E-17 ) ) ;
#21500=CARTESIAN_POINT ( 'NONE',  ( -0.1264236179284866091, -0.6648622046706456068, 0.1264236179284866091 ) ) ;
#21507=CARTESIAN_POINT ( 'NONE',  ( -1.100456976456230270E-17, 0.02849949750356862294, -0.1797182628040039365 ) ) ;
#21508=CARTESIAN_POINT ( 'NONE',  ( -1.094772975963752103E-17, -1.196358267662771757, -0.1787899950787401882 ) ) ;
#21509=CARTESIAN_POINT ( 'NONE',  ( -0.1574803149606297803, -1.481791338582676643, 0.06523048226347956391 ) ) ;
#21516=CARTESIAN_POINT ( 'NONE',  ( 3.284318927891251994E-17, -1.412893700733637958, 0.1787899950787401882 ) ) ;
#21529=CARTESIAN_POINT ( 'NONE',  ( -0.07405724077823318263, -0.4026830233473494003, 0.1787899950787401604 ) ) ;
#21531=CARTESIAN_POINT ( 'NONE',  ( -0.1028752476446956748, -0.09842519685039370636, 0.1273875674447041140 ) ) ;
#21542=CARTESIAN_POINT ( 'NONE',  ( -0.07405724077823318263, -1.179133858213953001, 0.1787899950787401604 ) ) ;
#21543=CARTESIAN_POINT ( 'NONE',  ( 0.07405724077823318263, -1.390748031442299082, -0.1787899950787401604 ) ) ;
#21565=CARTESIAN_POINT ( 'NONE',  ( 2.892866454678787531E-17, -1.543307086506645609, 0.1574803149606299191 ) ) ;
#21566=CARTESIAN_POINT ( 'NONE',  ( 3.284318927891251994E-17, -0.7829724408911181710, 0.1787899950787401882 ) ) ;
#21568=CARTESIAN_POINT ( 'NONE',  ( 0.1574803149606299191, -1.031496062992126150, -1.928577636452523993E-17 ) ) ;
#21587=CARTESIAN_POINT ( 'NONE',  ( 0.1574803149606300301, -0.1530511809948351398, -0.06523048226347956391 ) ) ;
#21595=CARTESIAN_POINT ( 'NONE',  ( 0.03196715850396897318, -0.09851384192498563452, -0.1894913400051448926 ) ) ;
#21600=CARTESIAN_POINT ( 'NONE',  ( 0.07405724077823318263, -1.760950739882781502, -0.1787899950787401604 ) ) ;
#21605=CARTESIAN_POINT ( 'NONE',  ( 0.1264236179284866091, -0.4237204723871811352, 0.1264236179284866091 ) ) ;
#21606=CARTESIAN_POINT ( 'NONE',  ( 0.07405724077823318263, -0.9183070865604088251, -0.1787899950787401604 ) ) ;
#21611=CARTESIAN_POINT ( 'NONE',  ( -0.1797182628040039087, -0.1215989276932817470, -0.07444174185955065859 ) ) ;
#21612=CARTESIAN_POINT ( 'NONE',  ( 0.1787899950787401604, -0.1910688501190024868, -0.07405724077823318263 ) ) ;
#21613=CARTESIAN_POINT ( 'NONE',  ( 0.07405724077823318263, -0.2637795275052916555, 0.1787899950787401604 ) ) ;
#21614=CARTESIAN_POINT ( 'NONE',  ( 3.284318927891251994E-17, -0.07431102356828367395, 0.1787899950787401882 ) ) ;
#21621=CARTESIAN_POINT ( 'NONE',  ( -0.1270800023317771588, -1.659492628480683019, -0.1270800023317771588 ) ) ;
#21624=CARTESIAN_POINT ( 'NONE',  ( -0.1766724065096720031, -0.08549467455868767218, 0.1834299084088460152 ) ) ;
#21629=CARTESIAN_POINT ( 'NONE',  ( -0.1574803149606297803, -0.9207677164279066684, 0.06523048226347956391 ) ) ;
#21630=CARTESIAN_POINT ( 'NONE',  ( 0.07405724077823318263, -0.1751968503399373434, -0.1787899950787401604 ) ) ;
#21633=CARTESIAN_POINT ( 'NONE',  ( 0.1264236179284866091, -1.078248031442299304, -0.1264236179284866091 ) ) ;
#21641=CARTESIAN_POINT ( 'NONE',  ( -0.1113553986120547346, -1.115157480207433105, 0.1113553986120547346 ) ) ;
#21655=CARTESIAN_POINT ( 'NONE',  ( 0.1787899950787401604, 0.01673228351833045899, -0.07405724077823318263 ) ) ;
#21662=CIRCLE ( 'NONE', #23163, 0.2204724409448818867 ) ;
#21664=CARTESIAN_POINT ( 'NONE',  ( -1.094772975963752103E-17, -1.246679086339474551, -0.1787899950787401882 ) ) ;
#21666=CARTESIAN_POINT ( 'NONE',  ( 0.1264236179284866091, -0.3302165353793074520, -0.1264236179284866091 ) ) ;
#21667=ORIENTED_EDGE ( 'NONE', *, *, #41444, .T. ) ;
#21675=CARTESIAN_POINT ( 'NONE',  ( 0.1264236179284866091, -0.7780511810485984947, 0.1264236179284866091 ) ) ;
#21678=CARTESIAN_POINT ( 'NONE',  ( 0.1797182628040039365, -1.280555620606667278, -2.200913952912460540E-17 ) ) ;
#21683=CARTESIAN_POINT ( 'NONE',  ( -0.05116749466471032931, 0.1299212598425196763, 0.1641566192618154341 ) ) ;
#21687=CARTESIAN_POINT ( 'NONE',  ( 2.892866454678787531E-17, -0.7952755904436534795, 0.1574803149606299191 ) ) ;
#21703=CARTESIAN_POINT ( 'NONE',  ( -0.1787899950787401604, 0.03641732288840918152, -0.07405724077823318263 ) ) ;
#21714=CARTESIAN_POINT ( 'NONE',  ( -0.1113553986120547346, 0.1053149607374482266, 0.1113553986120547346 ) ) ;
#21717=ORIENTED_EDGE ( 'NONE', *, *, #21029, .T. ) ;
#21724=CARTESIAN_POINT ( 'NONE',  ( -0.1264236179284866091, -0.8874271178355372935, -0.1264236179284866091 ) ) ;
#21726=CARTESIAN_POINT ( 'NONE',  ( 0.1787899950787401882, 0.1373031496600628232, -2.189545951927503898E-17 ) ) ;
#21737=CARTESIAN_POINT ( 'NONE',  ( 0.07444174185955046430, -0.8007327859609992826, -0.1797182628040039087 ) ) ;
#21742=CARTESIAN_POINT ( 'NONE',  ( -0.1574803149606300301, -0.5812007874015742148, -0.06523048226347956391 ) ) ;
#21743=CARTESIAN_POINT ( 'NONE',  ( -0.1026092249587055166, 0.1299212598425196763, 0.1321676130798911386 ) ) ;
#21748=CARTESIAN_POINT ( 'NONE',  ( -0.02739131347899105909, -0.09752745740044843625, 0.1550798682808147422 ) ) ;
#21750=CARTESIAN_POINT ( 'NONE',  ( -0.1113553986120547346, -0.6427165353255432922, 0.1113553986120547346 ) ) ;
#21753=CARTESIAN_POINT ( 'NONE',  ( 0.07405724077823318263, -0.6574803149068665364, 0.1787899950787401604 ) ) ;
#21759=CARTESIAN_POINT ( 'NONE',  ( 0.07405724077823318263, -1.198818897584032150, -0.1787899950787401604 ) ) ;
#21765=CARTESIAN_POINT ( 'NONE',  ( -0.1574803149606297803, 0.06348425207603099196, 0.06523048226347956391 ) ) ;
#21766=CARTESIAN_POINT ( 'NONE',  ( -0.06523048226347956391, -0.3252952754830241155, 0.1574803149606297803 ) ) ;
#21767=CARTESIAN_POINT ( 'NONE',  ( 0.07405724077823318263, -1.410433070812377565, 0.1787899950787401604 ) ) ;
#21775=CARTESIAN_POINT ( 'NONE',  ( 0.1235961452251413406, -0.09842519685039370636, -0.2140748031496062798 ) ) ;
#21779=CARTESIAN_POINT ( 'NONE',  ( 0.1264236179284866091, -0.4248286926386873885, -0.1264236179284866091 ) ) ;
#21786=B_SPLINE_CURVE_WITH_KNOTS ( 'NONE', 3,
 ( #9395, #2413, #13460, #5791, #9631, #13677, #13923, #20396, #17511, #42651, #39548, #46026, #13238, #27866, #20632, #28568, #38844, #6721, #6012, #35968, #17753, #45787, #35277 ),
 .UNSPECIFIED., .F., .F.,
 ( 4, 2, 2, 1, 1, 1, 2, 2, 2, 1, 1, 2, 2, 4 ),
 ( 0.000000000000000000, 0.2500000000000004996, 0.3750000000000006661, 0.4375000000000008327, 0.4687500000000011657, 0.4843750000000014433, 0.4921875000000015543, 0.5000000000000015543, 0.6249999999999980016, 0.6874999999999958922, 0.7187499999999952260, 0.7343749999999952260, 0.7499999999999952260, 1.000000000000000000 ),
 .UNSPECIFIED. ) ;
#21790=CARTESIAN_POINT ( 'NONE',  ( -0.1264236179284866091, -1.181594488135212506, 0.1264236179284866091 ) ) ;
#21792=CARTESIAN_POINT ( 'NONE',  ( -0.1264236179284866091, -1.422736220418677311, -0.1264236179284866091 ) ) ;
#21799=CARTESIAN_POINT ( 'NONE',  ( 0.06523048226347956391, -0.09399606299212612259, 0.1574803149606297803 ) ) ;
#21812=CARTESIAN_POINT ( 'NONE',  ( 0.07405724077823318263, -1.626968503883244876, -0.1787899950787401604 ) ) ;
#21813=CARTESIAN_POINT ( 'NONE',  ( 0.06523048226347956391, -1.565452755797984263, -0.1574803149606300301 ) ) ;
#21814=CARTESIAN_POINT ( 'NONE',  ( 0.1787899950787401604, -0.6919291338045056028, -0.07405724077823318263 ) ) ;
#21816=CARTESIAN_POINT ( 'NONE',  ( 0.06523048226347956391, -1.038877952755906442, 0.1574803149606297803 ) ) ;
#21823=CARTESIAN_POINT ( 'NONE',  ( 0.1113553986120547346, -1.292322834538141674, -0.1113553986120547346 ) ) ;
#21832=CARTESIAN_POINT ( 'NONE',  ( -0.1574803149606297803, -0.1333661416247563514, 0.06523048226347956391 ) ) ;
#21839=CARTESIAN_POINT ( 'NONE',  ( -0.1537669602759263732, -0.09851383235754725132, 0.06906785912561810847 ) ) ;
#21842=CARTESIAN_POINT ( 'NONE',  ( 0.07405724077823318263, -1.721580661142623869, -0.1787899950787401604 ) ) ;
#21847=CARTESIAN_POINT ( 'NONE',  ( -0.1787899950787401604, -0.3966535432533230265, 0.07405724077823318263 ) ) ;
#21848=CARTESIAN_POINT ( 'NONE',  ( -0.1787899950787401604, -0.9872047243556864027, -0.07405724077823318263 ) ) ;
#21849=CARTESIAN_POINT ( 'NONE',  ( -0.2471922927914643187, -0.07821957050364394815, -0.07683452368279758415 ) ) ;
#21851=CARTESIAN_POINT ( 'NONE',  ( 0.07444174185955046430, -0.2101816048586362673, -0.1797182628040039087 ) ) ;
#21853=CARTESIAN_POINT ( 'NONE',  ( 0.07405724077823318263, -0.1615412910638844290, 0.1787899950787401604 ) ) ;
#21854=CARTESIAN_POINT ( 'NONE',  ( 0.07405724077823318263, -0.09645669285962235606, -0.1787899950787401604 ) ) ;
#21855=CYLINDRICAL_SURFACE ( 'NONE', #28055, 0.1574803149606299191 ) ;
#21861=CARTESIAN_POINT ( 'NONE',  ( 0.1787899950787401882, -0.4532480314422991929, -2.189545951927503898E-17 ) ) ;
#21864=CARTESIAN_POINT ( 'NONE',  ( -0.1235961452251413406, -0.09842519685039370636, 0.2140748031496062798 ) ) ;
#21872=CARTESIAN_POINT ( 'NONE',  ( 0.07405724077823318263, -0.2539370078202523584, -0.1787899950787401604 ) ) ;
#21875=CARTESIAN_POINT ( 'NONE',  ( -0.1787899950787401604, -1.105314960576158301, -0.07405724077823318263 ) ) ;
#21893=CARTESIAN_POINT ( 'NONE',  ( -0.1264236179284866091, 0.06840551186478720236, -0.1264236179284866091 ) ) ;
#21899=CARTESIAN_POINT ( 'NONE',  ( 0.1787899950787401604, -1.337722393426090228, 0.07405724077823318263 ) ) ;
#21901=CARTESIAN_POINT ( 'NONE',  ( 0.1787899950787401882, -0.2170275590013547307, -2.189545951927503898E-17 ) ) ;
#21902=CARTESIAN_POINT ( 'NONE',  ( -0.1574803149606297803, 0.02411417333587350526, 0.06523048226347956391 ) ) ;
#21910=CARTESIAN_POINT ( 'NONE',  ( -0.07405724077823318263, -1.572834645615527327, 0.1787899950787401604 ) ) ;
#21911=CARTESIAN_POINT ( 'NONE',  ( -0.1787899950787401604, -1.690944881836001334, 0.07405724077823318263 ) ) ;
#21915=CARTESIAN_POINT ( 'NONE',  ( 0.1270800023317771588, -1.324846959189344364, 0.1270800023317771588 ) ) ;
#21942=CARTESIAN_POINT ( 'NONE',  ( -0.1264236179284866091, -0.1924212597887563214, 0.1264236179284866091 ) ) ;
#21949=CARTESIAN_POINT ( 'NONE',  ( 0.06523048226347956391, 0.1274606300287869365, -0.1574803149606300301 ) ) ;
#21957=CARTESIAN_POINT ( 'NONE',  ( 3.284318927891251994E-17, -0.7545531020875060335, 0.1787899950787401882 ) ) ;
#21969=CARTESIAN_POINT ( 'NONE',  ( -0.07444174185955065859, -0.8204178253310762114, 0.1797182628040039087 ) ) ;
#21975=CARTESIAN_POINT ( 'NONE',  ( -0.2471922904502826812, -0.09842519685039370636, -0.1427165354330708902 ) ) ;
#21980=ORIENTED_EDGE ( 'NONE', *, *, #45161, .F. ) ;
#21984=CARTESIAN_POINT ( 'NONE',  ( -0.07405724077823318263, -0.8198818897100156322, 0.1787899950787401604 ) ) ;
#21991=CARTESIAN_POINT ( 'NONE',  ( -0.1574803149606297803, -1.560531496062992574, 0.06523048226347956391 ) ) ;
#21996=CARTESIAN_POINT ( 'NONE',  ( -0.1787899950787401882, -1.422736220418677311, 0.000000000000000000 ) ) ;
#22000=CARTESIAN_POINT ( 'NONE',  ( -9.642888182262618425E-18, -0.02755905501058318954, -0.1574803149606299191 ) ) ;
#22004=CARTESIAN_POINT ( 'NONE',  ( 0.1787899950787401882, -0.4297499524812070648, -2.189545951927503898E-17 ) ) ;
#22005=CARTESIAN_POINT ( 'NONE',  ( -0.1643603419142423416, -0.09842519685039370636, -0.06715674897764882523 ) ) ;
#22014=CARTESIAN_POINT ( 'NONE',  ( 0.1264236179284866091, -1.132381889710015743, 0.1264236179284866091 ) ) ;
#22015=CARTESIAN_POINT ( 'NONE',  ( 0.1264236179284866091, -1.314468503883243988, -0.1264236179284866091 ) ) ;
#22022=CARTESIAN_POINT ( 'NONE',  ( -0.06523048226347956391, -0.09891732283464571562, 0.1574803149606297803 ) ) ;
#22028=CARTESIAN_POINT ( 'NONE',  ( -0.1158283541424031532, -0.08956345598586890056, -0.1361971163587911426 ) ) ;
#22029=CARTESIAN_POINT ( 'NONE',  ( 0.1113553986120547346, -0.5147637794200315975, 0.1113553986120547346 ) ) ;
#22037=CARTESIAN_POINT ( 'NONE',  ( -0.07405724077823318263, -1.528543307032852239, 0.1787899950787401604 ) ) ;
#22038=CARTESIAN_POINT ( 'NONE',  ( 0.1113553986120547346, -1.577755905404283343, 0.1113553986120547346 ) ) ;
#22039=CARTESIAN_POINT ( 'NONE',  ( 0.07405724077823318263, -0.6870078739619840391, -0.1787899950787401604 ) ) ;
#22041=CARTESIAN_POINT ( 'NONE',  ( -0.06523048226347956391, -1.058562992125983149, -0.1574803149606300301 ) ) ;
#22050=CARTESIAN_POINT ( 'NONE',  ( -9.642888182262618425E-18, -1.326771653435779408, -0.1574803149606299191 ) ) ;
#22056=CARTESIAN_POINT ( 'NONE',  ( 0.1574803149606300301, -0.07923228335703978720, 0.06523048226347956391 ) ) ;
#22067=VERTEX_POINT ( 'NONE', #4632 ) ;
#22072=CARTESIAN_POINT ( 'NONE',  ( -0.1787899950787401604, -0.8690944881352120621, -0.07405724077823318263 ) ) ;
#22078=CARTESIAN_POINT ( 'NONE',  ( 0.1270800023317771588, -0.2520123135200535436, -0.1270800023317771588 ) ) ;
#22079=CARTESIAN_POINT ( 'NONE',  ( -0.1787899950787401604, -0.1763050705914436245, -0.07405724077823318263 ) ) ;
#22080=CARTESIAN_POINT ( 'NONE',  ( -0.1264236179284866091, -0.04970472435568527164, -0.1264236179284866091 ) ) ;
#22091=CARTESIAN_POINT ( 'NONE',  ( -0.07405724077823318263, -0.3523622046706461619, 0.1787899950787401604 ) ) ;
#22093=CARTESIAN_POINT ( 'NONE',  ( -1.094772975963752103E-17, -1.033956692859621995, -0.1787899950787401882 ) ) ;
#22095=CARTESIAN_POINT ( 'NONE',  ( 0.2471922904502826812, -0.03219022224904106305, 0.1427165354330708902 ) ) ;
#22113=CARTESIAN_POINT ( 'NONE',  ( -0.1787899950787401604, 0.03641732288840918152, 0.07405724077823318263 ) ) ;
#22121=CARTESIAN_POINT ( 'NONE',  ( -0.1787899950787401604, -1.234375936733175916, 0.07405724077823318263 ) ) ;
#22123=CARTESIAN_POINT ( 'NONE',  ( 0.07405724077823318263, -0.2490157479777327099, -0.1787899950787401604 ) ) ;
#22125=CARTESIAN_POINT ( 'NONE',  ( -9.642888182262618425E-18, 0.01181102372957427288, -0.1574803149606299191 ) ) ;
#22133=CARTESIAN_POINT ( 'NONE',  ( -0.1264236179284866091, -1.624507873961984261, -0.1264236179284866091 ) ) ;
#22138=CARTESIAN_POINT ( 'NONE',  ( -0.1797182628040039087, -1.494630423756273085, 0.07444174185955065859 ) ) ;
#22143=CARTESIAN_POINT ( 'NONE',  ( -0.006597203818611992697, 0.1299212598425198428, 0.1741786893156897775 ) ) ;
#22158=CARTESIAN_POINT ( 'NONE',  ( -0.07405724077823318263, -0.2047244093950554844, -0.1787899950787401604 ) ) ;
#22161=CARTESIAN_POINT ( 'NONE',  ( 0.2471922904502826812, -0.03219022224904102836, -0.1427165354330708902 ) ) ;
#22165=CARTESIAN_POINT ( 'NONE',  ( -0.06523048226347956391, 0.1077755906587081480, 0.1574803149606297803 ) ) ;
#22176=CARTESIAN_POINT ( 'NONE',  ( 0.1787899950787401604, -0.8603601887016788519, -0.07405724077823318263 ) ) ;
#22178=AXIS2_PLACEMENT_3D ( 'NONE', #15720, #23837, #38449 ) ;
#22179=CARTESIAN_POINT ( 'NONE',  ( 0.07405724077823318263, 0.1446850394238423654, -0.1787899950787401604 ) ) ;
#22182=ORIENTED_EDGE ( 'NONE', *, *, #32939, .F. ) ;
#22192=CARTESIAN_POINT ( 'NONE',  ( 0.1797182628040039365, -0.9655949906854075504, -2.200913952912460540E-17 ) ) ;
#22203=CARTESIAN_POINT ( 'NONE',  ( -0.1574803149606297803, -0.6845472439869605408, 0.06523048226347956391 ) ) ;
#22206=CARTESIAN_POINT ( 'NONE',  ( -0.07405724077823318263, -0.7017716534895438452, 0.1787899950787401604 ) ) ;
#22212=CARTESIAN_POINT ( 'NONE',  ( -0.06523048226347956391, -1.649114173228347413, -0.1574803149606300301 ) ) ;
#22226=CARTESIAN_POINT ( 'NONE',  ( 0.05275482926409180012, 0.07559918600399875843, -0.2549750559894655155 ) ) ;
#22228=CARTESIAN_POINT ( 'NONE',  ( -0.1264236179284866091, -0.4051436532686086833, 0.1264236179284866091 ) ) ;
#22229=CARTESIAN_POINT ( 'NONE',  ( -0.2247554567094850464, -0.08955974650949173610, -0.08956146268411240008 ) ) ;
#22242=CARTESIAN_POINT ( 'NONE',  ( -0.1264236179284866091, -1.299704724355684959, 0.1264236179284866091 ) ) ;
#22243=CARTESIAN_POINT ( 'NONE',  ( -0.1787899950787401882, -1.614665354276944909, 0.000000000000000000 ) ) ;
#22246=CARTESIAN_POINT ( 'NONE',  ( 0.1270800023317771588, -0.6161855418665097561, 0.1270800023317771588 ) ) ;
#22251=CARTESIAN_POINT ( 'NONE',  ( -0.1574803149606299191, -0.2637795275590551491, 0.000000000000000000 ) ) ;
#22259=CARTESIAN_POINT ( 'NONE',  ( -0.1796295154119676718, -0.08412760742784908263, -0.1817225848796409637 ) ) ;
#22264=CARTESIAN_POINT ( 'NONE',  ( 0.1264236179284866091, -1.599901574749385880, 0.1264236179284866091 ) ) ;
#22265=CARTESIAN_POINT ( 'NONE',  ( -0.1787899950787401882, -0.7140748030958424808, 0.000000000000000000 ) ) ;
#22267=CARTESIAN_POINT ( 'NONE',  ( -0.06523048226347956391, -1.216043307086613012, -0.1574803149606300301 ) ) ;
#22293=CARTESIAN_POINT ( 'NONE',  ( -0.1400282309210590381, -0.09851383267563169899, 0.09116504983989133504 ) ) ;
#22300=AXIS2_PLACEMENT_3D ( 'NONE', #15741, #27001, #33725 ) ;
#22302=CARTESIAN_POINT ( 'NONE',  ( 0.1264236179284866091, -0.9650590550643465271, -0.1264236179284866091 ) ) ;
#22303=CARTESIAN_POINT ( 'NONE',  ( 0.1264236179284866091, -0.3843503936470239468, 0.1264236179284866091 ) ) ;
#22304=CARTESIAN_POINT ( 'NONE',  ( 0.07405724077823318263, -0.9724409448281265966, 0.1787899950787401604 ) ) ;
#22307=CARTESIAN_POINT ( 'NONE',  ( 3.301370929368692659E-17, -0.1880359355672976407, 0.1797182628040039365 ) ) ;
#22309=CARTESIAN_POINT ( 'NONE',  ( -0.1264236179284866091, -0.1284448818360001965, -0.1264236179284866091 ) ) ;
#22322=CARTESIAN_POINT ( 'NONE',  ( 0.1113553986120547346, -0.9379921258767245362, -0.1113553986120547346 ) ) ;
#22323=CARTESIAN_POINT ( 'NONE',  ( -0.1787899950787401604, -0.2834645668753703052, -0.07405724077823318263 ) ) ;
#22325=CARTESIAN_POINT ( 'NONE',  ( -0.1787899950787401604, -1.061023621993481214, 0.07405724077823318263 ) ) ;
#22333=CARTESIAN_POINT ( 'NONE',  ( 0.1574803149606300301, -1.216043306979087468, -0.06523048226347956391 ) ) ;
#22353=CARTESIAN_POINT ( 'NONE',  ( -0.1264236179284866091, -1.428765700512702796, 0.1264236179284866091 ) ) ;
#22356=CARTESIAN_POINT ( 'NONE',  ( 3.284318927891251994E-17, -0.3449803149068665364, 0.1787899950787401882 ) ) ;
#22360=STYLED_ITEM ( 'NONE', ( #11550 ), #36588 ) ;
#22362=CARTESIAN_POINT ( 'NONE',  ( -0.2471913174571636063, -0.07307272215568164087, 0.08638584879643394776 ) ) ;
#22367=CARTESIAN_POINT ( 'NONE',  ( -0.07405724077823318263, -1.587598425143086800, -0.1787899950787401604 ) ) ;
#22368=CARTESIAN_POINT ( 'NONE',  ( 0.07405724077823318263, -1.745078740103716886, -0.1787899950787401604 ) ) ;
#22373=CARTESIAN_POINT ( 'NONE',  ( 0.07444174185955046430, -1.391283967063361215, -0.1797182628040039087 ) ) ;
#22394=CARTESIAN_POINT ( 'NONE',  ( -0.1797182628040039365, -0.001028061551549484288, 0.000000000000000000 ) ) ;
#22400=CARTESIAN_POINT ( 'NONE',  ( -0.1787899950787401604, -0.1998031495525358359, -0.07405724077823318263 ) ) ;
#22406=CARTESIAN_POINT ( 'NONE',  ( 0.1807077244537487193, -0.08350519546663393022, -0.1811005174359491543 ) ) ;
#22409=CARTESIAN_POINT ( 'NONE',  ( -0.1574803149606297803, 0.06348425207603099196, 0.06523048226347956391 ) ) ;
#22411=( GEOMETRIC_REPRESENTATION_CONTEXT ( 3 ) GLOBAL_UNCERTAINTY_ASSIGNED_CONTEXT ( ( #16866 ) ) GLOBAL_UNIT_ASSIGNED_CONTEXT ( ( #6683, #39509, #10546 ) ) REPRESENTATION_CONTEXT ( 'NONE', 'WORKASPACE' ) ) ;
#22416=DIRECTION ( 'NONE',  ( 0.000000000000000000, 1.000000000000000000, 0.000000000000000000 ) ) ;
#22418=CARTESIAN_POINT ( 'NONE',  ( -0.07405724077823318263, -0.9292578264969543200, -0.1787899950787401604 ) ) ;
#22425=CARTESIAN_POINT ( 'NONE',  ( -0.1787899950787401604, -0.4803149605761579677, -0.07405724077823318263 ) ) ;
#22431=CARTESIAN_POINT ( 'NONE',  ( 0.1797182628040039087, -0.9631343607641484894, -0.07444174185955065859 ) ) ;
#22440=CARTESIAN_POINT ( 'NONE',  ( 0.1113553986120547346, 0.1151574804224878013, 0.1113553986120547346 ) ) ;
#22444=CARTESIAN_POINT ( 'NONE',  ( -0.1264236179284866091, -0.8321850393163149340, -0.1264236179284866091 ) ) ;
#22449=DIRECTION ( 'NONE',  ( 0.000000000000000000, 1.000000000000000000, 0.000000000000000000 ) ) ;
#22450=CARTESIAN_POINT ( 'NONE',  ( 0.1574803149606300301, -1.624507874015748810, 0.06523048226347956391 ) ) ;
#22455=ORIENTED_EDGE ( 'NONE', *, *, #14578, .T. ) ;
#22457=CARTESIAN_POINT ( 'NONE',  ( -9.642888182262618425E-18, -0.3031496061916854612, -0.1574803149606299191 ) ) ;
#22471=CARTESIAN_POINT ( 'NONE',  ( 0.1264236179284866091, -0.4346712123237267966, 0.1264236179284866091 ) ) ;
#22472=CARTESIAN_POINT ( 'NONE',  ( 0.08190613820814231227, -0.09842519685039370636, 0.1253801239223421293 ) ) ;
#22474=DIRECTION ( 'NONE',  ( 0.000000000000000000, 1.000000000000000000, 0.000000000000000000 ) ) ;
#22482=CARTESIAN_POINT ( 'NONE',  ( 0.1264236179284866091, -1.280019684985606254, -0.1264236179284866091 ) ) ;
#22483=CARTESIAN_POINT ( 'NONE',  ( 0.1787899950787401882, -1.555610236166708571, -2.189545951927503898E-17 ) ) ;
#22490=CARTESIAN_POINT ( 'NONE',  ( -0.06523048226347956391, -0.2957677165354329341, 0.1574803149606297803 ) ) ;
#22494=CARTESIAN_POINT ( 'NONE',  ( -0.1158283541424031532, -0.08956345598586890056, -0.1361971163587911426 ) ) ;
#22501=CARTESIAN_POINT ( 'NONE',  ( -0.07885344035849289890, -0.08956334183977000818, 0.1372477332191901489 ) ) ;
#22508=CARTESIAN_POINT ( 'NONE',  ( 0.1264236179284866091, -1.511318897584031484, -0.1264236179284866091 ) ) ;
#22509=CARTESIAN_POINT ( 'NONE',  ( 3.284318927891251994E-17, -0.7042322834108031282, 0.1787899950787401882 ) ) ;
#22510=CARTESIAN_POINT ( 'NONE',  ( -0.1574803149606297803, -1.284940944881890923, 0.06523048226347956391 ) ) ;
#22526=CARTESIAN_POINT ( 'NONE',  ( 0.07600661141694387002, 0.08819060268787905221, 0.2415506333043779541 ) ) ;
#22533=CARTESIAN_POINT ( 'NONE',  ( -0.2118147889498118164, -0.09842519685039370636, 0.1047082926952616067 ) ) ;
#22542=CARTESIAN_POINT ( 'NONE',  ( -0.07405724077823318263, -0.8789370078202529690, -0.1787899950787401604 ) ) ;
#22543=CARTESIAN_POINT ( 'NONE',  ( 3.284318927891251994E-17, -0.4680118109698582773, 0.1787899950787401882 ) ) ;
#22544=CARTESIAN_POINT ( 'NONE',  ( -0.1264236179284866091, -0.9896653542769447975, -0.1264236179284866091 ) ) ;
#22548=CARTESIAN_POINT ( 'NONE',  ( 0.1270800023317771588, -0.3701225497405259968, -0.1270800023317771588 ) ) ;
#22549=CARTESIAN_POINT ( 'NONE',  ( -0.1574803149606297803, 0.1323818897637794312, 0.06523048226347956391 ) ) ;
#22564=CARTESIAN_POINT ( 'NONE',  ( -0.1574803149606299191, -0.9625984250893229177, 0.000000000000000000 ) ) ;
#22565=CARTESIAN_POINT ( 'NONE',  ( 0.1787899950787401604, -0.2637795275052916555, 0.07405724077823318263 ) ) ;
#22568=CARTESIAN_POINT ( 'NONE',  ( 0.1264236179284866091, -1.235728346402928945, -0.1264236179284866091 ) ) ;
#22576=CARTESIAN_POINT ( 'NONE',  ( 0.1574803149606300301, -1.181594488081448846, 0.06523048226347956391 ) ) ;
#22595=B_SPLINE_CURVE_WITH_KNOTS ( 'NONE', 3,
 ( #10234, #6380, #43278, #13362, #28215, #42779 ),
 .UNSPECIFIED., .F., .F.,
 ( 4, 2, 4 ),
 ( 0.000000000000000000, 0.5000000000000000000, 1.000000000000000000 ),
 .UNSPECIFIED. ) ;
#22597=CARTESIAN_POINT ( 'NONE',  ( 0.07405724077823318263, -1.421383810748923393, 0.1787899950787401604 ) ) ;
#22599=CARTESIAN_POINT ( 'NONE',  ( -0.1787899950787401604, -0.3966535432533230265, -0.07405724077823318263 ) ) ;
#22609=CARTESIAN_POINT ( 'NONE',  ( 0.1787899950787401882, -1.757381889710015965, -2.189545951927503898E-17 ) ) ;
#22610=CARTESIAN_POINT ( 'NONE',  ( 3.284318927891251994E-17, -1.644192913332062966, 0.1787899950787401882 ) ) ;
#22616=CARTESIAN_POINT ( 'NONE',  ( 0.1113553986120547346, -0.8001968503937008093, 0.1113553986120547346 ) ) ;
#22618=CARTESIAN_POINT ( 'NONE',  ( 0.07444174185955065859, -1.445417825331076767, 0.1797182628040039087 ) ) ;
#22619=DIRECTION ( 'NONE',  ( 0.000000000000000000, 1.000000000000000000, 0.000000000000000000 ) ) ;
#22620=CARTESIAN_POINT ( 'NONE',  ( 0.2471922904502826812, 0.09842519685039370636, -5.914624404477007554E-17 ) ) ;
#22641=CARTESIAN_POINT ( 'NONE',  ( 3.301370929368692659E-17, -0.06992569934682500710, 0.1797182628040039365 ) ) ;
#22644=CARTESIAN_POINT ( 'NONE',  ( 0.1264236179284866091, -1.201279527505291433, -0.1264236179284866091 ) ) ;
#22651=CARTESIAN_POINT ( 'NONE',  ( 0.1787899950787401882, -0.1382874015210395768, -2.189545951927503898E-17 ) ) ;
#22656=CARTESIAN_POINT ( 'NONE',  ( 0.1113553986120547346, -0.1112204723334179052, -0.1113553986120547346 ) ) ;
#22663=CARTESIAN_POINT ( 'NONE',  ( 0.1787899950787401882, -1.020301133583568776, -2.189545951927503898E-17 ) ) ;
#22665=CARTESIAN_POINT ( 'NONE',  ( 3.284318927891251994E-17, 0.08809055123486594918, 0.1787899950787401882 ) ) ;
#22666=VERTEX_POINT ( 'NONE', #22095 ) ;
#22671=CARTESIAN_POINT ( 'NONE',  ( 0.1787899950787401604, -0.4950787401037172186, -0.07405724077823318263 ) ) ;
#22676=CARTESIAN_POINT ( 'NONE',  ( 0.1270800023317771588, -1.000043809583045284, -0.1270800023317771588 ) ) ;
#22683=CARTESIAN_POINT ( 'NONE',  ( 0.1574803149606299191, 0.1200787401574803237, 2.850509043694854679E-09 ) ) ;
#22688=CARTESIAN_POINT ( 'NONE',  ( 0.1264236179284866091, -0.7337598424659212970, 0.1264236179284866091 ) ) ;
#22694=CARTESIAN_POINT ( 'NONE',  ( 0.1574803149606300301, -1.698326771653543510, -0.06523048226347956391 ) ) ;
#22701=CARTESIAN_POINT ( 'NONE',  ( 0.1264236179284866091, -1.486712598371433103, 0.1264236179284866091 ) ) ;
#22708=CARTESIAN_POINT ( 'NONE',  ( 0.1380782811756038342, 0.1289404906632452552, -0.09318370980563837891 ) ) ;
#22711=CARTESIAN_POINT ( 'NONE',  ( -0.07405724077823318263, -0.5355570390953806603, -0.1787899950787401604 ) ) ;
#22712=CARTESIAN_POINT ( 'NONE',  ( -0.002407869453279200614, -0.08955980254238483929, 0.2209030018291311126 ) ) ;
#22717=CARTESIAN_POINT ( 'NONE',  ( 0.2471915046495881119, -0.08339338023400436062, 0.06619788746988974903 ) ) ;
#22722=CARTESIAN_POINT ( 'NONE',  ( -0.07405724077823318263, -1.336614173174582865, 0.1787899950787401604 ) ) ;
#22723=CARTESIAN_POINT ( 'NONE',  ( -0.07405724077823318263, -1.567913385773008095, 0.1787899950787401604 ) ) ;
#22733=CARTESIAN_POINT ( 'NONE',  ( -0.1574803149606299191, -0.3031496062992126150, 0.000000000000000000 ) ) ;
#22742=CARTESIAN_POINT ( 'NONE',  ( -0.1677420379284152441, -0.08956119648846384840, 0.01551656620580007390 ) ) ;
#22743=ORIENTED_EDGE ( 'NONE', *, *, #20943, .T. ) ;
#22746=CARTESIAN_POINT ( 'NONE',  ( -0.1179171413540952840, 0.09842519685039383126, -0.2173535775632838007 ) ) ;
#22748=CARTESIAN_POINT ( 'NONE',  ( 0.1264236179284866091, -1.521161417269070837, 0.1264236179284866091 ) ) ;
#22749=CARTESIAN_POINT ( 'NONE',  ( -0.1787899950787401882, -0.8321850393163149340, 0.000000000000000000 ) ) ;
#22750=CARTESIAN_POINT ( 'NONE',  ( -0.1574803149606297803, -1.206200787401574770, 0.06523048226347956391 ) ) ;
#22771=CARTESIAN_POINT ( 'NONE',  ( -0.2160651621502015785, -0.09842519685039370636, -0.1192374171493116308 ) ) ;
#22781=CARTESIAN_POINT ( 'NONE',  ( -0.1787899950787401604, -0.8297244093950564281, 0.07405724077823318263 ) ) ;
#22782=CARTESIAN_POINT ( 'NONE',  ( -0.1787899950787401604, -1.065944881836000224, -0.07405724077823318263 ) ) ;
#22787=CARTESIAN_POINT ( 'NONE',  ( 0.07444174185955065859, -0.3430556206066676106, 0.1797182628040039087 ) ) ;
#22788=CARTESIAN_POINT ( 'NONE',  ( -0.1574803149606300301, 0.08809055118110237226, -0.06523048226347956391 ) ) ;
#22789=CARTESIAN_POINT ( 'NONE',  ( 3.284318927891251994E-17, -0.1530511810485986057, 0.1787899950787401882 ) ) ;
#22794=PLANE ( 'NONE',  #17752 ) ;
#22799=CARTESIAN_POINT ( 'NONE',  ( -1.094772975963752103E-17, -0.2121062991588350544, -0.1787899950787401882 ) ) ;
#22801=CARTESIAN_POINT ( 'NONE',  ( -0.1264236179284866091, -1.225885826717889815, -0.1264236179284866091 ) ) ;
#22823=CARTESIAN_POINT ( 'NONE',  ( -0.2246256911002503798, -0.09851385142897184366, -0.1004183578296887897 ) ) ;
#22831=CARTESIAN_POINT ( 'NONE',  ( 0.1787899950787401882, -1.492742078465458810, -2.189545951927503898E-17 ) ) ;
#22834=CARTESIAN_POINT ( 'NONE',  ( 0.07405724077823318263, -0.4852362204186770889, -0.1787899950787401604 ) ) ;
#22845=CARTESIAN_POINT ( 'NONE',  ( -0.1787899950787401604, -1.735236220418678643, 0.07405724077823318263 ) ) ;
#22846=CARTESIAN_POINT ( 'NONE',  ( -0.1264236179284866091, -1.737696850339937038, -0.1264236179284866091 ) ) ;
#22851=CARTESIAN_POINT ( 'NONE',  ( -0.1574803149606300301, -0.6993110236220480003, -0.06523048226347956391 ) ) ;
#22852=CARTESIAN_POINT ( 'NONE',  ( 0.1270800023317771588, -1.403587116669659407, 0.1270800023317771588 ) ) ;
#22877=CARTESIAN_POINT ( 'NONE',  ( 0.1270800023317771588, 0.01373571797600956802, 0.1270800023317771588 ) ) ;
#22878=CARTESIAN_POINT ( 'NONE',  ( -0.1264236179284866091, -1.181594488135212506, 0.1264236179284866091 ) ) ;
#22879=DIRECTION ( 'NONE',  ( 0.000000000000000000, 1.000000000000000000, 0.000000000000000000 ) ) ;
#22882=CARTESIAN_POINT ( 'NONE',  ( -0.06523048226347956391, 0.04379921259842517456, -0.1574803149606300301 ) ) ;
#22886=CARTESIAN_POINT ( 'NONE',  ( -0.03837864586579538273, -0.06712557525760225186, -0.2632749781601607109 ) ) ;
#22890=CARTESIAN_POINT ( 'NONE',  ( 0.1113553986120547346, -0.03248031485310291788, -0.1113553986120547346 ) ) ;
#22898=CARTESIAN_POINT ( 'NONE',  ( 0.1787899950787401604, -0.9391003461819946718, -0.07405724077823318263 ) ) ;
#22907=CARTESIAN_POINT ( 'NONE',  ( 0.1787899950787401882, -0.5369094487651339120, -2.189545951927503898E-17 ) ) ;
#22910=CARTESIAN_POINT ( 'NONE',  ( -0.1797182628040039365, -0.9459099513153288452, 0.000000000000000000 ) ) ;
#22923=CARTESIAN_POINT ( 'NONE',  ( -0.1787899950787401882, -0.7878937007336378473, 0.000000000000000000 ) ) ;
#22929=CARTESIAN_POINT ( 'NONE',  ( 0.06523048226347956391, -1.604822834538142784, -0.1574803149606300301 ) ) ;
#22933=CARTESIAN_POINT ( 'NONE',  ( 0.1574803149606299191, -1.700787401574803237, -1.928577636452523993E-17 ) ) ;
#22942=CARTESIAN_POINT ( 'NONE',  ( 0.1574803149606300301, -0.3499015746956224415, -0.06523048226347956391 ) ) ;
#22943=CARTESIAN_POINT ( 'NONE',  ( -0.1787899950787401882, -1.580216535379306952, 0.000000000000000000 ) ) ;
#22949=DIRECTION ( 'NONE',  ( 0.000000000000000000, 0.000000000000000000, 1.000000000000000000 ) ) ;
#22952=CARTESIAN_POINT ( 'NONE',  ( 0.07405724077823318263, -0.6192184564182152684, -0.1787899950787401604 ) ) ;
#22953=CARTESIAN_POINT ( 'NONE',  ( 0.07190187720976377872, -0.08956013875575118133, 0.2047185321618893994 ) ) ;
#22957=CARTESIAN_POINT ( 'NONE',  ( 0.000000000000000000, -0.09842519685039370636, 0.000000000000000000 ) ) ;
#22959=CARTESIAN_POINT ( 'NONE',  ( 2.892866454678787531E-17, -0.007874015640504449659, 0.1574803149606299191 ) ) ;
#22964=CARTESIAN_POINT ( 'NONE',  ( -0.07405724077823318263, -1.272637795221826629, -0.1787899950787401604 ) ) ;
#22965=CARTESIAN_POINT ( 'NONE',  ( 0.1787899950787401604, -1.474409448765133801, -0.07405724077823318263 ) ) ;
#22972=CARTESIAN_POINT ( 'NONE',  ( -0.1113553986120547346, -0.2588582677165354173, 0.1113553986120547346 ) ) ;
#22979=CARTESIAN_POINT ( 'NONE',  ( 0.1574803149606300301, -0.5467519683964097155, -0.06523048226347956391 ) ) ;
#22980=CARTESIAN_POINT ( 'NONE',  ( -0.1564674760227699191, -0.09340956239926194449, 0.1950964973271945568 ) ) ;
#22982=CARTESIAN_POINT ( 'NONE',  ( -0.1288387865083106543, -0.08955301800084583541, 0.09875942480506787191 ) ) ;
#22990=CARTESIAN_POINT ( 'NONE',  ( -0.1264236179284866091, -1.658956692859621995, -0.1264236179284866091 ) ) ;
#22991=CARTESIAN_POINT ( 'NONE',  ( -0.1787899950787401604, -0.8690944881352120621, 0.07405724077823318263 ) ) ;
#22992=CARTESIAN_POINT ( 'NONE',  ( 0.1113553986120547346, -1.223425196850393748, -0.1113553986120547346 ) ) ;
#23015=CARTESIAN_POINT ( 'NONE',  ( -0.1946994858204661449, -0.09842519685039370636, -0.1548548131872939104 ) ) ;
#23018=ORIENTED_EDGE ( 'NONE', *, *, #17008, .F. ) ;
#23021=VERTEX_POINT ( 'NONE', #46538 ) ;
#23023=CARTESIAN_POINT ( 'NONE',  ( -0.1264236179284866091, -0.9552165353793071745, -0.1264236179284866091 ) ) ;
#23024=CARTESIAN_POINT ( 'NONE',  ( -0.1264236179284866091, -1.068405511757259951, -0.1264236179284866091 ) ) ;
#23028=CARTESIAN_POINT ( 'NONE',  ( -0.1797182628040039087, -0.2790792426539118187, -0.07444174185955065859 ) ) ;
#23029=CARTESIAN_POINT ( 'NONE',  ( 0.1113553986120547346, 0.1151574803149606335, -0.1113553986120547346 ) ) ;
#23040=CARTESIAN_POINT ( 'NONE',  ( -0.1264236179284866091, -0.4335629920722205433, 0.1264236179284866091 ) ) ;
#23042=CARTESIAN_POINT ( 'NONE',  ( 0.07405724077823318263, -1.208661417269070393, 0.1787899950787401604 ) ) ;
#23049=CARTESIAN_POINT ( 'NONE',  ( 0.1113553986120547346, -1.184055118002708795, 0.1113553986120547346 ) ) ;
#23053=CARTESIAN_POINT ( 'NONE',  ( 0.04026256913104946100, -0.09842715401333676506, -0.1741995584308680955 ) ) ;
#23059=VECTOR ( 'NONE', #16393, 39.37007874015748143 ) ;
#23075=CARTESIAN_POINT ( 'NONE',  ( -0.1264236179284866091, -1.517348377678057192, -0.1264236179284866091 ) ) ;
#23077=CARTESIAN_POINT ( 'NONE',  ( 3.284318927891251994E-17, -0.4237204723871811352, 0.1787899950787401882 ) ) ;
#23083=CARTESIAN_POINT ( 'NONE',  ( 0.07405724077823318263, -1.725393700733637958, 0.1787899950787401604 ) ) ;
#23084=CARTESIAN_POINT ( 'NONE',  ( 0.1264236179284866091, 0.1274606299750234428, 0.1264236179284866091 ) ) ;
#23089=CARTESIAN_POINT ( 'NONE',  ( 0.1113553986120547346, -0.7214566929133858775, 0.1113553986120547346 ) ) ;
#23090=CARTESIAN_POINT ( 'NONE',  ( 0.07444174185955046430, -1.470024124543674926, -0.1797182628040039087 ) ) ;
#23092=CARTESIAN_POINT ( 'NONE',  ( -0.1113553986120547346, -0.4458661416247566289, 0.1113553986120547346 ) ) ;
#23093=CARTESIAN_POINT ( 'NONE',  ( 0.2471922904502825702, 0.06774690380563494485, -0.09545378441111782020 ) ) ;
#23105=CARTESIAN_POINT ( 'NONE',  ( -0.06523048226347956391, -0.8371062991050713942, 0.1574803149606297803 ) ) ;
#23106=CARTESIAN_POINT ( 'NONE',  ( 3.284318927891251994E-17, -0.03494094482812622193, 0.1787899950787401882 ) ) ;
#23119=CARTESIAN_POINT ( 'NONE',  ( 0.1797182628040039087, -0.02317373084288805798, 0.07444174185955046430 ) ) ;
#23120=CARTESIAN_POINT ( 'NONE',  ( 0.1787899950787401604, -1.203740157426551383, -0.07405724077823318263 ) ) ;
#23131=CARTESIAN_POINT ( 'NONE',  ( -0.1574803149606300301, 0.01919291349335381161, -0.06523048226347956391 ) ) ;
#23139=CARTESIAN_POINT ( 'NONE',  ( 0.1787899950787401604, -1.062131842244986135, 0.07405724077823318263 ) ) ;
#23141=CARTESIAN_POINT ( 'NONE',  ( -0.1787899950787401882, -0.0004921259304884630223, 0.000000000000000000 ) ) ;
#23148=CARTESIAN_POINT ( 'NONE',  ( -0.1787899950787401882, -0.5959645668753701386, 0.000000000000000000 ) ) ;
#23153=CARTESIAN_POINT ( 'NONE',  ( -0.1270800023317771588, -1.019728848953123990, 0.1270800023317771588 ) ) ;
#23161=CARTESIAN_POINT ( 'NONE',  ( 0.1574803149606299191, -0.6673228345381416737, -1.928577636452523993E-17 ) ) ;
#23163=AXIS2_PLACEMENT_3D ( 'NONE', #31974, #38907, #13983 ) ;
#23168=CARTESIAN_POINT ( 'NONE',  ( -0.1264236179284866091, -0.9798228345919054449, 0.1264236179284866091 ) ) ;
#23170=DIRECTION ( 'NONE',  ( 0.000000000000000000, 0.000000000000000000, 1.000000000000000000 ) ) ;
#23173=CARTESIAN_POINT ( 'NONE',  ( -0.06523048226347956391, -1.757381889656251195, -0.1574803149606300301 ) ) ;
#23175=CARTESIAN_POINT ( 'NONE',  ( -0.1264236179284866091, -0.08415354325332302654, -0.1264236179284866091 ) ) ;
#23179=CARTESIAN_POINT ( 'NONE',  ( -0.1113553986120547346, -1.686023622047244208, -0.1113553986120547346 ) ) ;
#23187=CARTESIAN_POINT ( 'NONE',  ( 0.1787899950787401604, -1.523622047190330564, 0.07405724077823318263 ) ) ;
#23195=CARTESIAN_POINT ( 'NONE',  ( 0.1264236179284866091, -0.6216790863394745514, -0.1264236179284866091 ) ) ;
#23196=CARTESIAN_POINT ( 'NONE',  ( 0.06715823863710629338, -0.08956012741285963863, 0.2065986400649870158 ) ) ;
#23207=CARTESIAN_POINT ( 'NONE',  ( 3.284318927891251994E-17, -1.373523621993480326, 0.1787899950787401882 ) ) ;
#23208=CARTESIAN_POINT ( 'NONE',  ( -0.07405724077823318263, -1.503937007820251637, -0.1787899950787401604 ) ) ;
#23210=VECTOR ( 'NONE', #7019, 39.37007874015748143 ) ;
#23218=CARTESIAN_POINT ( 'NONE',  ( 0.1574803149606300301, -0.2859251968503936370, 0.06523048226347956391 ) ) ;
#23226=CARTESIAN_POINT ( 'NONE',  ( 0.06523048226347956391, -0.5565944880814488460, 0.1574803149606297803 ) ) ;
#23231=CARTESIAN_POINT ( 'NONE',  ( -0.1264236179284866091, -0.5467519684501732646, 0.1264236179284866091 ) ) ;
#23238=CARTESIAN_POINT ( 'NONE',  ( -0.09934514972680209832, 0.09575019180979019162, -0.2280761219286889518 ) ) ;
#23239=CARTESIAN_POINT ( 'NONE',  ( 0.07405724077823318263, -1.745078740103716886, -0.1787899950787401604 ) ) ;
#23240=CARTESIAN_POINT ( 'NONE',  ( 0.07405724077823318263, -0.8592519684501739308, 0.1787899950787401604 ) ) ;
#23241=CARTESIAN_POINT ( 'NONE',  ( 0.1574803149606299191, -1.188976377952756014, -1.928577636452523993E-17 ) ) ;
#23248=EDGE_LOOP ( 'NONE', ( #133, #7539, #23386, #14518, #27857, #29840, #26490, #23584, #373, #41503, #1594, #21980, #46030, #24589, #7686, #14281, #20640 ) ) ;
#23262=CARTESIAN_POINT ( 'NONE',  ( -0.004818628365293897708, -0.09851383159603781248, 0.1563573961146315083 ) ) ;
#23267=CARTESIAN_POINT ( 'NONE',  ( 0.1264236179284866091, -0.8567913385289133155, 0.1264236179284866091 ) ) ;
#23268=CARTESIAN_POINT ( 'NONE',  ( 0.1264236179284866091, -1.127460629867496067, 0.1264236179284866091 ) ) ;
#23270=CARTESIAN_POINT ( 'NONE',  ( -0.1270800023317771588, -0.3602800300554865887, -0.1270800023317771588 ) ) ;
#23271=CARTESIAN_POINT ( 'NONE',  ( 0.06523048226347956391, -1.801673228238930946, -0.1574803149606300301 ) ) ;
#23274=CARTESIAN_POINT ( 'NONE',  ( -0.1787899950787401604, -0.1604330708123782034, 0.07405724077823318263 ) ) ;
#23286=CARTESIAN_POINT ( 'NONE',  ( -0.07405724077823318263, -0.4704724408911186706, 0.1787899950787401604 ) ) ;
#23288=CARTESIAN_POINT ( 'NONE',  ( 0.1787899950787401604, -1.282480314906867314, 0.07405724077823318263 ) ) ;
#23297=CARTESIAN_POINT ( 'NONE',  ( 0.06597690942901487943, -0.09842519659738405147, -0.1661715391456292656 ) ) ;
#23310=EDGE_LOOP ( 'NONE', ( #40471, #31354, #31650 ) ) ;
#23316=CARTESIAN_POINT ( 'NONE',  ( -0.1264236179284866091, -1.507505857993017839, 0.1264236179284866091 ) ) ;
#23320=CARTESIAN_POINT ( 'NONE',  ( -0.1787899950787401604, -0.4311023621509605386, 0.07405724077823318263 ) ) ;
#23324=CARTESIAN_POINT ( 'NONE',  ( 0.07405724077823318263, -0.2293307086076536994, 0.1787899950787401604 ) ) ;
#23329=CARTESIAN_POINT ( 'NONE',  ( -0.1264236179284866091, -1.742618110182456714, -0.1264236179284866091 ) ) ;
#23330=CARTESIAN_POINT ( 'NONE',  ( -0.07405724077823318263, 0.1446850394238423654, -0.1787899950787401604 ) ) ;
#23336=CARTESIAN_POINT ( 'NONE',  ( 0.1574803149606300301, -0.7583661417322827836, 0.06523048226347956391 ) ) ;
#23338=CARTESIAN_POINT ( 'NONE',  ( 0.1797182628040039365, -1.516776093047611962, -2.200913952912460540E-17 ) ) ;
#23339=CARTESIAN_POINT ( 'NONE',  ( 0.000000000000000000, 0.1299212598425196763, 0.000000000000000000 ) ) ;
#23340=CARTESIAN_POINT ( 'NONE',  ( 0.1574803149606300301, -0.4729330707586144600, 0.06523048226347956391 ) ) ;
#23349=CARTESIAN_POINT ( 'NONE',  ( -0.07405724077823318263, 0.06594488194352733645, -0.1787899950787401604 ) ) ;
#23358=CARTESIAN_POINT ( 'NONE',  ( 2.892866454678787531E-17, -0.05708661417322834220, 0.1574803149606299191 ) ) ;
#23360=CARTESIAN_POINT ( 'NONE',  ( 0.1574803149606299191, -1.061023621939716666, -1.928577636452523993E-17 ) ) ;
#23373=CARTESIAN_POINT ( 'NONE',  ( -0.09216094027006721534, -0.09383642490574109485, -0.2322237458740071259 ) ) ;
#23377=CARTESIAN_POINT ( 'NONE',  ( -0.1574803149606297803, 0.02411417333587350179, 0.06523048226347956391 ) ) ;
#23385=CARTESIAN_POINT ( 'NONE',  ( -0.07405724077823318263, -0.9686279052371123965, -0.1787899950787401604 ) ) ;
#23386=ORIENTED_EDGE ( 'NONE', *, *, #41505, .F. ) ;
#23387=CARTESIAN_POINT ( 'NONE',  ( -0.1787899950787401604, 0.03641732288840918152, -0.07405724077823318263 ) ) ;
#23393=CARTESIAN_POINT ( 'NONE',  ( 0.1787899950787401604, -0.5738188975840317063, -0.07405724077823318263 ) ) ;
#23397=CARTESIAN_POINT ( 'NONE',  ( -0.07444174185955065859, -1.135378455252336050, 0.1797182628040039087 ) ) ;
#23407=CARTESIAN_POINT ( 'NONE',  ( 0.07405724077823318263, 0.05118110241596821042, 0.1787899950787401604 ) ) ;
#23412=ORIENTED_EDGE ( 'NONE', *, *, #19965, .F. ) ;
#23417=CARTESIAN_POINT ( 'NONE',  ( -0.1574803149606297803, -1.747539369971212730, 0.06523048226347956391 ) ) ;
#23422=CARTESIAN_POINT ( 'NONE',  ( 0.1787899950787401604, 0.1348425197388028463, 0.07405724077823318263 ) ) ;
#23427=CARTESIAN_POINT ( 'NONE',  ( -0.07405724077823318263, -1.612204724355685403, 0.1787899950787401604 ) ) ;
#23432=CARTESIAN_POINT ( 'NONE',  ( -0.1787899950787401882, -0.4888050705914433469, 0.000000000000000000 ) ) ;
#23433=CARTESIAN_POINT ( 'NONE',  ( 0.1747654535727043434, -0.08956020295265729181, 0.1168153130661813005 ) ) ;
#23440=CARTESIAN_POINT ( 'NONE',  ( -0.1264236179284866091, -1.783096409174122154, 0.1264236179284866091 ) ) ;
#23443=CARTESIAN_POINT ( 'NONE',  ( 0.2471920549079764384, -0.08080427097405437631, 0.07167403547456246971 ) ) ;
#23448=CARTESIAN_POINT ( 'NONE',  ( -0.1787899950787401604, -1.464566929080096225, -0.07405724077823318263 ) ) ;
#23458=CARTESIAN_POINT ( 'NONE',  ( -0.06523048226347956391, -0.3892716535433071168, -0.1574803149606300301 ) ) ;
#23467=CARTESIAN_POINT ( 'NONE',  ( 0.06523048226347956391, -0.5418307085538903722, -0.1574803149606300301 ) ) ;
#23471=CARTESIAN_POINT ( 'NONE',  ( -0.1656966359942823597, -0.08956191954329044413, 0.02636594708157497663 ) ) ;
#23472=CARTESIAN_POINT ( 'NONE',  ( -0.1787899950787401604, -0.5885826771115909573, 0.07405724077823318263 ) ) ;
#23479=CARTESIAN_POINT ( 'NONE',  ( -0.09432024557781878982, 0.09445537554013626325, -0.2309772516917564245 ) ) ;
#23481=CARTESIAN_POINT ( 'NONE',  ( -0.1787899950787401882, -1.693405511757259951, 0.000000000000000000 ) ) ;
#23482=CARTESIAN_POINT ( 'NONE',  ( 0.1787899950787401604, -0.9281496062454495100, -0.07405724077823318263 ) ) ;
#23483=CARTESIAN_POINT ( 'NONE',  ( 2.892866454678787531E-17, -1.356299212598425230, 0.1574803149606299191 ) ) ;
#23503=CARTESIAN_POINT ( 'NONE',  ( 0.2009854772848184978, -0.09842519685039370636, -0.04150255699268778908 ) ) ;
#23512=CARTESIAN_POINT ( 'NONE',  ( 3.284318927891251994E-17, -0.9798228345919054449, 0.1787899950787401882 ) ) ;
#23513=CARTESIAN_POINT ( 'NONE',  ( -0.07405724077823318263, -1.031496062938363822, -0.1787899950787401604 ) ) ;
#23517=CARTESIAN_POINT ( 'NONE',  ( 0.1797182628040039087, -0.4168745182444627551, 0.07444174185955046430 ) ) ;
#23519=CARTESIAN_POINT ( 'NONE',  ( -9.642888182262618425E-18, -0.03740157480314960925, -0.1574803149606299191 ) ) ;
#23526=CARTESIAN_POINT ( 'NONE',  ( -0.1264236179284866091, -0.4827755904974173617, -0.1264236179284866091 ) ) ;
#23528=ADVANCED_FACE ( 'NONE', ( #34966 ), #5575, .T. ) ;
#23529=CARTESIAN_POINT ( 'NONE',  ( 0.1787899950787401882, -1.280019684985606254, -2.189545951927503898E-17 ) ) ;
#23538=CARTESIAN_POINT ( 'NONE',  ( 0.06305891922640385894, -0.09842519065806150380, -0.1673058913905094147 ) ) ;
#23543=CARTESIAN_POINT ( 'NONE',  ( 0.06523048226347956391, -0.09399606299212612259, 0.1574803149606297803 ) ) ;
#23546=CARTESIAN_POINT ( 'NONE',  ( -0.1602258124790746086, -0.09851385344451535353, -0.1931672967797941065 ) ) ;
#23553=CARTESIAN_POINT ( 'NONE',  ( 0.1787899950787401604, -0.3720472440407247561, -0.07405724077823318263 ) ) ;
#23559=CARTESIAN_POINT ( 'NONE',  ( -0.07405724077823318263, -0.2490157479777327099, -0.1787899950787401604 ) ) ;
#23562=CARTESIAN_POINT ( 'NONE',  ( -1.094772975963752103E-17, -1.708169291284818980, -0.1787899950787401882 ) ) ;
#23563=CARTESIAN_POINT ( 'NONE',  ( 0.1243106777423573922, -0.09842519685039372024, 0.1163740807232158392 ) ) ;
#23565=CARTESIAN_POINT ( 'NONE',  ( 2.892866454678787531E-17, -0.7263779527559055538, 0.1574803149606299191 ) ) ;
#23567=CARTESIAN_POINT ( 'NONE',  ( 3.301370929368692659E-17, -1.605358770212966357, 0.1797182628040039365 ) ) ;
#23568=DIRECTION ( 'NONE',  ( 0.000000000000000000, 1.000000000000000000, 0.000000000000000000 ) ) ;
#23569=CARTESIAN_POINT ( 'NONE',  ( 3.284318927891251994E-17, -0.3843503936470239468, 0.1787899950787401882 ) ) ;
#23570=CARTESIAN_POINT ( 'NONE',  ( 0.2471922904502826535, 0.07794254751779122747, -0.07737183577689113467 ) ) ;
#23577=CARTESIAN_POINT ( 'NONE',  ( 0.1787899950787401604, 0.05118110241596821736, 0.07405724077823318263 ) ) ;
#23584=ORIENTED_EDGE ( 'NONE', *, *, #15216, .F. ) ;
#23586=EDGE_LOOP ( 'NONE', ( #7098, #38392, #42845 ) ) ;
#23602=CARTESIAN_POINT ( 'NONE',  ( 0.1574803149606300301, -0.07431102351452013866, -0.06523048226347956391 ) ) ;
#23609=CARTESIAN_POINT ( 'NONE',  ( 0.1787899950787401604, -1.096580661142624757, -0.07405724077823318263 ) ) ;
#23611=CARTESIAN_POINT ( 'NONE',  ( 3.284318927891251994E-17, 0.009350393754550925460, 0.1787899950787401882 ) ) ;
#23620=CARTESIAN_POINT ( 'NONE',  ( 0.1787899950787401882, -0.6156496062454488438, -2.189545951927503898E-17 ) ) ;
#23625=CARTESIAN_POINT ( 'NONE',  ( -0.1797182628040039365, -1.142760345016116119, 0.000000000000000000 ) ) ;
#23629=DIRECTION ( 'NONE',  ( 0.000000000000000000, 0.000000000000000000, 1.000000000000000000 ) ) ;
#23640=CARTESIAN_POINT ( 'NONE',  ( 0.1113553986120547346, -1.646653543199559033, -0.1113553986120547346 ) ) ;
#23646=CARTESIAN_POINT ( 'NONE',  ( 0.01960094289354776670, -0.05179116514259233389, 0.2741164612101792963 ) ) ;
#23647=CARTESIAN_POINT ( 'NONE',  ( 0.1574803149606300301, -1.777066929133858109, -0.06523048226347956391 ) ) ;
#23652=CARTESIAN_POINT ( 'NONE',  ( -0.05635946233522095422, 0.07780450164205261754, 0.2528939201155192551 ) ) ;
#23655=CARTESIAN_POINT ( 'NONE',  ( -0.1787899950787401604, -1.577755905458046115, 0.07405724077823318263 ) ) ;
#23665=CARTESIAN_POINT ( 'NONE',  ( -0.1264236179284866091, -0.6019940469693956242, 0.1264236179284866091 ) ) ;
#23666=CARTESIAN_POINT ( 'NONE',  ( -0.1316538794915708688, -0.08956060683158523217, -0.1194074894494051159 ) ) ;
#23676=CARTESIAN_POINT ( 'NONE',  ( -0.1264236179284866091, -1.535925196796629866, 0.1264236179284866091 ) ) ;
#23679=CARTESIAN_POINT ( 'NONE',  ( 0.1270800023317771588, -0.6457131009216279249, -0.1270800023317771588 ) ) ;
#23683=CARTESIAN_POINT ( 'NONE',  ( 0.06523048226347956391, -0.3695866141732285781, 0.1574803149606297803 ) ) ;
#23685=DIRECTION ( 'NONE',  ( 0.000000000000000000, 0.000000000000000000, 1.000000000000000000 ) ) ;
#23696=CARTESIAN_POINT ( 'NONE',  ( -0.1605366408340857254, -0.08956085509329067551, -0.06625698018490121244 ) ) ;
#23697=CARTESIAN_POINT ( 'NONE',  ( 0.1787899950787401604, -0.5738188975840317063, 0.07405724077823318263 ) ) ;
#23705=CARTESIAN_POINT ( 'NONE',  ( -0.07405724077823318263, -1.725393700733637958, 0.1787899950787401604 ) ) ;
#23706=CARTESIAN_POINT ( 'NONE',  ( -0.07405724077823318263, -0.9035433070328510174, 0.1787899950787401604 ) ) ;
#23707=CARTESIAN_POINT ( 'NONE',  ( 0.06523048226347956391, -1.353838582677164393, 0.1574803149606297803 ) ) ;
#23724=CARTESIAN_POINT ( 'NONE',  ( 0.2471922904502826812, -0.09842519685039370636, -0.1427165354330708902 ) ) ;
#23731=CARTESIAN_POINT ( 'NONE',  ( 0.02145185034013027958, -0.09842519685039370636, -0.1903359544148515714 ) ) ;
#23736=CARTESIAN_POINT ( 'NONE',  ( -0.07405724077823318263, -1.036417322780882833, -0.1787899950787401604 ) ) ;
#23737=CARTESIAN_POINT ( 'NONE',  ( -0.1787899950787401604, -1.179133858213953001, 0.07405724077823318263 ) ) ;
#23740=CARTESIAN_POINT ( 'NONE',  ( 0.07444174185955046430, -0.5251422347798958556, -0.1797182628040039087 ) ) ;
#23741=CARTESIAN_POINT ( 'NONE',  ( -0.06523048226347956391, 0.08316929133858275147, -0.1574803149606300301 ) ) ;
#23749=CARTESIAN_POINT ( 'NONE',  ( -0.1787899950787401882, -0.3597440944344256208, 0.000000000000000000 ) ) ;
#23751=CARTESIAN_POINT ( 'NONE',  ( -0.1787899950787401604, -1.380905511757260173, -0.07405724077823318263 ) ) ;
#23763=CARTESIAN_POINT ( 'NONE',  ( 0.1598064471924473817, -0.09842432027591681287, -0.08022707942853385399 ) ) ;
#23772=CARTESIAN_POINT ( 'NONE',  ( -0.06406129441507303623, -0.09851384877607578805, 0.2183140915305173402 ) ) ;
#23777=CARTESIAN_POINT ( 'NONE',  ( 0.1264236179284866091, -1.576403495788293530, 0.1264236179284866091 ) ) ;
#23780=CARTESIAN_POINT ( 'NONE',  ( 0.1787899950787401882, -0.5713582676627716461, -2.189545951927503898E-17 ) ) ;
#23781=CARTESIAN_POINT ( 'NONE',  ( 2.892866454678787531E-17, 0.07086614183981043702, 0.1574803149606299191 ) ) ;
#23788=CARTESIAN_POINT ( 'NONE',  ( 0.07405724077823318263, -0.8001968503399367050, -0.1787899950787401604 ) ) ;
#23792=CARTESIAN_POINT ( 'NONE',  ( 0.1787899950787401882, -0.03604916507963244754, -2.189545951927503898E-17 ) ) ;
#23793=CARTESIAN_POINT ( 'NONE',  ( -0.1787899950787401882, 0.1520669291876218521, 0.000000000000000000 ) ) ;
#23796=CARTESIAN_POINT ( 'NONE',  ( -0.1113553986120547346, -0.9281496062992126150, 0.1113553986120547346 ) ) ;
#23797=CARTESIAN_POINT ( 'NONE',  ( -1.100456976456230270E-17, -1.546303652102730242, -0.1797182628040039365 ) ) ;
#23799=CARTESIAN_POINT ( 'NONE',  ( -0.06523048226347956391, -0.4827755904436537571, 0.1574803149606297803 ) ) ;
#23800=CARTESIAN_POINT ( 'NONE',  ( 0.1787899950787401604, -0.4163385826234020093, 0.07405724077823318263 ) ) ;
#23808=CARTESIAN_POINT ( 'NONE',  ( 1.928577636452524610E-17, -0.09842519685039370636, -0.1574803149606299191 ) ) ;
#23809=CARTESIAN_POINT ( 'NONE',  ( -0.07405724077823318263, 0.02657480320336980464, -0.1787899950787401604 ) ) ;
#23820=CARTESIAN_POINT ( 'NONE',  ( 0.1113553986120547346, -1.105314960522393752, 0.1113553986120547346 ) ) ;
#23821=CARTESIAN_POINT ( 'NONE',  ( -0.07405724077823318263, -1.312007873961984705, -0.1787899950787401604 ) ) ;
#23836=CARTESIAN_POINT ( 'NONE',  ( -0.1787899950787401604, 0.07578740162856664742, 0.07405724077823318263 ) ) ;
#23837=DIRECTION ( 'NONE',  ( -1.000000000000000000, 0.000000000000000000, 2.392722035830075028E-16 ) ) ;
#23840=CARTESIAN_POINT ( 'NONE',  ( -0.06523048226347956391, -0.2071850392625517456, 0.1574803149606297803 ) ) ;
#23844=CARTESIAN_POINT ( 'NONE',  ( -0.1787899950787401604, -1.199927117835539292, -0.07405724077823318263 ) ) ;
#23846=CARTESIAN_POINT ( 'NONE',  ( 0.1787899950787401604, -0.1751968503399373434, -0.07405724077823318263 ) ) ;
#23856=CARTESIAN_POINT ( 'NONE',  ( -0.1264236179284866091, -0.6697834645131652831, 0.1264236179284866091 ) ) ;
#23860=CARTESIAN_POINT ( 'NONE',  ( 3.301370929368692659E-17, -1.172287904071234177, 0.1797182628040039365 ) ) ;
#23869=CARTESIAN_POINT ( 'NONE',  ( 0.1574803149606300301, -0.7485236219397169988, 0.06523048226347956391 ) ) ;
#23880=CARTESIAN_POINT ( 'NONE',  ( -0.1574803149606300301, -1.673720472333417808, -0.06523048226347956391 ) ) ;
#23886=CARTESIAN_POINT ( 'NONE',  ( 0.1264236179284866091, 0.09301181107738563936, 0.1264236179284866091 ) ) ;
#23895=CARTESIAN_POINT ( 'NONE',  ( -0.1787899950787401604, -1.740157480261197875, -0.07405724077823318263 ) ) ;
#23904=CARTESIAN_POINT ( 'NONE',  ( 0.1264236179284866091, -0.7496318422449862462, 0.1264236179284866091 ) ) ;
#23907=CARTESIAN_POINT ( 'NONE',  ( -0.1552293633745783497, -0.08956123932130295728, -0.08013377253620669605 ) ) ;
#23917=CARTESIAN_POINT ( 'NONE',  ( -0.07405724077823318263, -1.454724409395055096, 0.1787899950787401604 ) ) ;
#23921=CARTESIAN_POINT ( 'NONE',  ( -0.1797182628040039365, -0.7490595576145413492, 0.000000000000000000 ) ) ;
#23926=CARTESIAN_POINT ( 'NONE',  ( -0.1574803149606300301, -0.5024606299212598381, -0.06523048226347956391 ) ) ;
#23934=CARTESIAN_POINT ( 'NONE',  ( 0.1574803149606300301, 0.07824803160359000698, 0.06523048226347956391 ) ) ;
#23941=CARTESIAN_POINT ( 'NONE',  ( -0.1667349855531194136, -0.08956067304632099602, -0.04285543117372075245 ) ) ;
#23942=CARTESIAN_POINT ( 'NONE',  ( 0.07405724077823318263, -0.6033464566391496531, -0.1787899950787401604 ) ) ;
#23947=EDGE_LOOP ( 'NONE', ( #40757, #9341, #26605, #25361, #3422, #41546 ) ) ;
#23951=CARTESIAN_POINT ( 'NONE',  ( -0.1264236179284866091, -1.767224409395055318, 0.1264236179284866091 ) ) ;
#23952=CARTESIAN_POINT ( 'NONE',  ( 3.284318927891251994E-17, -1.097933070812378009, 0.1787899950787401882 ) ) ;
#23953=CARTESIAN_POINT ( 'NONE',  ( -0.1113553986120547346, -1.400590551181102539, 0.1113553986120547346 ) ) ;
#23972=CARTESIAN_POINT ( 'NONE',  ( -0.1787899950787401882, -0.2132145194103413355, 0.000000000000000000 ) ) ;
#23974=CARTESIAN_POINT ( 'NONE',  ( 0.1312289434299238056, -0.09842519685039231858, -0.1483208907156891854 ) ) ;
#23982=CARTESIAN_POINT ( 'NONE',  ( 0.1264236179284866091, -1.093011810969858333, 0.1264236179284866091 ) ) ;
#23983=CARTESIAN_POINT ( 'NONE',  ( 0.1264236179284866091, -1.245570866087968520, 0.1264236179284866091 ) ) ;
#23987=CARTESIAN_POINT ( 'NONE',  ( -0.07444174185955065859, -0.4267170379295021632, 0.1797182628040039087 ) ) ;
#23991=CARTESIAN_POINT ( 'NONE',  ( 0.1113553986120547346, 0.02657480314960630058, 0.1113553986120547346 ) ) ;
#23999=CARTESIAN_POINT ( 'NONE',  ( -0.1264236179284866091, -0.3548228345919058890, 0.1264236179284866091 ) ) ;
#24000=CARTESIAN_POINT ( 'NONE',  ( 2.892866454678787531E-17, 0.02165354330708661734, 0.1574803149606299191 ) ) ;
#24001=CARTESIAN_POINT ( 'NONE',  ( 0.07405724077823318263, -1.351377952702143004, -0.1787899950787401604 ) ) ;
#24004=VERTEX_POINT ( 'NONE', #24000 ) ;
#24013=CARTESIAN_POINT ( 'NONE',  ( 2.892866454678787531E-17, -0.09645669291338582196, 0.1574803149606299191 ) ) ;
#24018=CARTESIAN_POINT ( 'NONE',  ( -0.1749793193338634034, -0.09851385152415884083, 0.1545203862959413366 ) ) ;
#24024=CARTESIAN_POINT ( 'NONE',  ( 0.1787899950787401604, -1.613312944607189880, 0.07405724077823318263 ) ) ;
#24027=CARTESIAN_POINT ( 'NONE',  ( 0.1787899950787401882, -0.6500984251430865779, -2.189545951927503898E-17 ) ) ;
#24034=CARTESIAN_POINT ( 'NONE',  ( -0.07405724077823318263, -0.3671259841982050798, -0.1787899950787401604 ) ) ;
#24036=CARTESIAN_POINT ( 'NONE',  ( -0.1264236179284866091, -0.7436023621509606496, 0.1264236179284866091 ) ) ;
#24041=CARTESIAN_POINT ( 'NONE',  ( 0.07405724077823318263, 0.08944296090461954785, -0.1787899950787401604 ) ) ;
#24042=CARTESIAN_POINT ( 'NONE',  ( -0.1264236179284866091, 0.1176181102899840625, 0.1264236179284866091 ) ) ;
#24048=CARTESIAN_POINT ( 'NONE',  ( -0.06523048226347956391, -0.9010826771653551726, -0.1574803149606300301 ) ) ;
#24050=CARTESIAN_POINT ( 'NONE',  ( 0.07444174185955046430, -1.548764282023991301, -0.1797182628040039087 ) ) ;
#24051=CARTESIAN_POINT ( 'NONE',  ( 2.892866454678787531E-17, -0.4409448817822370081, 0.1574803149606299191 ) ) ;
#24060=CARTESIAN_POINT ( 'NONE',  ( 0.07405724077823318263, -0.01771653537930735489, -0.1787899950787401604 ) ) ;
#24062=CARTESIAN_POINT ( 'NONE',  ( -0.07405724077823318263, -0.8986220471903317852, 0.1787899950787401604 ) ) ;
#24070=CARTESIAN_POINT ( 'NONE',  ( -0.1574803149606299191, -1.080708661309795371, 0.000000000000000000 ) ) ;
#24071=CARTESIAN_POINT ( 'NONE',  ( 0.1264236179284866091, -1.319389763725763665, -0.1264236179284866091 ) ) ;
#24084=CARTESIAN_POINT ( 'NONE',  ( 0.1515708385138894443, 0.1286422661082891605, 0.1012763973430838016 ) ) ;
#24090=CARTESIAN_POINT ( 'NONE',  ( -0.1264236179284866091, -1.123647590276482200, -0.1264236179284866091 ) ) ;
#24092=CARTESIAN_POINT ( 'NONE',  ( -0.1787899950787401604, -0.08169291333206318839, -0.07405724077823318263 ) ) ;
#24101=AXIS2_PLACEMENT_3D ( 'NONE', #3586, #6459, #25412 ) ;
#24102=CARTESIAN_POINT ( 'NONE',  ( 3.284318927891251994E-17, -0.6254921259304881964, 0.1787899950787401882 ) ) ;
#24106=CARTESIAN_POINT ( 'NONE',  ( 0.1797182628040039087, -1.125535935567297807, 0.07444174185955046430 ) ) ;
#24115=CARTESIAN_POINT ( 'NONE',  ( -0.1026092249587055166, 0.1299212598425196763, 0.1321676130798911386 ) ) ;
#24117=CARTESIAN_POINT ( 'NONE',  ( -1.094772975963752103E-17, 0.1077755906049446960, -0.1787899950787401882 ) ) ;
#24124=CARTESIAN_POINT ( 'NONE',  ( 0.06523048226347956391, -1.722933070758614349, -0.1574803149606300301 ) ) ;
#24132=CARTESIAN_POINT ( 'NONE',  ( -0.1787899950787401882, 0.1569881890301415284, 0.000000000000000000 ) ) ;
#24138=CARTESIAN_POINT ( 'NONE',  ( -0.08837071341806060354, 0.09266989036297286486, 0.2344122156857451345 ) ) ;
#24141=CARTESIAN_POINT ( 'NONE',  ( -0.1787899950787401604, -1.695866141678520567, 0.07405724077823318263 ) ) ;
#24148=CARTESIAN_POINT ( 'NONE',  ( 0.1533123297493048931, 0.1250557930784849670, -0.05373872839130795082 ) ) ;
#24151=CARTESIAN_POINT ( 'NONE',  ( -0.06782836439666850570, -0.08956100471190649170, -0.1695658838066383955 ) ) ;
#24164=CARTESIAN_POINT ( 'NONE',  ( 0.1797182628040039087, -0.7662839670633605493, -0.07444174185955065859 ) ) ;
#24167=CARTESIAN_POINT ( 'NONE',  ( 0.1574803149606300301, -0.4040354330708660902, 0.06523048226347956391 ) ) ;
#24179=CARTESIAN_POINT ( 'NONE',  ( 0.000000000000000000, -0.09842519685039370636, 0.000000000000000000 ) ) ;
#24181=CARTESIAN_POINT ( 'NONE',  ( 0.1787899950787401882, -0.4926181101824567143, -2.189545951927503898E-17 ) ) ;
#24188=CARTESIAN_POINT ( 'NONE',  ( 0.1797182628040039087, 0.1343065841177418784, 0.07444174185955046430 ) ) ;
#24189=CARTESIAN_POINT ( 'NONE',  ( 0.1787899950787401604, -1.129921259788756682, 0.07405724077823318263 ) ) ;
#24190=CARTESIAN_POINT ( 'NONE',  ( 0.1574803149606299191, -1.346456692913385877, -1.928577636452523993E-17 ) ) ;
#24204=CARTESIAN_POINT ( 'NONE',  ( 0.05554372828378647403, -0.07731288306167657942, -0.2533648624690311157 ) ) ;
#24207=CARTESIAN_POINT ( 'NONE',  ( 0.1787899950787401604, -0.2353601887016795458, 0.07405724077823318263 ) ) ;
#24210=CARTESIAN_POINT ( 'NONE',  ( 0.06844676939238621138, -0.09842519685039370636, 0.2099670925079330785 ) ) ;
#24211=CARTESIAN_POINT ( 'NONE',  ( -0.1113553986120547346, 0.006889763779527558960, -0.1113553986120547346 ) ) ;
#24218=CARTESIAN_POINT ( 'NONE',  ( -0.1264236179284866091, -0.9945866141194644738, -0.1264236179284866091 ) ) ;
#24219=CARTESIAN_POINT ( 'NONE',  ( 0.1787899950787401882, -1.280019684985606254, -2.189545951927503898E-17 ) ) ;
#24223=CARTESIAN_POINT ( 'NONE',  ( -1.100456976456230270E-17, -0.4833115261184787181, -0.1797182628040039365 ) ) ;
#24227=CARTESIAN_POINT ( 'NONE',  ( -0.06523048226347956391, -0.05954724409448820810, 0.1574803149606297803 ) ) ;
#24235=CARTESIAN_POINT ( 'NONE',  ( 0.1787899950787401882, -0.5762795275052914334, -2.189545951927503898E-17 ) ) ;
#24236=CARTESIAN_POINT ( 'NONE',  ( -1.094772975963752103E-17, -1.348917322780881944, -0.1787899950787401882 ) ) ;
#24255=CARTESIAN_POINT ( 'NONE',  ( 0.1778978046402051039, -0.09851384678937105677, 0.1186814646440462612 ) ) ;
#24257=B_SPLINE_CURVE_WITH_KNOTS ( 'NONE', 3,
 ( #43202, #9935, #21409, #25016, #20702, #38697, #28395, #2488, #46337, #35343, #35576, #17826, #5869, #17114, #16878, #24778, #17584, #44106, #24542 ),
 .UNSPECIFIED., .F., .F.,
 ( 4, 1, 1, 1, 2, 2, 1, 1, 1, 1, 2, 2, 4 ),
 ( 0.000000000000000000, 0.1250000000000016376, 0.1875000000000024425, 0.2187500000000027756, 0.2343750000000029976, 0.2500000000000031641, 0.3750000000000044409, 0.4375000000000049960, 0.4687500000000053846, 0.4843750000000054956, 0.4921875000000056066, 0.5000000000000056621, 1.000000000000000000 ),
 .UNSPECIFIED. ) ;
#24260=CARTESIAN_POINT ( 'NONE',  ( -0.1787899950787401882, -1.551797196575694926, 0.000000000000000000 ) ) ;
#24263=CARTESIAN_POINT ( 'NONE',  ( 0.1264236179284866091, -0.6058070865604094912, -0.1264236179284866091 ) ) ;
#24267=CARTESIAN_POINT ( 'NONE',  ( 0.1787899950787401882, -0.3400590550643468601, -2.189545951927503898E-17 ) ) ;
#24268=CARTESIAN_POINT ( 'NONE',  ( -0.07405724077823318263, -0.7017716534895438452, 0.1787899950787401604 ) ) ;
#24272=CARTESIAN_POINT ( 'NONE',  ( 3.284318927891251994E-17, 0.03284847271564315246, 0.1787899950787401882 ) ) ;
#24273=CARTESIAN_POINT ( 'NONE',  ( -0.1787899950787401604, 0.03641732288840918152, 0.07405724077823318263 ) ) ;
#24279=CARTESIAN_POINT ( 'NONE',  ( 0.1574803149606300301, -0.8715551181102356715, -0.06523048226347956391 ) ) ;
#24281=CARTESIAN_POINT ( 'NONE',  ( -0.1797182628040039087, -1.499551683598794982, -0.07444174185955065859 ) ) ;
#24283=CARTESIAN_POINT ( 'NONE',  ( -1.094772975963752103E-17, -0.4040354330171023745, -0.1787899950787401882 ) ) ;
#24289=CARTESIAN_POINT ( 'NONE',  ( -0.2137641352136847028, -0.06208088008912424766, -0.1620118252825171745 ) ) ;
#24292=CARTESIAN_POINT ( 'NONE',  ( 0.1264236179284866091, -0.1087598424659214497, 0.1264236179284866091 ) ) ;
#24294=CARTESIAN_POINT ( 'NONE',  ( -0.1787899950787401604, -0.9429133857730090940, 0.07405724077823318263 ) ) ;
#24306=DIRECTION ( 'NONE',  ( 0.000000000000000000, 1.000000000000000000, 0.000000000000000000 ) ) ;
#24319=CARTESIAN_POINT ( 'NONE',  ( -0.1787899950787401882, -1.079356251693805113, 0.000000000000000000 ) ) ;
#24321=CARTESIAN_POINT ( 'NONE',  ( 0.1264236179284866091, -0.1432086613635592531, 0.1264236179284866091 ) ) ;
#24328=CARTESIAN_POINT ( 'NONE',  ( -0.07444174185955065859, -0.1265201875358013817, -0.1797182628040039087 ) ) ;
#24329=CARTESIAN_POINT ( 'NONE',  ( 0.1787899950787401604, -0.7706692912848194243, -0.07405724077823318263 ) ) ;
#24333=CARTESIAN_POINT ( 'NONE',  ( -0.1270800023317771588, -1.187051683598793428, -0.1270800023317771588 ) ) ;
#24344=CARTESIAN_POINT ( 'NONE',  ( -0.07405724077823318263, 0.006889763833291078637, 0.1787899950787401604 ) ) ;
#24354=CARTESIAN_POINT ( 'NONE',  ( 0.05836929678887253087, -0.07899262986804667097, 0.2517335218907257310 ) ) ;
#24357=CARTESIAN_POINT ( 'NONE',  ( -0.06523048226347956391, -1.767224409448819866, -0.1574803149606300301 ) ) ;
#24359=ADVANCED_FACE ( 'NONE', ( #37313 ), #34713, .T. ) ;
#24364=CARTESIAN_POINT ( 'NONE',  ( 0.1787899950787401604, -1.636811023568283341, -0.07405724077823318263 ) ) ;
#24370=CARTESIAN_POINT ( 'NONE',  ( 0.1574028386749138364, 0.1230214933236144365, -0.03225005981621940909 ) ) ;
#24373=CARTESIAN_POINT ( 'NONE',  ( -0.1104063604032177182, -0.08956089369968209257, -0.1415710564723076936 ) ) ;
#24374=CARTESIAN_POINT ( 'NONE',  ( 0.2471922904502826812, -0.09842519685039370636, 0.1427165354330708902 ) ) ;
#24384=ADVANCED_BREP_SHAPE_REPRESENTATION ( 'Threaded Bushing', ( #36588, #20860 ), #22411 ) ;
#24387=CARTESIAN_POINT ( 'NONE',  ( -0.1270800023317771588, -0.6752406599767460937, -0.1270800023317771588 ) ) ;
#24388=CARTESIAN_POINT ( 'NONE',  ( 0.2471922904502827090, 0.07885719401822738339, 0.07558487950069545103 ) ) ;
#24390=CARTESIAN_POINT ( 'NONE',  ( -9.642888182262618425E-18, -0.3917322834645669549, -0.1574803149606299191 ) ) ;
#24391=DIRECTION ( 'NONE',  ( 0.000000000000000000, 0.000000000000000000, 1.000000000000000000 ) ) ;
#24401=AXIS2_PLACEMENT_3D ( 'NONE', #14496, #26240, #40338 ) ;
#24403=CARTESIAN_POINT ( 'NONE',  ( -0.1235961452251413406, 0.09842519685039370636, 0.2140748031496062798 ) ) ;
#24409=DIRECTION ( 'NONE',  ( 0.000000000000000000, 1.000000000000000000, 0.000000000000000000 ) ) ;
#24410=CARTESIAN_POINT ( 'NONE',  ( 0.1797182628040039087, 0.02111760773978908073, -0.07444174185955065859 ) ) ;
#24411=CARTESIAN_POINT ( 'NONE',  ( 0.07405724077823318263, -1.041338582623402287, -0.1787899950787401604 ) ) ;
#24412=CARTESIAN_POINT ( 'NONE',  ( 0.1113553986120547346, -1.341535433070866201, -0.1113553986120547346 ) ) ;
#24419=ORIENTED_EDGE ( 'NONE', *, *, #17008, .T. ) ;
#24425=CARTESIAN_POINT ( 'NONE',  ( -0.2471922904502826535, 0.08140987345728177560, 0.07064030526712006264 ) ) ;
#24427=CARTESIAN_POINT ( 'NONE',  ( -0.1528720448724869563, 0.09445537554013619386, 0.1971723546074427569 ) ) ;
#24430=CARTESIAN_POINT ( 'NONE',  ( 0.07405724077823318263, -0.2402814485441996661, 0.1787899950787401604 ) ) ;
#24431=CARTESIAN_POINT ( 'NONE',  ( 0.1605230700181201065, -0.09842519685039370636, 0.1447514863646086891 ) ) ;
#24437=CARTESIAN_POINT ( 'NONE',  ( 3.284318927891251994E-17, -1.097933070812378009, 0.1787899950787401882 ) ) ;
#24438=CARTESIAN_POINT ( 'NONE',  ( 0.07405724077823318263, -1.287401574749386768, 0.1787899950787401604 ) ) ;
#24440=DIRECTION ( 'NONE',  ( -1.000000000000000000, 0.000000000000000000, 0.000000000000000000 ) ) ;
#24442=CARTESIAN_POINT ( 'NONE',  ( 0.07444174185955046430, -0.4857721560397386673, -0.1797182628040039087 ) ) ;
#24447=CARTESIAN_POINT ( 'NONE',  ( -0.06523048226347956391, -0.02017716535433068670, 0.1574803149606297803 ) ) ;
#24455=CARTESIAN_POINT ( 'NONE',  ( 0.000000000000000000, 0.09842519685039370636, 0.000000000000000000 ) ) ;
#24457=CARTESIAN_POINT ( 'NONE',  ( -1.094772975963752103E-17, -0.6058070865604094912, -0.1787899950787401882 ) ) ;
#24458=CARTESIAN_POINT ( 'NONE',  ( -0.1264236179284866091, -1.383366141678519678, -0.1264236179284866091 ) ) ;
#24468=CARTESIAN_POINT ( 'NONE',  ( 0.1113553986120547346, -1.262795275483023394, 0.1113553986120547346 ) ) ;
#24471=CARTESIAN_POINT ( 'NONE',  ( 0.1346784485371297357, -0.09842520765884796297, -0.1175907832281543053 ) ) ;
#24478=B_SPLINE_CURVE_WITH_KNOTS ( 'NONE', 3,
 ( #3685, #14717, #39855, #29390, #14482, #11133, #22362, #17595, #25755, #47059, #36303, #28654, #43214, #25024, #6800, #3206, #17836, #29141, #32479, #14253, #3454, #10902, #1254 ),
 .UNSPECIFIED., .F., .F.,
 ( 4, 2, 2, 1, 1, 1, 2, 2, 2, 1, 1, 2, 2, 4 ),
 ( 0.000000000000000000, 0.2499999999999978906, 0.3749999999999967248, 0.4374999999999960032, 0.4687499999999957812, 0.4843749999999957812, 0.4921874999999958367, 0.4999999999999958922, 0.6249999999999973355, 0.6874999999999981126, 0.7187499999999983347, 0.7343749999999984457, 0.7499999999999985567, 1.000000000000000000 ),
 .UNSPECIFIED. ) ;
#24484=CARTESIAN_POINT ( 'NONE',  ( -0.2364785587839823289, -0.09851385148207500442, -0.06085331962129881395 ) ) ;
#24487=CARTESIAN_POINT ( 'NONE',  ( 0.07405724077823318263, -1.618234204449711111, 0.1787899950787401604 ) ) ;
#24489=CARTESIAN_POINT ( 'NONE',  ( 0.1787899950787401604, -0.6082677164816695514, -0.07405724077823318263 ) ) ;
#24492=EDGE_LOOP ( 'NONE', ( #38690, #19282, #6689, #4242, #15007, #29558 ) ) ;
#24495=CARTESIAN_POINT ( 'NONE',  ( 0.07405724077823318263, -0.2933070865604095467, -0.1787899950787401604 ) ) ;
#24496=CARTESIAN_POINT ( 'NONE',  ( -0.1787899950787401604, -0.7854330708123791194, 0.07405724077823318263 ) ) ;
#24498=DIRECTION ( 'NONE',  ( 0.000000000000000000, 0.000000000000000000, 1.000000000000000000 ) ) ;
#24501=CARTESIAN_POINT ( 'NONE',  ( 0.07405724077823318263, -0.02866727531585293309, -0.1787899950787401604 ) ) ;
#24506=CARTESIAN_POINT ( 'NONE',  ( -9.642888182262618425E-18, -0.8248031496062991907, -0.1574803149606299191 ) ) ;
#24508=CARTESIAN_POINT ( 'NONE',  ( -0.1797182628040039365, -1.693941447378320753, 0.000000000000000000 ) ) ;
#24511=CARTESIAN_POINT ( 'NONE',  ( 0.2471922904502826812, 0.03219022224904102836, -0.1427165354330708902 ) ) ;
#24517=CARTESIAN_POINT ( 'NONE',  ( 0.1787899950787401882, -0.1825787401037169411, -2.189545951927503898E-17 ) ) ;
#24519=CARTESIAN_POINT ( 'NONE',  ( -0.1787899950787401604, -0.9822834645131651721, 0.07405724077823318263 ) ) ;
#24542=CARTESIAN_POINT ( 'NONE',  ( -0.2471922904502826812, 0.03219022224904098672, -0.1427165354330708902 ) ) ;
#24544=CARTESIAN_POINT ( 'NONE',  ( 0.07405724077823318263, -1.145793259567821520, 0.1787899950787401604 ) ) ;
#24546=CARTESIAN_POINT ( 'NONE',  ( -0.1787899950787401604, -0.04232283459190578495, -0.07405724077823318263 ) ) ;
#24547=EDGE_LOOP ( 'NONE', ( #22182, #7000, #42084, #1517 ) ) ;
#24550=CARTESIAN_POINT ( 'NONE',  ( 0.07444174185955046430, -0.2495516835987934279, -0.1797182628040039087 ) ) ;
#24551=CARTESIAN_POINT ( 'NONE',  ( 0.1787899950787401604, -0.8100393700249772788, -0.07405724077823318263 ) ) ;
#24557=CARTESIAN_POINT ( 'NONE',  ( -0.1797182628040039087, -1.337150108795643888, 0.07444174185955065859 ) ) ;
#24587=CARTESIAN_POINT ( 'NONE',  ( 0.1787899950787401882, 0.01919291343959027632, -2.189545951927503898E-17 ) ) ;
#24589=ORIENTED_EDGE ( 'NONE', *, *, #18454, .F. ) ;
#24593=CARTESIAN_POINT ( 'NONE',  ( 0.1264236179284866091, -1.644192913332062966, 0.1264236179284866091 ) ) ;
#24601=CARTESIAN_POINT ( 'NONE',  ( -0.07405724077823318263, -0.6930373540560104129, -0.1787899950787401604 ) ) ;
#24603=CARTESIAN_POINT ( 'NONE',  ( 0.1081428761283521750, -0.08956233663024114333, 0.09372579465688228584 ) ) ;
#24620=CARTESIAN_POINT ( 'NONE',  ( 0.2471922904502826812, 0.09336655125506181097, 0.03811874944176495139 ) ) ;
#24622=ADVANCED_FACE ( 'NONE', ( #37238 ), #34254, .T. ) ;
#24623=CARTESIAN_POINT ( 'NONE',  ( 0.1113553986120547346, -0.5935039370078740717, -0.1113553986120547346 ) ) ;
#24647=CARTESIAN_POINT ( 'NONE',  ( -1.100456976456230270E-17, 0.1072396549838836588, -0.1797182628040039365 ) ) ;
#24648=CARTESIAN_POINT ( 'NONE',  ( -0.1264236179284866091, -0.9945866141194644738, -0.1264236179284866091 ) ) ;
#24649=CARTESIAN_POINT ( 'NONE',  ( -9.642888182262618425E-18, -1.494094488188976388, -0.1574803149606299191 ) ) ;
#24650=B_SPLINE_CURVE_WITH_KNOTS ( 'NONE', 3,
 ( #9563, #28024, #46428, #20795, #39237, #31385 ),
 .UNSPECIFIED., .F., .F.,
 ( 4, 2, 4 ),
 ( 0.000000000000000000, 0.5000000000000000000, 1.000000000000000000 ),
 .UNSPECIFIED. ) ;
#24672=ORIENTED_EDGE ( 'NONE', *, *, #40190, .T. ) ;
#24675=CARTESIAN_POINT ( 'NONE',  ( -0.1264236179284866091, -1.112696850339937038, -0.1264236179284866091 ) ) ;
#24676=CARTESIAN_POINT ( 'NONE',  ( -0.07405724077823318263, -1.174212598371433769, 0.1787899950787401604 ) ) ;
#24679=CARTESIAN_POINT ( 'NONE',  ( 0.1797182628040039087, -0.5694335733625731644, -0.07444174185955065859 ) ) ;
#24682=CARTESIAN_POINT ( 'NONE',  ( 0.1574803149606300301, -0.2071850393700788440, 0.06523048226347956391 ) ) ;
#24686=CARTESIAN_POINT ( 'NONE',  ( -0.1113553986120547346, -0.07185039370078739884, -0.1113553986120547346 ) ) ;
#24692=CARTESIAN_POINT ( 'NONE',  ( 0.1787899950787401604, -0.5787401574265509385, 0.07405724077823318263 ) ) ;
#24693=CARTESIAN_POINT ( 'NONE',  ( 0.06523048226347956391, -1.024114173228346525, -0.1574803149606300301 ) ) ;
#24701=CARTESIAN_POINT ( 'NONE',  ( 0.1519290731529907845, -0.09842257466124233745, -0.09437017930498711737 ) ) ;
#24708=CARTESIAN_POINT ( 'NONE',  ( 0.1574803149606300301, -0.1924212597349927445, -0.06523048226347956391 ) ) ;
#24715=CARTESIAN_POINT ( 'NONE',  ( -0.1598647906827895537, -0.09851385182058956802, 0.1688384727535816865 ) ) ;
#24718=CARTESIAN_POINT ( 'NONE',  ( -0.1787899950787401882, -1.669907432796167601, 0.000000000000000000 ) ) ;
#24720=CARTESIAN_POINT ( 'NONE',  ( -0.07405724077823318263, -0.5590551180564723444, -0.1787899950787401604 ) ) ;
#24722=ORIENTED_EDGE ( 'NONE', *, *, #16679, .F. ) ;
#24726=CARTESIAN_POINT ( 'NONE',  ( -0.1264236179284866091, -0.7534448818360000022, -0.1264236179284866091 ) ) ;
#24732=CARTESIAN_POINT ( 'NONE',  ( 0.1787899950787401604, -0.03850979500089227181, 0.07405724077823318263 ) ) ;
#24733=CARTESIAN_POINT ( 'NONE',  ( 3.284318927891251994E-17, 0.004429133912031243958, 0.1787899950787401882 ) ) ;
#24739=CARTESIAN_POINT ( 'NONE',  ( -0.06523048226347956391, -0.8863188976377954775, 0.1574803149606297803 ) ) ;
#24741=CARTESIAN_POINT ( 'NONE',  ( 0.1797182628040039365, -1.752996565488557090, -2.200913952912460540E-17 ) ) ;
#24742=CARTESIAN_POINT ( 'NONE',  ( 0.06523048226347956391, -0.5024606298137324067, -0.1574803149606300301 ) ) ;
#24749=CARTESIAN_POINT ( 'NONE',  ( -0.2020936974011077469, -0.07057211410350064384, -0.1687521643629676660 ) ) ;
#24752=CARTESIAN_POINT ( 'NONE',  ( -0.1787899950787401882, -0.08415354325332302654, 0.000000000000000000 ) ) ;
#24754=CARTESIAN_POINT ( 'NONE',  ( 0.1264236179284866091, -0.9601377952218268508, -0.1264236179284866091 ) ) ;
#24762=CARTESIAN_POINT ( 'NONE',  ( 0.1113553986120547346, -1.134842519577511810, -0.1113553986120547346 ) ) ;
#24773=CARTESIAN_POINT ( 'NONE',  ( -0.07405724077823318263, 0.02657480320336980464, -0.1787899950787401604 ) ) ;
#24778=CARTESIAN_POINT ( 'NONE',  ( -0.2471922904502826812, 0.07821434602335945729, -0.07684457919973873563 ) ) ;
#24780=CARTESIAN_POINT ( 'NONE',  ( -0.1787899950787401882, -1.276206645394592609, 0.000000000000000000 ) ) ;
#24782=CARTESIAN_POINT ( 'NONE',  ( 0.1787899950787401604, -0.06200787396198446239, 0.07405724077823318263 ) ) ;
#24789=B_SPLINE_CURVE_WITH_KNOTS ( 'NONE', 3,
 ( #8842, #22746, #37352, #23238, #23479, #4505, #38080, #37599, #19141, #35209, #34974, #46199, #5483, #31619, #13398, #45718, #28028, #38788, #42587 ),
 .UNSPECIFIED., .F., .F.,
 ( 4, 1, 1, 1, 2, 2, 1, 1, 1, 1, 2, 2, 4 ),
 ( 0.000000000000000000, 0.1250000000000026645, 0.1875000000000038858, 0.2187500000000046074, 0.2343750000000049682, 0.2500000000000053291, 0.3750000000000067168, 0.4375000000000074385, 0.4687500000000076605, 0.4843750000000076605, 0.4921875000000074940, 0.5000000000000073275, 1.000000000000000000 ),
 .UNSPECIFIED. ) ;
#24790=CARTESIAN_POINT ( 'NONE',  ( -0.1787899950787401604, -1.459645669237573884, 0.07405724077823318263 ) ) ;
#24791=CARTESIAN_POINT ( 'NONE',  ( 0.07405724077823318263, -0.7657480314423001921, -0.1787899950787401604 ) ) ;
#24795=CARTESIAN_POINT ( 'NONE',  ( -0.07444174185955065859, -1.253488691472810279, 0.1797182628040039087 ) ) ;
#24818=CARTESIAN_POINT ( 'NONE',  ( -0.1264236179284866091, 0.04379921265218866822, 0.1264236179284866091 ) ) ;
#24821=ORIENTED_EDGE ( 'NONE', *, *, #47127, .T. ) ;
#24828=CARTESIAN_POINT ( 'NONE',  ( -0.1574803149606299191, -0.4114173227271181177, 0.000000000000000000 ) ) ;
#24829=CARTESIAN_POINT ( 'NONE',  ( -1.094772975963752103E-17, -1.629429133804503937, -0.1787899950787401882 ) ) ;
#24839=CARTESIAN_POINT ( 'NONE',  ( 0.07405724077823318263, -0.7373286926386874995, -0.1787899950787401604 ) ) ;
#24841=CARTESIAN_POINT ( 'NONE',  ( -0.1574803149606297803, -0.01525590540428398145, 0.06523048226347956391 ) ) ;
#24856=CARTESIAN_POINT ( 'NONE',  ( -1.100456976456230270E-17, -0.8376422347798956336, -0.1797182628040039365 ) ) ;
#24859=CARTESIAN_POINT ( 'NONE',  ( 0.1574803149606300301, -0.5615157480314956207, 0.06523048226347956391 ) ) ;
#24860=CARTESIAN_POINT ( 'NONE',  ( -0.1406027654606837041, 0.1242474013968406649, -0.08019598169044524216 ) ) ;
#24866=CARTESIAN_POINT ( 'NONE',  ( -9.642888182262618425E-18, -0.6181102361129449108, -0.1574803149606299191 ) ) ;
#24869=CARTESIAN_POINT ( 'NONE',  ( 0.1787899950787401604, -0.6476377952218281830, -0.07405724077823318263 ) ) ;
#24881=CARTESIAN_POINT ( 'NONE',  ( -0.1797182628040039087, 0.1146215447476630483, -0.07444174185955065859 ) ) ;
#24882=CARTESIAN_POINT ( 'NONE',  ( 0.1787899950787401604, -1.046259842465921297, -0.07405724077823318263 ) ) ;
#24883=CARTESIAN_POINT ( 'NONE',  ( -9.642888182262618425E-18, -1.533464566929133799, -0.1574803149606299191 ) ) ;
#24897=CARTESIAN_POINT ( 'NONE',  ( -0.2471922904502826535, 0.07794254751779101931, 0.07737183577689189795 ) ) ;
#24903=CARTESIAN_POINT ( 'NONE',  ( -0.1561257034333340399, -0.09842519685039370636, 0.06437166193198956554 ) ) ;
#24916=CARTESIAN_POINT ( 'NONE',  ( -0.1787899950787401604, -1.184055118056472455, 0.07405724077823318263 ) ) ;
#24917=CARTESIAN_POINT ( 'NONE',  ( -0.1787899950787401604, -1.459645669237573884, -0.07405724077823318263 ) ) ;
#24922=CARTESIAN_POINT ( 'NONE',  ( 0.1574803149606300301, -0.1235236220472441943, -0.06523048226347956391 ) ) ;
#24933=CARTESIAN_POINT ( 'NONE',  ( -0.1264236179284866091, -0.04478346451316559534, -0.1264236179284866091 ) ) ;
#24935=CARTESIAN_POINT ( 'NONE',  ( 0.06523048226347956391, -1.462106299105069951, 0.1574803149606297803 ) ) ;
#24936=CARTESIAN_POINT ( 'NONE',  ( 0.1787899950787401604, -0.5344488188438744070, -0.07405724077823318263 ) ) ;
#24937=CARTESIAN_POINT ( 'NONE',  ( -0.1574803149606300301, -1.093011811023621993, -0.06523048226347956391 ) ) ;
#24952=CARTESIAN_POINT ( 'NONE',  ( 0.1574803149606299191, -0.2342519683964098265, -1.928577636452523993E-17 ) ) ;
#24957=CARTESIAN_POINT ( 'NONE',  ( -0.1699452736636291317, -0.09851383556842245592, 0.02540171885215976658 ) ) ;
#24961=CARTESIAN_POINT ( 'NONE',  ( -0.07405724077823318263, -1.756029480040262269, -0.1787899950787401604 ) ) ;
#24967=CARTESIAN_POINT ( 'NONE',  ( -0.1787899950787401882, -0.3203740156942680994, 0.000000000000000000 ) ) ;
#24968=CARTESIAN_POINT ( 'NONE',  ( -0.1264236179284866091, -0.8617125983714329918, 0.1264236179284866091 ) ) ;
#24972=CARTESIAN_POINT ( 'NONE',  ( 0.07405724077823318263, -0.1074074327961678510, -0.1787899950787401604 ) ) ;
#24973=CARTESIAN_POINT ( 'NONE',  ( -1.094772975963752103E-17, -0.2859251967966303098, -0.1787899950787401882 ) ) ;
#24974=CARTESIAN_POINT ( 'NONE',  ( 0.1264236179284866091, 0.04872047249470835839, 0.1264236179284866091 ) ) ;
#24981=CARTESIAN_POINT ( 'NONE',  ( -0.1270800023317771588, -1.807130423756275972, 0.1270800023317771588 ) ) ;
#24987=CARTESIAN_POINT ( 'NONE',  ( -0.2278981769381095701, -0.05062618494087340465, -0.1538518510337364420 ) ) ;
#24990=CARTESIAN_POINT ( 'NONE',  ( 0.06523048226347956391, -0.9109251967428659835, 0.1574803149606297803 ) ) ;
#24991=CARTESIAN_POINT ( 'NONE',  ( -0.07405724077823318263, -0.1948818897100161873, 0.1787899950787401604 ) ) ;
#24993=CARTESIAN_POINT ( 'NONE',  ( 0.1787899950787401604, -1.124999999946237228, 0.07405724077823318263 ) ) ;
#25000=CARTESIAN_POINT ( 'NONE',  ( -0.1113553986120547346, -1.124999999892472458, -0.1113553986120547346 ) ) ;
#25012=CARTESIAN_POINT ( 'NONE',  ( -0.1787899950787401604, -0.002952755851748290004, 0.07405724077823318263 ) ) ;
#25016=CARTESIAN_POINT ( 'NONE',  ( -0.2471922904502826257, 0.09572725253288318081, -0.02812286105090850558 ) ) ;
#25018=CARTESIAN_POINT ( 'NONE',  ( 0.07405724077823318263, -1.288509795000891689, -0.1787899950787401604 ) ) ;
#25020=CARTESIAN_POINT ( 'NONE',  ( -0.1787899950787401604, -0.2785433070328505734, -0.07405724077823318263 ) ) ;
#25021=ORIENTED_EDGE ( 'NONE', *, *, #2007, .T. ) ;
#25024=CARTESIAN_POINT ( 'NONE',  ( -0.2471911249971451008, -0.08424752482805999976, 0.06442904123723289245 ) ) ;
#25028=CARTESIAN_POINT ( 'NONE',  ( -0.1264236179284866091, -1.654035433017102319, 0.1264236179284866091 ) ) ;
#25055=CARTESIAN_POINT ( 'NONE',  ( 0.1264236179284866091, 0.02411417328210995956, -0.1264236179284866091 ) ) ;
#25064=CARTESIAN_POINT ( 'NONE',  ( -0.1113553986120547346, 0.09547244105240886014, -0.1113553986120547346 ) ) ;
#25073=DIRECTION ( 'NONE',  ( 0.000000000000000000, 1.000000000000000000, 0.000000000000000000 ) ) ;
#25074=CARTESIAN_POINT ( 'NONE',  ( -0.1787899950787401604, -0.8013050705914438465, 0.07405724077823318263 ) ) ;
#25076=CARTESIAN_POINT ( 'NONE',  ( -0.1589669047091706866, -0.08956155894763247194, 0.04881376169791724201 ) ) ;
#25089=CARTESIAN_POINT ( 'NONE',  ( 0.1270800023317771588, -0.8130359355672972521, 0.1270800023317771588 ) ) ;
#25093=CARTESIAN_POINT ( 'NONE',  ( -0.1574803149606297803, -0.5762795275590550936, 0.06523048226347956391 ) ) ;
#25094=CARTESIAN_POINT ( 'NONE',  ( -0.1456127326761254559, 0.1283478695987083085, 0.08092402698540318573 ) ) ;
#25101=CARTESIAN_POINT ( 'NONE',  ( -0.1574803149606300301, -0.6107283463491653963, -0.06523048226347956391 ) ) ;
#25104=CARTESIAN_POINT ( 'NONE',  ( -0.1264236179284866091, -0.6747047243556849594, -0.1264236179284866091 ) ) ;
#25105=FACE_OUTER_BOUND ( 'NONE', #43929, .T. ) ;
#25112=CARTESIAN_POINT ( 'NONE',  ( -0.07444174185955065859, 0.04572390695238758712, 0.1797182628040039087 ) ) ;
#25113=CARTESIAN_POINT ( 'NONE',  ( -0.1787899950787401882, -1.186515747977732183, 0.000000000000000000 ) ) ;
#25114=CARTESIAN_POINT ( 'NONE',  ( -0.1574803149606300301, -1.565452755905512028, -0.06523048226347956391 ) ) ;
#25131=CARTESIAN_POINT ( 'NONE',  ( 3.284318927891251994E-17, -0.4002223934260890070, 0.1787899950787401882 ) ) ;
#25132=CARTESIAN_POINT ( 'NONE',  ( -0.1735869313432972239, -0.09842519685039370636, -0.005721762985481354535 ) ) ;
#25140=CARTESIAN_POINT ( 'NONE',  ( -0.07405724077823318263, -1.115157480261196987, -0.1787899950787401604 ) ) ;
#25141=CARTESIAN_POINT ( 'NONE',  ( -0.1787899950787401882, -1.339074803095842592, 0.000000000000000000 ) ) ;
#25146=CARTESIAN_POINT ( 'NONE',  ( -0.1270800023317771588, -0.5866579828113921424, 0.1270800023317771588 ) ) ;
#25151=CARTESIAN_POINT ( 'NONE',  ( -0.06523048226347956391, -0.1382874015748031260, 0.1574803149606297803 ) ) ;
#25164=ORIENTED_EDGE ( 'NONE', *, *, #5852, .T. ) ;
#25165=CARTESIAN_POINT ( 'NONE',  ( 0.1264236179284866091, -0.06446850388324429360, 0.1264236179284866091 ) ) ;
#25169=CARTESIAN_POINT ( 'NONE',  ( -0.06523048226347956391, -1.521161417215307177, -0.1574803149606300301 ) ) ;
#25170=CARTESIAN_POINT ( 'NONE',  ( -0.1264236179284866091, -0.6008858267178898149, -0.1264236179284866091 ) ) ;
#25171=CARTESIAN_POINT ( 'NONE',  ( -9.642888182262618425E-18, -1.061023622047244208, -0.1574803149606299191 ) ) ;
#25180=ORIENTED_EDGE ( 'NONE', *, *, #4876, .F. ) ;
#25187=CARTESIAN_POINT ( 'NONE',  ( -0.1113553986120547346, -0.2096456691838114172, 0.1113553986120547346 ) ) ;
#25189=ORIENTED_EDGE ( 'NONE', *, *, #32550, .T. ) ;
#25193=CARTESIAN_POINT ( 'NONE',  ( 0.1430555697033809026, -0.09851384659136652733, -0.1381766785746311177 ) ) ;
#25197=CARTESIAN_POINT ( 'NONE',  ( 3.284318927891251994E-17, -1.660064913111128249, 0.1787899950787401882 ) ) ;
#25202=CARTESIAN_POINT ( 'NONE',  ( -0.07405724077823318263, -0.4064960629383624346, -0.1787899950787401604 ) ) ;
#25203=CARTESIAN_POINT ( 'NONE',  ( -0.07405724077823318263, -0.8592519684501739308, 0.1787899950787401604 ) ) ;
#25207=CARTESIAN_POINT ( 'NONE',  ( 0.07405724077823318263, -0.1861475902764828938, -0.1787899950787401604 ) ) ;
#25208=CARTESIAN_POINT ( 'NONE',  ( 0.2471921892202938176, -0.09660984127287172707, -0.02628542481976669717 ) ) ;
#25212=CIRCLE ( 'NONE', #7619, 0.2204724409448818867 ) ;
#25215=CARTESIAN_POINT ( 'NONE',  ( 0.1797182628040039087, -1.750535935567296475, -0.07444174185955065859 ) ) ;
#25218=CARTESIAN_POINT ( 'NONE',  ( -0.1550311931537672050, -0.09383642490574117812, 0.1959255884475979703 ) ) ;
#25226=CARTESIAN_POINT ( 'NONE',  ( 0.07405724077823318263, -0.1505905511273389341, 0.1787899950787401604 ) ) ;
#25229=CARTESIAN_POINT ( 'NONE',  ( 0.1787899950787401604, -1.046259842465921297, 0.07405724077823318263 ) ) ;
#25236=AXIS2_PLACEMENT_3D ( 'NONE', #1586, #5905, #1830 ) ;
#25250=CARTESIAN_POINT ( 'NONE',  ( 0.1787899950787401604, 0.05118110241596821042, 0.07405724077823318263 ) ) ;
#25260=CARTESIAN_POINT ( 'NONE',  ( -0.1787899950787401882, -1.315576724134750242, 0.000000000000000000 ) ) ;
#25262=CARTESIAN_POINT ( 'NONE',  ( 0.1787899950787401882, -0.2957677164816697180, -2.189545951927503898E-17 ) ) ;
#25270=CARTESIAN_POINT ( 'NONE',  ( 3.284318927891251994E-17, -1.570374015694267600, 0.1787899950787401882 ) ) ;
#25271=CARTESIAN_POINT ( 'NONE',  ( 0.1264236179284866091, -0.7386811023084409733, 0.1264236179284866091 ) ) ;
#25274=CARTESIAN_POINT ( 'NONE',  ( 0.06841996760812382727, 0.1299212598425196763, 0.1651804176431311000 ) ) ;
#25275=CARTESIAN_POINT ( 'NONE',  ( -0.1797182628040039087, -1.263331211157848966, -0.07444174185955065859 ) ) ;
#25286=CARTESIAN_POINT ( 'NONE',  ( -0.1787899950787401882, 0.03887795280966901967, 0.000000000000000000 ) ) ;
#25298=AXIS2_PLACEMENT_3D ( 'NONE', #1993, #12570, #12807 ) ;
#25304=CARTESIAN_POINT ( 'NONE',  ( 0.1787899950787401604, 0.02165354336085011100, -0.07405724077823318263 ) ) ;
#25310=CARTESIAN_POINT ( 'NONE',  ( 0.1632645169460268941, -0.09126532511078781773, -0.1911722030488886837 ) ) ;
#25314=CARTESIAN_POINT ( 'NONE',  ( -0.1264236179284866091, -1.772145669237574994, 0.1264236179284866091 ) ) ;
#25323=CARTESIAN_POINT ( 'NONE',  ( -0.07405724077823318263, -0.8751239682292385469, 0.1787899950787401604 ) ) ;
#25325=CARTESIAN_POINT ( 'NONE',  ( -0.1574803149606300301, -0.02017716524680367163, -0.06523048226347956391 ) ) ;
#25343=CARTESIAN_POINT ( 'NONE',  ( -0.1270800023317771588, -0.8327209749373759573, -0.1270800023317771588 ) ) ;
#25348=CARTESIAN_POINT ( 'NONE',  ( -0.1574803149606299191, -0.5393700787401575214, 0.000000000000000000 ) ) ;
#25357=CARTESIAN_POINT ( 'NONE',  ( 0.1574803149606300301, -0.6254921258767247583, -0.06523048226347956391 ) ) ;
#25361=ORIENTED_EDGE ( 'NONE', *, *, #16679, .T. ) ;
#25366=CARTESIAN_POINT ( 'NONE',  ( -0.1787899950787401604, -1.184055118056472455, 0.07405724077823318263 ) ) ;
#25367=CARTESIAN_POINT ( 'NONE',  ( -0.1113553986120547346, -1.597440944881889813, 0.1113553986120547346 ) ) ;
#25374=CARTESIAN_POINT ( 'NONE',  ( 0.1574803149606300301, -0.3154527557979848185, 0.06523048226347956391 ) ) ;
#25386=CARTESIAN_POINT ( 'NONE',  ( -0.07405724077823318263, -0.3780767241347506857, -0.1787899950787401604 ) ) ;
#25387=CARTESIAN_POINT ( 'NONE',  ( 0.0003584782005013444962, -0.09842519685039370636, 0.1560556493606787276 ) ) ;
#25391=ORIENTED_EDGE ( 'NONE', *, *, #39318, .T. ) ;
#25395=CARTESIAN_POINT ( 'NONE',  ( 0.1787899950787401604, -1.243110236166709459, -0.07405724077823318263 ) ) ;
#25396=CARTESIAN_POINT ( 'NONE',  ( -0.1787899950787401882, -1.417814960576157635, 0.000000000000000000 ) ) ;
#25401=CARTESIAN_POINT ( 'NONE',  ( 3.301370929368692659E-17, -0.6211068017090294324, 0.1797182628040039365 ) ) ;
#25405=CARTESIAN_POINT ( 'NONE',  ( -0.06523048226347956391, -0.07431102362204727863, -0.1574803149606300301 ) ) ;
#25412=DIRECTION ( 'NONE',  ( 0.000000000000000000, 0.000000000000000000, 1.000000000000000000 ) ) ;
#25421=CARTESIAN_POINT ( 'NONE',  ( 0.1574803149606300301, -1.535925196742866650, 0.06523048226347956391 ) ) ;
#25422=CARTESIAN_POINT ( 'NONE',  ( -0.1264236179284866091, -0.6697834645131652831, 0.1264236179284866091 ) ) ;
#25424=CARTESIAN_POINT ( 'NONE',  ( -0.1574803149606299191, -1.129921259842519676, 0.000000000000000000 ) ) ;
#25441=CARTESIAN_POINT ( 'NONE',  ( 2.892866454678787531E-17, -0.2834645668216070891, 0.1574803149606299191 ) ) ;
#25446=CARTESIAN_POINT ( 'NONE',  ( -0.1736230502038370316, -0.09851383841496653970, -0.005720786448288354628 ) ) ;
#25451=CARTESIAN_POINT ( 'NONE',  ( -0.07405724077823318263, -1.701895621772544942, 0.1787899950787401604 ) ) ;
#25456=( BOUNDED_CURVE ( )  B_SPLINE_CURVE ( 2, ( #37487, #19744, #40583, #19270, #37018, #33926, #4171, #8723, #23358 ),
 .UNSPECIFIED., .F., .F. ) 
 B_SPLINE_CURVE_WITH_KNOTS ( ( 3, 2, 2, 2, 3 ),
 ( 0.1049999999999999961, 0.1074999999999999983, 0.1100000000000000006, 0.1125000000000000028, 0.1150000000000000050 ),
 .UNSPECIFIED. ) 
 CURVE ( )  GEOMETRIC_REPRESENTATION_ITEM ( )  RATIONAL_B_SPLINE_CURVE ( ( 1.000000000000000000, 0.9238795325112869605, 1.000000000000000000, 0.9238795325112869605, 1.000000000000000000, 0.9238795325112869605, 1.000000000000000000, 0.9238795325112869605, 1.000000000000000000 ) ) 
 REPRESENTATION_ITEM ( '' )  ) ;
#25457=CARTESIAN_POINT ( 'NONE',  ( 0.07405724077823318263, -0.3720472440407247561, -0.1787899950787401604 ) ) ;
#25458=CARTESIAN_POINT ( 'NONE',  ( -0.07405724077823318263, -0.8986220471903317852, 0.1787899950787401604 ) ) ;
#25462=CARTESIAN_POINT ( 'NONE',  ( 0.1797182628040039365, -0.2175634946224157540, -2.200913952912460540E-17 ) ) ;
#25463=CARTESIAN_POINT ( 'NONE',  ( -0.07405724077823318263, -0.08772239342608903478, 0.1787899950787401604 ) ) ;
#25464=CARTESIAN_POINT ( 'NONE',  ( 3.284318927891251994E-17, -0.2662401574265516047, 0.1787899950787401882 ) ) ;
#25465=CARTESIAN_POINT ( 'NONE',  ( 0.1264236179284866091, -0.05954724404072461036, -0.1264236179284866091 ) ) ;
#25471=CARTESIAN_POINT ( 'NONE',  ( 0.1797182628040039087, -1.671795778086982098, -0.07444174185955065859 ) ) ;
#25472=CARTESIAN_POINT ( 'NONE',  ( 3.284318927891251994E-17, -0.4237204723871811352, 0.1787899950787401882 ) ) ;
#25484=CARTESIAN_POINT ( 'NONE',  ( -0.1787899950787401604, -0.2047244093950554844, -0.07405724077823318263 ) ) ;
#25487=CARTESIAN_POINT ( 'NONE',  ( -0.1264236179284866091, -1.107775590497417362, -0.1264236179284866091 ) ) ;
#25496=B_SPLINE_CURVE_WITH_KNOTS ( 'NONE', 3,
 ( #9107, #41661, #9585, #34764, #16543, #31170, #31406, #13190, #35232, #24204, #27826, #5966, #20585, #21050, #14117, #42835, #33055, #35912, #10531, #7152, #29257, #32094, #21775 ),
 .UNSPECIFIED., .F., .F.,
 ( 4, 2, 2, 1, 1, 1, 2, 2, 2, 1, 1, 2, 2, 4 ),
 ( 0.000000000000000000, 0.2500000000000006106, 0.3750000000000008327, 0.4375000000000010547, 0.4687500000000012212, 0.4843750000000014433, 0.4921875000000014988, 0.5000000000000014433, 0.6250000000000012212, 0.6875000000000011102, 0.7187500000000009992, 0.7343750000000007772, 0.7500000000000005551, 1.000000000000000000 ),
 .UNSPECIFIED. ) ;
#25507=CARTESIAN_POINT ( 'NONE',  ( -0.1264236179284866091, -0.03986220467064590517, 0.1264236179284866091 ) ) ;
#25517=CARTESIAN_POINT ( 'NONE',  ( 0.07405724077823318263, -1.224533417048137451, 0.1787899950787401604 ) ) ;
#25519=CARTESIAN_POINT ( 'NONE',  ( -0.1787899950787401604, -0.3129921259304885850, 0.07405724077823318263 ) ) ;
#25531=CARTESIAN_POINT ( 'NONE',  ( 0.1787899950787401882, -1.678641732229700922, -2.189545951927503898E-17 ) ) ;
#25532=CARTESIAN_POINT ( 'NONE',  ( -0.1264236179284866091, -1.649114173174582643, 0.1264236179284866091 ) ) ;
#25534=CARTESIAN_POINT ( 'NONE',  ( -0.1545411696117860445, -0.09842519685039370636, -0.08990488994085453489 ) ) ;
#25539=CARTESIAN_POINT ( 'NONE',  ( 1.928577636452524610E-17, -0.09842519685039370636, -0.1574803149606299191 ) ) ;
#25555=CARTESIAN_POINT ( 'NONE',  ( 0.1787899950787401604, -0.1358267715997797664, -0.07405724077823318263 ) ) ;
#25564=CARTESIAN_POINT ( 'NONE',  ( -0.1574803149606299191, 0.1003937008949285503, 0.000000000000000000 ) ) ;
#25571=CARTESIAN_POINT ( 'NONE',  ( -0.07405724077823318263, -0.8357538894890804704, 0.1787899950787401604 ) ) ;
#25585=CARTESIAN_POINT ( 'NONE',  ( -0.07444174185955065859, -0.8351816048586360175, -0.1797182628040039087 ) ) ;
#25594=CARTESIAN_POINT ( 'NONE',  ( 0.1574803149606300301, 0.1176181103437476255, 0.06523048226347956391 ) ) ;
#25596=EDGE_CURVE ( 'NONE', #46651, #46167, #9703, .T. ) ;
#25600=CARTESIAN_POINT ( 'NONE',  ( -0.1264236179284866091, -0.7042322834108031282, 0.1264236179284866091 ) ) ;
#25603=CARTESIAN_POINT ( 'NONE',  ( -0.2471922904502826812, 0.03219022224904106305, 0.1427165354330708902 ) ) ;
#25606=CARTESIAN_POINT ( 'NONE',  ( 0.06523048226347956391, -1.535925196850394636, -0.1574803149606300301 ) ) ;
#25607=LINE ( 'NONE', #13857, #20651 ) ;
#25613=CONICAL_SURFACE ( 'NONE', #16439, 0.2471922904502826812, 0.5235987755982992597 ) ;
#25622=CARTESIAN_POINT ( 'NONE',  ( -0.1787899950787401604, -0.3682342044497113887, 0.07405724077823318263 ) ) ;
#25623=CARTESIAN_POINT ( 'NONE',  ( -0.1604209458837513869, -0.09842519685039370636, 0.05490810003033267522 ) ) ;
#25629=CARTESIAN_POINT ( 'NONE',  ( 0.2471908670705635913, -0.09572725253288331959, 0.02814577918614308283 ) ) ;
#25633=CARTESIAN_POINT ( 'NONE',  ( 0.1264236179284866091, -1.250492125930488196, 0.1264236179284866091 ) ) ;
#25634=CARTESIAN_POINT ( 'NONE',  ( -0.1264236179284866091, -1.412893700733637958, 0.1264236179284866091 ) ) ;
#25640=CARTESIAN_POINT ( 'NONE',  ( -0.1574803149606299191, -0.1850393700787401619, 0.000000000000000000 ) ) ;
#25643=CARTESIAN_POINT ( 'NONE',  ( -0.1787899950787401882, -0.2022637794737956740, 0.000000000000000000 ) ) ;
#25651=ORIENTED_EDGE ( 'NONE', *, *, #45584, .F. ) ;
#25654=CARTESIAN_POINT ( 'NONE',  ( 0.1787899950787401882, -1.594980314906866203, -2.189545951927503898E-17 ) ) ;
#25655=CARTESIAN_POINT ( 'NONE',  ( -0.06523048226347956391, -1.560531495955465253, -0.1574803149606300301 ) ) ;
#25656=CARTESIAN_POINT ( 'NONE',  ( -0.06523048226347956391, -1.009350393593261064, -0.1574803149606300301 ) ) ;
#25657=CARTESIAN_POINT ( 'NONE',  ( 0.1787899950787401882, -0.6943897637257637756, -2.189545951927503898E-17 ) ) ;
#25659=CARTESIAN_POINT ( 'NONE',  ( -0.1574803149606299191, -1.051181102362204856, 0.000000000000000000 ) ) ;
#25669=CARTESIAN_POINT ( 'NONE',  ( -0.06523048226347956391, -1.324311023514519459, -0.1574803149606300301 ) ) ;
#25685=CARTESIAN_POINT ( 'NONE',  ( -0.1585677771909188849, -0.09851383642568464771, -0.08159708949282913626 ) ) ;
#25692=CARTESIAN_POINT ( 'NONE',  ( 0.000000000000000000, 0.000000000000000000, 0.000000000000000000 ) ) ;
#25694=CARTESIAN_POINT ( 'NONE',  ( 0.1787899950787401604, -0.3769685038832444324, -0.07405724077823318263 ) ) ;
#25695=CARTESIAN_POINT ( 'NONE',  ( 3.284318927891251994E-17, -0.8961614172690708369, 0.1787899950787401882 ) ) ;
#25699=CARTESIAN_POINT ( 'NONE',  ( 0.07444174185955065859, -0.1462052269058802256, 0.1797182628040039087 ) ) ;
#25700=CARTESIAN_POINT ( 'NONE',  ( 0.1264236179284866091, -0.1590806611426246187, 0.1264236179284866091 ) ) ;
#25701=CARTESIAN_POINT ( 'NONE',  ( -0.1264236179284866091, -0.3203740156942680994, -0.1264236179284866091 ) ) ;
#25702=CARTESIAN_POINT ( 'NONE',  ( -0.07405724077823318263, -0.1161417322297011862, 0.1787899950787401604 ) ) ;
#25710=CARTESIAN_POINT ( 'NONE',  ( -0.1895013542075498492, -0.07859528327916792678, 0.1760244123200213340 ) ) ;
#25717=CARTESIAN_POINT ( 'NONE',  ( -0.1264236179284866091, -0.3252952755367877757, -0.1264236179284866091 ) ) ;
#25720=CARTESIAN_POINT ( 'NONE',  ( -0.1264236179284866091, -1.137303149552535420, 0.1264236179284866091 ) ) ;
#25738=CARTESIAN_POINT ( 'NONE',  ( -0.1264236179284866091, -0.0004921259304884456750, 0.1264236179284866091 ) ) ;
#25745=( BOUNDED_CURVE ( )  B_SPLINE_CURVE ( 2, ( #35904, #14106, #41118, #21765, #40419, #36849, #29937, #629, #29708 ),
 .UNSPECIFIED., .F., .F. ) 
 B_SPLINE_CURVE_WITH_KNOTS ( ( 3, 2, 2, 2, 3 ),
 ( 0.03500000000000000333, 0.03749999999999999861, 0.04000000000000000083, 0.04250000000000000305, 0.04499999999999999833 ),
 .UNSPECIFIED. ) 
 CURVE ( )  GEOMETRIC_REPRESENTATION_ITEM ( )  RATIONAL_B_SPLINE_CURVE ( ( 1.000000000000000000, 0.9238795325112869605, 1.000000000000000000, 0.9238795325112869605, 1.000000000000000000, 0.9238795325112869605, 1.000000000000000000, 0.9238795325112869605, 1.000000000000000000 ) ) 
 REPRESENTATION_ITEM ( '' )  ) ;
#25748=CARTESIAN_POINT ( 'NONE',  ( 0.1787899950787401604, -1.298352314685932152, 0.07405724077823318263 ) ) ;
#25749=CARTESIAN_POINT ( 'NONE',  ( 0.1787899950787401604, -0.2588582676627719792, 0.07405724077823318263 ) ) ;
#25755=CARTESIAN_POINT ( 'NONE',  ( -0.2471922279628200048, -0.07692167320558097876, 0.07932652958038384494 ) ) ;
#25757=CARTESIAN_POINT ( 'NONE',  ( -0.07405724077823318263, -1.646653543253324026, 0.1787899950787401604 ) ) ;
#25758=B_SPLINE_CURVE_WITH_KNOTS ( 'NONE', 3,
 ( #9979, #12652, #2298, #9028, #5188, #19810, #38499, #16241, #27758, #23652, #5671, #31330, #45908, #13124, #42321, #9513, #24138, #36567, #10941, #29430 ),
 .UNSPECIFIED., .F., .F.,
 ( 4, 1, 1, 1, 1, 1, 2, 2, 1, 1, 1, 2, 2, 4 ),
 ( 0.000000000000000000, 0.2499999999999955591, 0.3749999999999933387, 0.4374999999999921174, 0.4687499999999915068, 0.4843749999999912847, 0.4921874999999911737, 0.4999999999999910072, 0.6249999999999926725, 0.6874999999999935607, 0.7187499999999942268, 0.7343749999999943379, 0.7499999999999945599, 1.000000000000000000 ),
 .UNSPECIFIED. ) ;
#25761=CARTESIAN_POINT ( 'NONE',  ( -0.1270800023317771588, -1.462642234779895745, -0.1270800023317771588 ) ) ;
#25787=CARTESIAN_POINT ( 'NONE',  ( 0.07405724077823318263, -0.1062992125446616531, 0.1787899950787401604 ) ) ;
#25791=CARTESIAN_POINT ( 'NONE',  ( -0.07564704710143098365, -0.08785038237282348506, 0.2417569064347979690 ) ) ;
#25794=CARTESIAN_POINT ( 'NONE',  ( 0.07405724077823318263, -1.804133858213953889, 0.1787899950787401604 ) ) ;
#25802=CARTESIAN_POINT ( 'NONE',  ( -0.1264236179284866091, -0.8382145194103405306, 0.1264236179284866091 ) ) ;
#25804=CARTESIAN_POINT ( 'NONE',  ( 0.1264236179284866091, 0.1422244095025824717, -0.1264236179284866091 ) ) ;
#25805=ORIENTED_EDGE ( 'NONE', *, *, #19690, .T. ) ;
#25812=CARTESIAN_POINT ( 'NONE',  ( -0.1264236179284866091, -0.5221456692375747721, -0.1264236179284866091 ) ) ;
#25814=CARTESIAN_POINT ( 'NONE',  ( -1.100456976456230270E-17, -0.9557524710003681978, -0.1797182628040039365 ) ) ;
#25827=CARTESIAN_POINT ( 'NONE',  ( -1.094772975963752103E-17, -0.8371062991588346103, -0.1787899950787401882 ) ) ;
#25833=CARTESIAN_POINT ( 'NONE',  ( 0.1574803149606299191, -1.622047244094488194, -1.928577636452523993E-17 ) ) ;
#25839=CARTESIAN_POINT ( 'NONE',  ( 0.1787899950787401604, -1.444881889710016631, 0.07405724077823318263 ) ) ;
#25848=CARTESIAN_POINT ( 'NONE',  ( 0.1264236179284866091, -0.3854586138985299226, -0.1264236179284866091 ) ) ;
#25849=CARTESIAN_POINT ( 'NONE',  ( -0.2080960361476567044, -0.08955968088635905822, -0.1267239370720273928 ) ) ;
#25858=CARTESIAN_POINT ( 'NONE',  ( 0.1787899950787401604, -1.405511810969858999, 0.07405724077823318263 ) ) ;
#25859=CARTESIAN_POINT ( 'NONE',  ( 0.07405724077823318263, -1.444881889710016631, 0.1787899950787401604 ) ) ;
#25867=CARTESIAN_POINT ( 'NONE',  ( -0.06523048226347956391, -0.3499015748031495399, -0.1574803149606300301 ) ) ;
#25873=CARTESIAN_POINT ( 'NONE',  ( 2.892866454678787531E-17, -0.5196850392625512738, 0.1574803149606299191 ) ) ;
#25882=CARTESIAN_POINT ( 'NONE',  ( -0.1264236179284866091, -1.609744094434425232, 0.1264236179284866091 ) ) ;
#25883=CARTESIAN_POINT ( 'NONE',  ( 0.1574803149606300301, -1.575295275483024948, 0.06523048226347956391 ) ) ;
#25884=CARTESIAN_POINT ( 'NONE',  ( -0.1787899950787401882, -0.7534448818360000022, 0.000000000000000000 ) ) ;
#25885=CARTESIAN_POINT ( 'NONE',  ( 0.1574803149606300301, -1.265255905511811774, -0.06523048226347956391 ) ) ;
#25901=CARTESIAN_POINT ( 'NONE',  ( 0.06655125492330998815, 0.08353766247256362576, 0.2470096859212614071 ) ) ;
#25915=CARTESIAN_POINT ( 'NONE',  ( -0.07405724077823318263, -0.9576771653005667906, -0.1787899950787401604 ) ) ;
#25916=CARTESIAN_POINT ( 'NONE',  ( -1.094772975963752103E-17, -0.4483267715997795166, -0.1787899950787401882 ) ) ;
#25917=CARTESIAN_POINT ( 'NONE',  ( -0.1787899950787401604, -0.9035433070328510174, 0.07405724077823318263 ) ) ;
#25922=CARTESIAN_POINT ( 'NONE',  ( 0.1797182628040039087, -0.1806540458035179320, 0.07444174185955046430 ) ) ;
#25923=CARTESIAN_POINT ( 'NONE',  ( 0.1574803149606300301, 0.1520669291338582751, -0.06523048226347956391 ) ) ;
#25924=CARTESIAN_POINT ( 'NONE',  ( -0.1787899950787401604, -0.1210629920722208208, 0.07405724077823318263 ) ) ;
#25925=CARTESIAN_POINT ( 'NONE',  ( 0.2471922904502827645, -0.04197619597984889039, -0.1314166662975417565 ) ) ;
#25927=EDGE_CURVE ( 'NONE', #3498, #38566, #45047, .T. ) ;
#25938=CARTESIAN_POINT ( 'NONE',  ( 0.07405724077823318263, -0.3080708660879689087, 0.1787899950787401604 ) ) ;
#25940=CARTESIAN_POINT ( 'NONE',  ( -0.07405724077823318263, -1.149606299158835387, -0.1787899950787401604 ) ) ;
#25949=CARTESIAN_POINT ( 'NONE',  ( 0.1113553986120547346, -1.213582677057826853, -0.1113553986120547346 ) ) ;
#25964=CARTESIAN_POINT ( 'NONE',  ( 0.1264236179284866091, -1.527190897363096544, -0.1264236179284866091 ) ) ;
#25966=CARTESIAN_POINT ( 'NONE',  ( 0.1787899950787401604, -0.3326771653005671237, -0.07405724077823318263 ) ) ;
#25975=CARTESIAN_POINT ( 'NONE',  ( -1.094772975963752103E-17, -1.629429133804503937, -0.1787899950787401882 ) ) ;
#25976=CARTESIAN_POINT ( 'NONE',  ( -1.094772975963752103E-17, -1.663877952702141672, -0.1787899950787401882 ) ) ;
#25982=CARTESIAN_POINT ( 'NONE',  ( 0.1797182628040039087, -1.361756408008243824, 0.07444174185955046430 ) ) ;
#25992=CARTESIAN_POINT ( 'NONE',  ( -0.06523048226347956391, -0.8124999998924731237, -0.1574803149606300301 ) ) ;
#26006=CARTESIAN_POINT ( 'NONE',  ( 0.1270800023317771588, -0.1043745182444627967, 0.1270800023317771588 ) ) ;
#26016=CARTESIAN_POINT ( 'NONE',  ( 0.1264236179284866091, -0.1432086613635592531, 0.1264236179284866091 ) ) ;
#26023=CARTESIAN_POINT ( 'NONE',  ( 0.1113553986120547346, 0.08562992136736949367, -0.1113553986120547346 ) ) ;
#26031=CARTESIAN_POINT ( 'NONE',  ( 0.1264236179284866091, -0.7890019209851437676, 0.1264236179284866091 ) ) ;
#26042=CARTESIAN_POINT ( 'NONE',  ( -0.1787899950787401604, -0.5196850393163150450, -0.07405724077823318263 ) ) ;
#26048=CARTESIAN_POINT ( 'NONE',  ( -0.1797182628040039365, -1.064020187535801298, 0.000000000000000000 ) ) ;
#26060=CARTESIAN_POINT ( 'NONE',  ( -1.094772975963752103E-17, -0.7189960629383621571, -0.1787899950787401882 ) ) ;
#26062=FACE_OUTER_BOUND ( 'NONE', #9711, .T. ) ;
#26066=CARTESIAN_POINT ( 'NONE',  ( -0.1574803149606299191, -1.681102362204724532, 0.000000000000000000 ) ) ;
#26072=CARTESIAN_POINT ( 'NONE',  ( -0.06523048226347956391, -0.2859251967428664831, 0.1574803149606297803 ) ) ;
#26079=CARTESIAN_POINT ( 'NONE',  ( 0.1121631700669272619, 0.09842519685039372024, -0.2206756344348396182 ) ) ;
#26081=CARTESIAN_POINT ( 'NONE',  ( 0.1787899950787401882, -0.3510097950008925216, -2.189545951927503898E-17 ) ) ;
#26082=CARTESIAN_POINT ( 'NONE',  ( 0.07338256679960847295, -0.09842519685039370636, 0.1314280838991750133 ) ) ;
#26091=B_SPLINE_CURVE_WITH_KNOTS ( 'NONE', 3,
 ( #38866, #9884, #36242, #28590, #39328, #32420, #6504, #3628, #40031, #14190, #40268, #32658, #46996, #7453, #7, #14658, #39790, #21849, #6984, #7226, #43154 ),
 .UNSPECIFIED., .F., .F.,
 ( 4, 2, 1, 1, 2, 2, 2, 1, 1, 1, 2, 2, 4 ),
 ( 0.000000000000000000, 0.1250000000000001388, 0.1875000000000001665, 0.2187500000000002498, 0.2343750000000003053, 0.2500000000000003886, 0.3750000000000004996, 0.4375000000000004996, 0.4687500000000004996, 0.4843750000000006106, 0.4921875000000006661, 0.5000000000000006661, 1.000000000000000000 ),
 .UNSPECIFIED. ) ;
#26097=CARTESIAN_POINT ( 'NONE',  ( 0.07405724077823318263, -1.277559055064345861, -0.1787899950787401604 ) ) ;
#26098=CARTESIAN_POINT ( 'NONE',  ( -0.07405724077823318263, -1.464566929080096225, -0.1787899950787401604 ) ) ;
#26105=CARTESIAN_POINT ( 'NONE',  ( -0.06523048226347956391, -0.2711614173228347746, -0.1574803149606300301 ) ) ;
#26113=CONICAL_SURFACE ( 'NONE', #5436, 0.2471922904502826812, 0.5235987755982992597 ) ;
#26115=CARTESIAN_POINT ( 'NONE',  ( -0.1696281918730704608, -0.08954833399976612485, -0.01761539643617799841 ) ) ;
#26123=CARTESIAN_POINT ( 'NONE',  ( -0.1264236179284866091, -1.501476377898992354, -0.1264236179284866091 ) ) ;
#26124=CARTESIAN_POINT ( 'NONE',  ( -1.094772975963752103E-17, -0.7632874015210393548, -0.1787899950787401882 ) ) ;
#26126=CARTESIAN_POINT ( 'NONE',  ( -0.1574803149606297803, -1.245570866141732624, 0.06523048226347956391 ) ) ;
#26135=CARTESIAN_POINT ( 'NONE',  ( -0.1574803149606300301, -1.319389763671999782, -0.06523048226347956391 ) ) ;
#26149=CARTESIAN_POINT ( 'NONE',  ( -0.1602016258198147580, -0.09842519685039370636, -0.1931405315332122008 ) ) ;
#26156=EDGE_LOOP ( 'NONE', ( #1024, #4280, #17329 ) ) ;
#26160=CARTESIAN_POINT ( 'NONE',  ( 0.1264236179284866091, -0.8863188975840314843, -0.1264236179284866091 ) ) ;
#26161=CARTESIAN_POINT ( 'NONE',  ( 0.1264236179284866091, -0.4630905511273386010, 0.1264236179284866091 ) ) ;
#26162=CARTESIAN_POINT ( 'NONE',  ( -0.07405724077823318263, -1.134842519631275914, 0.1787899950787401604 ) ) ;
#26166=CARTESIAN_POINT ( 'NONE',  ( -0.07444174185955065859, -0.3233705812365890719, -0.1797182628040039087 ) ) ;
#26168=CARTESIAN_POINT ( 'NONE',  ( -0.1264236179284866091, -0.03986220467064590517, 0.1264236179284866091 ) ) ;
#26172=( LENGTH_UNIT ( ) NAMED_UNIT ( * ) SI_UNIT ( $, .METRE. ) ) ;
#26173=PLANE ( 'NONE',  #4270 ) ;
#26178=ORIENTED_EDGE ( 'NONE', *, *, #35766, .T. ) ;
#26182=CARTESIAN_POINT ( 'NONE',  ( 0.1574803149606300301, -0.9404527557979834862, -0.06523048226347956391 ) ) ;
#26183=CARTESIAN_POINT ( 'NONE',  ( -0.1787899950787401604, -0.2391732282926934683, 0.07405724077823318263 ) ) ;
#26185=CARTESIAN_POINT ( 'NONE',  ( 0.1264236179284866091, -1.166830708607653477, 0.1264236179284866091 ) ) ;
#26198=CARTESIAN_POINT ( 'NONE',  ( -0.09591045553298832571, -0.09842280622452256877, -0.1509607186031187431 ) ) ;
#26214=CARTESIAN_POINT ( 'NONE',  ( -0.1264236179284866091, -1.389395621772545608, 0.1264236179284866091 ) ) ;
#26216=CARTESIAN_POINT ( 'NONE',  ( -0.1787899950787401604, -0.4360236219934807145, -0.07405724077823318263 ) ) ;
#26226=CARTESIAN_POINT ( 'NONE',  ( -0.07405724077823318263, -1.784448818843874962, -0.1787899950787401604 ) ) ;
#26227=CARTESIAN_POINT ( 'NONE',  ( 3.284318927891251994E-17, -1.683562992072220599, 0.1787899950787401882 ) ) ;
#26232=CARTESIAN_POINT ( 'NONE',  ( -0.1113553986120547346, -0.7706692913385826404, 0.1113553986120547346 ) ) ;
#26233=CARTESIAN_POINT ( 'NONE',  ( -0.1797182628040039365, -1.418350896197218436, 0.000000000000000000 ) ) ;
#26240=DIRECTION ( 'NONE',  ( 0.000000000000000000, 1.000000000000000000, 0.000000000000000000 ) ) ;
#26253=CARTESIAN_POINT ( 'NONE',  ( 0.07444174185955046430, -0.05270128989800624414, -0.1797182628040039087 ) ) ;
#26255=CARTESIAN_POINT ( 'NONE',  ( -0.07405724077823318263, -1.257874015694269376, 0.1787899950787401604 ) ) ;
#26264=CARTESIAN_POINT ( 'NONE',  ( -0.1787899950787401604, -0.1161417322297011862, 0.07405724077823318263 ) ) ;
#26267=CARTESIAN_POINT ( 'NONE',  ( -0.1574803149606297803, 0.09301181102362202080, 0.06523048226347956391 ) ) ;
#26268=CARTESIAN_POINT ( 'NONE',  ( 0.2088134963345943673, -0.06712557525760230737, -0.1648743713627059404 ) ) ;
#26272=CARTESIAN_POINT ( 'NONE',  ( -0.06523048226347956391, -0.1038385825696382520, -0.1574803149606300301 ) ) ;
#26279=CARTESIAN_POINT ( 'NONE',  ( 0.000000000000000000, -0.09842519685039370636, 0.000000000000000000 ) ) ;
#26281=CARTESIAN_POINT ( 'NONE',  ( 0.1787899950787401604, -0.9784704249221527483, -0.07405724077823318263 ) ) ;
#26284=CARTESIAN_POINT ( 'NONE',  ( 0.07405724077823318263, 0.02657480320336980464, -0.1787899950787401604 ) ) ;
#26291=CARTESIAN_POINT ( 'NONE',  ( -0.1264236179284866091, -0.4729330708123779536, 0.1264236179284866091 ) ) ;
#26296=CARTESIAN_POINT ( 'NONE',  ( 0.1797182628040039365, -1.004965069425564961, -2.200913952912460540E-17 ) ) ;
#26306=CARTESIAN_POINT ( 'NONE',  ( -0.1574803149606300301, -0.6894685038294798840, -0.06523048226347956391 ) ) ;
#26310=CARTESIAN_POINT ( 'NONE',  ( 0.1787899950787401604, -0.7312992125446612368, 0.07405724077823318263 ) ) ;
#26315=ADVANCED_FACE ( 'NONE', ( #30098 ), #4158, .T. ) ;
#26317=CARTESIAN_POINT ( 'NONE',  ( -0.06523048226347956391, -1.713090551181103649, 0.1574803149606297803 ) ) ;
#26325=CARTESIAN_POINT ( 'NONE',  ( 0.1574803149606300301, 0.1126968503937008370, -0.06523048226347956391 ) ) ;
#26326=CARTESIAN_POINT ( 'NONE',  ( 0.06523048226347956391, -0.3203740156405044948, 0.1574803149606297803 ) ) ;
#26334=CARTESIAN_POINT ( 'NONE',  ( -0.1787899950787401604, -0.6093759367331758048, -0.07405724077823318263 ) ) ;
#26335=CARTESIAN_POINT ( 'NONE',  ( -0.06320621770493051184, -0.08956000428219212939, 0.2147707455372145635 ) ) ;
#26339=CARTESIAN_POINT ( 'NONE',  ( 0.1787899950787401604, -1.770793259567822853, 0.07405724077823318263 ) ) ;
#26341=CARTESIAN_POINT ( 'NONE',  ( 0.2471911544649836034, -0.08539615244825589369, 0.06152421978428734145 ) ) ;
#26344=CARTESIAN_POINT ( 'NONE',  ( -0.1787899950787401882, -1.343996062938362268, 0.000000000000000000 ) ) ;
#26345=CARTESIAN_POINT ( 'NONE',  ( 3.284318927891251994E-17, -1.604822834591905556, 0.1787899950787401882 ) ) ;
#26353=CARTESIAN_POINT ( 'NONE',  ( -0.1574803149606297803, -0.3006889763779526104, 0.06523048226347956391 ) ) ;
#26362=CARTESIAN_POINT ( 'NONE',  ( -0.1560601414942001663, -0.08956156883362471899, 0.05573596787081475795 ) ) ;
#26370=CARTESIAN_POINT ( 'NONE',  ( 0.1787899950787401882, -1.516240157426551161, -2.189545951927503898E-17 ) ) ;
#26371=CARTESIAN_POINT ( 'NONE',  ( 3.284318927891251994E-17, -0.9010826771115905132, 0.1787899950787401882 ) ) ;
#26372=CARTESIAN_POINT ( 'NONE',  ( 0.06523048226347956391, -1.156988188976378229, 0.1574803149606297803 ) ) ;
#26383=EDGE_CURVE ( 'NONE', #36909, #11736, #44722, .T. ) ;
#26394=CARTESIAN_POINT ( 'NONE',  ( -0.04623149810832708623, -0.09851382820108051108, 0.1526845614456639744 ) ) ;
#26402=CARTESIAN_POINT ( 'NONE',  ( 0.07405724077823318263, -0.8444881889226140137, -0.1787899950787401604 ) ) ;
#26403=CARTESIAN_POINT ( 'NONE',  ( 0.1787899950787401604, -1.041338582623402287, -0.07405724077823318263 ) ) ;
#26406=CARTESIAN_POINT ( 'NONE',  ( 0.07444174185955046430, -0.2889217623389510603, -0.1797182628040039087 ) ) ;
#26407=CARTESIAN_POINT ( 'NONE',  ( 0.06523048226347956391, 0.1176181102362205133, -0.1574803149606300301 ) ) ;
#26408=CARTESIAN_POINT ( 'NONE',  ( -0.1787899950787401604, -0.04724409443442544737, -0.07405724077823318263 ) ) ;
#26411=( BOUNDED_CURVE ( )  B_SPLINE_CURVE ( 2, ( #36201, #14619, #46962, #211, #32853, #29521, #14861, #35948, #14150 ),
 .UNSPECIFIED., .F., .T. ) 
 B_SPLINE_CURVE_WITH_KNOTS ( ( 3, 2, 2, 2, 3 ),
 ( 0.01499999999999999944, 0.01750000000000000167, 0.02000000000000000042, 0.02249999999999999917, 0.02500000000000000139 ),
 .UNSPECIFIED. ) 
 CURVE ( )  GEOMETRIC_REPRESENTATION_ITEM ( )  RATIONAL_B_SPLINE_CURVE ( ( 1.000000000000000000, 0.9238795325112869605, 1.000000000000000000, 0.9238795325112869605, 1.000000000000000000, 0.9238795325112869605, 1.000000000000000000, 0.9238795325112869605, 1.000000000000000000 ) ) 
 REPRESENTATION_ITEM ( '' )  ) ;
#26413=CARTESIAN_POINT ( 'NONE',  ( 0.000000000000000000, 0.09842519685039370636, 0.000000000000000000 ) ) ;
#26419=CARTESIAN_POINT ( 'NONE',  ( 0.1113553986120547346, -0.9478346455617638888, 0.1113553986120547346 ) ) ;
#26420=CARTESIAN_POINT ( 'NONE',  ( -0.1264236179284866091, -0.1973425196312759700, 0.1264236179284866091 ) ) ;
#26422=CARTESIAN_POINT ( 'NONE',  ( -0.1787899950787401604, -1.262795275536788386, -0.07405724077823318263 ) ) ;
#26431=TOROIDAL_SURFACE ( 'NONE', #21026, 0.2007874015748031815, 0.01968503937007873988 ) ;
#26436=CARTESIAN_POINT ( 'NONE',  ( -0.1192973132712141088, -0.09842522298280542703, -0.1331694143430761090 ) ) ;
#26441=CARTESIAN_POINT ( 'NONE',  ( -0.1787899950787401604, -0.08661417317458304510, -0.07405724077823318263 ) ) ;
#26444=CARTESIAN_POINT ( 'NONE',  ( -0.2006330517481570708, -0.09851385263128563385, -0.1463975219237275693 ) ) ;
#26449=CARTESIAN_POINT ( 'NONE',  ( 0.1787899950787401882, -1.453371999725301178, -2.189545951927503898E-17 ) ) ;
#26452=CARTESIAN_POINT ( 'NONE',  ( -0.1787899950787401604, -0.4753937007336378473, -0.07405724077823318263 ) ) ;
#26460=CARTESIAN_POINT ( 'NONE',  ( -0.1264236179284866091, -0.2465551180564728440, -0.1264236179284866091 ) ) ;
#26465=CARTESIAN_POINT ( 'NONE',  ( 0.07405724077823318263, 0.1288130396447769721, -0.1787899950787401604 ) ) ;
#26466=CARTESIAN_POINT ( 'NONE',  ( -0.1787899950787401604, -1.730314960576156968, 0.07405724077823318263 ) ) ;
#26469=CARTESIAN_POINT ( 'NONE',  ( 0.1574803149606300301, -0.7140748031496056969, -0.06523048226347956391 ) ) ;
#26471=CARTESIAN_POINT ( 'NONE',  ( -0.07444174185955065859, -1.465102864701155916, -0.1797182628040039087 ) ) ;
#26472=CARTESIAN_POINT ( 'NONE',  ( -0.1113553986120547346, -0.05216535422318158144, 0.1113553986120547346 ) ) ;
#26478=CARTESIAN_POINT ( 'NONE',  ( 0.06523048226347956391, -0.8174212597349923559, -0.1574803149606300301 ) ) ;
#26490=ORIENTED_EDGE ( 'NONE', *, *, #27645, .F. ) ;
#26491=CARTESIAN_POINT ( 'NONE',  ( -0.1270800023317771588, -0.08468947887438406374, -0.1270800023317771588 ) ) ;
#26492=CARTESIAN_POINT ( 'NONE',  ( 3.284318927891251994E-17, -1.216043307032850462, 0.1787899950787401882 ) ) ;
#26497=EDGE_CURVE ( 'NONE', #33652, #33104, #44019, .T. ) ;
#26499=CARTESIAN_POINT ( 'NONE',  ( -0.1574803149606299191, 0.05118110236220472370, 0.000000000000000000 ) ) ;
#26503=CARTESIAN_POINT ( 'NONE',  ( -0.07405724077823318263, -0.1899606298674962612, 0.1787899950787401604 ) ) ;
#26507=CARTESIAN_POINT ( 'NONE',  ( 0.1574803149606300301, -0.1186023620971974196, 0.06523048226347956391 ) ) ;
#26513=CARTESIAN_POINT ( 'NONE',  ( -0.07405724077823318263, -0.9538641257095545889, 0.1787899950787401604 ) ) ;
#26515=CARTESIAN_POINT ( 'NONE',  ( -1.094772975963752103E-17, 0.06840551186478720236, -0.1787899950787401882 ) ) ;
#26527=CARTESIAN_POINT ( 'NONE',  ( 0.1270800023317771588, -1.078783967063360327, -0.1270800023317771588 ) ) ;
#26528=CARTESIAN_POINT ( 'NONE',  ( 0.1372385047410485115, 0.1299212598425196485, -0.09687705708535346294 ) ) ;
#26535=CARTESIAN_POINT ( 'NONE',  ( 0.1321676148590689159, 0.1299212598425196763, -0.1026092226670043267 ) ) ;
#26542=CARTESIAN_POINT ( 'NONE',  ( -0.1787899950787401604, -0.7854330708123791194, 0.07405724077823318263 ) ) ;
#26551=CARTESIAN_POINT ( 'NONE',  ( -9.642888182262618425E-18, -1.730314960629921517, -0.1574803149606299191 ) ) ;
#26554=EDGE_CURVE ( 'NONE', #3517, #37608, #30628, .T. ) ;
#26560=CARTESIAN_POINT ( 'NONE',  ( 0.1264236179284866091, -1.555610236166708571, -0.1264236179284866091 ) ) ;
#26561=B_SPLINE_CURVE_WITH_KNOTS ( 'NONE', 3,
 ( #2599, #21048, #14115, #36403, #17232, #17929, #10288, #32815, #46448, #24897, #24425, #14581, #3561, #39026, #13630, #43328, #42832, #35910, #6194, #32584 ),
 .UNSPECIFIED., .F., .F.,
 ( 4, 1, 1, 1, 1, 1, 2, 2, 1, 1, 1, 2, 2, 4 ),
 ( 0.000000000000000000, 0.2499999999999993894, 0.3749999999999990008, 0.4374999999999987788, 0.4687499999999986122, 0.4843749999999986122, 0.4921874999999985012, 0.4999999999999984457, 0.6249999999999980016, 0.6874999999999978906, 0.7187499999999977796, 0.7343749999999978906, 0.7499999999999980016, 1.000000000000000000 ),
 .UNSPECIFIED. ) ;
#26569=CARTESIAN_POINT ( 'NONE',  ( -0.1787899950787401604, -0.4912657005127034071, -0.07405724077823318263 ) ) ;
#26570=CARTESIAN_POINT ( 'NONE',  ( 0.05749879812895779263, -0.08956009822529961695, 0.2100333487722925163 ) ) ;
#26575=CARTESIAN_POINT ( 'NONE',  ( 0.1787899950787401604, -1.805242078465460809, -0.07405724077823318263 ) ) ;
#26581=CARTESIAN_POINT ( 'NONE',  ( -0.1787899950787401882, -1.265255905458047225, 0.000000000000000000 ) ) ;
#26582=CARTESIAN_POINT ( 'NONE',  ( -1.094772975963752103E-17, -1.545767716481669218, -0.1787899950787401882 ) ) ;
#26590=ADVANCED_FACE ( 'NONE', ( #36194 ), #10800, .F. ) ;
#26600=CARTESIAN_POINT ( 'NONE',  ( -0.1690299954235125468, -0.08956068868289060458, -0.02622682328975086199 ) ) ;
#26605=ORIENTED_EDGE ( 'NONE', *, *, #16090, .T. ) ;
#26608=CARTESIAN_POINT ( 'NONE',  ( -0.1787899950787401604, -1.617125984198204414, -0.07405724077823318263 ) ) ;
#26609=CARTESIAN_POINT ( 'NONE',  ( 0.07405724077823318263, -0.8838582676627719792, -0.1787899950787401604 ) ) ;
#26610=CARTESIAN_POINT ( 'NONE',  ( -0.06523048226347956391, -1.176673228346457156, -0.1574803149606300301 ) ) ;
#26624=CARTESIAN_POINT ( 'NONE',  ( 0.09934514972678533395, 0.09575019180979006672, 0.2280761219286985830 ) ) ;
#26631=CARTESIAN_POINT ( 'NONE',  ( -0.2232765723780838485, -0.09842519685039370636, 0.08144284342645886909 ) ) ;
#26640=CARTESIAN_POINT ( 'NONE',  ( 0.1787899950787401604, -0.9281496062454495100, -0.07405724077823318263 ) ) ;
#26642=CARTESIAN_POINT ( 'NONE',  ( 0.1264236179284866091, -1.038877952702141672, -0.1264236179284866091 ) ) ;
#26646=CARTESIAN_POINT ( 'NONE',  ( -0.1797182628040039087, -0.3578194001342265285, -0.07444174185955065859 ) ) ;
#26653=DIRECTION ( 'NONE',  ( -0.8660254037844388186, 0.000000000000000000, 0.4999999999999998890 ) ) ;
#26659=CARTESIAN_POINT ( 'NONE',  ( -0.1264236179284866091, -0.3646653542769452971, -0.1264236179284866091 ) ) ;
#26661=CARTESIAN_POINT ( 'NONE',  ( 0.1787899950787401882, -1.161909448765133801, -2.189545951927503898E-17 ) ) ;
#26683=ORIENTED_EDGE ( 'NONE', *, *, #41904, .F. ) ;
#26687=CARTESIAN_POINT ( 'NONE',  ( 3.284318927891251994E-17, -1.423844440670183120, 0.1787899950787401882 ) ) ;
#26689=CARTESIAN_POINT ( 'NONE',  ( 0.07405724077823318263, -0.4458661416785199560, -0.1787899950787401604 ) ) ;
#26698=CARTESIAN_POINT ( 'NONE',  ( 0.1787899950787401882, -1.718011810969858333, -2.189545951927503898E-17 ) ) ;
#26699=CARTESIAN_POINT ( 'NONE',  ( 0.1264236179284866091, -1.786909448765134023, -0.1264236179284866091 ) ) ;
#26705=CARTESIAN_POINT ( 'NONE',  ( -0.06523048226347956391, -0.7288385826771652809, 0.1574803149606297803 ) ) ;
#26707=CARTESIAN_POINT ( 'NONE',  ( 0.1797182628040039365, -1.477406014307454774, -2.200913952912460540E-17 ) ) ;
#26717=CARTESIAN_POINT ( 'NONE',  ( -1.094772975963752103E-17, 0.06348425202226751218, -0.1787899950787401882 ) ) ;
#26731=CARTESIAN_POINT ( 'NONE',  ( 0.1797182628040039087, -0.01825247100036840597, -0.07444174185955065859 ) ) ;
#26732=CARTESIAN_POINT ( 'NONE',  ( -0.1264236179284866091, -1.191437007820251859, -0.1264236179284866091 ) ) ;
#26741=CARTESIAN_POINT ( 'NONE',  ( 0.06523048226347956391, -0.005413385719244615847, 0.1574803149606297803 ) ) ;
#26748=CARTESIAN_POINT ( 'NONE',  ( 0.1787899950787401882, -1.059671212323726408, -2.189545951927503898E-17 ) ) ;
#26750=CARTESIAN_POINT ( 'NONE',  ( -0.1787899950787401882, 0.07824803154982658271, 0.000000000000000000 ) ) ;
#26759=CARTESIAN_POINT ( 'NONE',  ( -0.1787899950787401882, -0.6353346456155275490, 0.000000000000000000 ) ) ;
#26764=CARTESIAN_POINT ( 'NONE',  ( -0.1270800023317771588, -0.9902012898980059319, -0.1270800023317771588 ) ) ;
#26772=CARTESIAN_POINT ( 'NONE',  ( -0.1264236179284866091, 0.08316929139234625901, 0.1264236179284866091 ) ) ;
#26778=CARTESIAN_POINT ( 'NONE',  ( -1.094772975963752103E-17, -0.9158464566391496531, -0.1787899950787401882 ) ) ;
#26779=VERTEX_POINT ( 'NONE', #22028 ) ;
#26781=CARTESIAN_POINT ( 'NONE',  ( -0.1113553986120547346, -1.754921259734992134, -0.1113553986120547346 ) ) ;
#26785=CARTESIAN_POINT ( 'NONE',  ( 0.1113553986120547346, -1.735236220472441193, -0.1113553986120547346 ) ) ;
#26792=CARTESIAN_POINT ( 'NONE',  ( 0.1787899950787401882, -1.481791338528913426, -2.189545951927503898E-17 ) ) ;
#26796=CARTESIAN_POINT ( 'NONE',  ( 0.1113553986120547346, -0.04232283453814220803, 0.1113553986120547346 ) ) ;
#26800=CARTESIAN_POINT ( 'NONE',  ( 0.1787899950787401604, -0.5896908973630964335, 0.07405724077823318263 ) ) ;
#26801=CARTESIAN_POINT ( 'NONE',  ( -0.05328757346823071589, -0.08955999039829311281, 0.2169276614305941098 ) ) ;
#26813=CARTESIAN_POINT ( 'NONE',  ( -1.094772975963752103E-17, -1.393208661363559031, -0.1787899950787401882 ) ) ;
#26815=CARTESIAN_POINT ( 'NONE',  ( -0.1264236179284866091, -1.531003936954110189, 0.1264236179284866091 ) ) ;
#26823=CARTESIAN_POINT ( 'NONE',  ( -0.1113553986120547346, -0.3375984251968503491, 0.1113553986120547346 ) ) ;
#26831=CARTESIAN_POINT ( 'NONE',  ( -9.642888182262618425E-18, -0.5393700786326299790, -0.1574803149606299191 ) ) ;
#26834=CARTESIAN_POINT ( 'NONE',  ( -0.1027821604407747752, -0.08956149871714005894, 0.1226111552267875882 ) ) ;
#26840=CARTESIAN_POINT ( 'NONE',  ( -0.1574803149606297803, -0.02509842519685037340, 0.06523048226347956391 ) ) ;
#26841=CARTESIAN_POINT ( 'NONE',  ( -0.1787899950787401604, -1.656496062938362268, -0.07405724077823318263 ) ) ;
#26842=CARTESIAN_POINT ( 'NONE',  ( -0.07405724077823318263, -0.9183070865604088251, -0.1787899950787401604 ) ) ;
#26843=CARTESIAN_POINT ( 'NONE',  ( -0.1574803149606299191, -1.248031496062992129, 0.000000000000000000 ) ) ;
#26845=EDGE_CURVE ( 'NONE', #36464, #47458, #28210, .T. ) ;
#26848=UNCERTAINTY_MEASURE_WITH_UNIT (LENGTH_MEASURE( 1.000000000000000082E-05 ), #44575, 'distance_accuracy_value', 'NONE') ;
#26867=CARTESIAN_POINT ( 'NONE',  ( -0.2086866875178732261, -0.09842519685039370636, -0.1330263174222271749 ) ) ;
#26873=CARTESIAN_POINT ( 'NONE',  ( 3.284318927891251994E-17, -0.8617125983714329918, 0.1787899950787401882 ) ) ;
#26874=CARTESIAN_POINT ( 'NONE',  ( 0.1787899950787401604, -1.120078740103715997, -0.07405724077823318263 ) ) ;
#26879=CARTESIAN_POINT ( 'NONE',  ( -0.1270800023317771588, -0.3898075891106047575, 0.1270800023317771588 ) ) ;
#26880=CARTESIAN_POINT ( 'NONE',  ( 0.1113553986120547346, 0.1053149606299212532, 0.1113553986120547346 ) ) ;
#26889=CARTESIAN_POINT ( 'NONE',  ( 0.000000000000000000, 0.09842519685039370636, 0.000000000000000000 ) ) ;
#26890=CARTESIAN_POINT ( 'NONE',  ( 0.06523048226347956391, -0.9896653542231822476, 0.1574803149606297803 ) ) ;
#26891=CARTESIAN_POINT ( 'NONE',  ( 0.07405724077823318263, -0.4261811023084413064, 0.1787899950787401604 ) ) ;
#26893=CARTESIAN_POINT ( 'NONE',  ( 0.1787899950787401604, -1.243110236166709459, 0.07405724077823318263 ) ) ;
#26903=CARTESIAN_POINT ( 'NONE',  ( -0.1190585826237822442, -0.09842520615623508162, -0.1333826362739909122 ) ) ;
#26904=CARTESIAN_POINT ( 'NONE',  ( 2.892866454678787531E-17, 0.06102362204724409711, 0.1574803149606299191 ) ) ;
#26917=CIRCLE ( 'NONE', #22300, 0.2471922904502826812 ) ;
#26925=CARTESIAN_POINT ( 'NONE',  ( -0.07405724077823318263, -1.480438928859160619, -0.1787899950787401604 ) ) ;
#26926=ORIENTED_EDGE ( 'NONE', *, *, #6371, .F. ) ;
#26927=CARTESIAN_POINT ( 'NONE',  ( -0.1787899950787401882, -0.4729330708123779536, 0.000000000000000000 ) ) ;
#26936=CARTESIAN_POINT ( 'NONE',  ( 0.07405724077823318263, -1.710629921206078041, -0.1787899950787401604 ) ) ;
#26940=CARTESIAN_POINT ( 'NONE',  ( 0.1113553986120547346, -0.7116141732283465249, -0.1113553986120547346 ) ) ;
#26942=CARTESIAN_POINT ( 'NONE',  ( 0.1270800023317771588, -1.590594990685407328, -0.1270800023317771588 ) ) ;
#26951=DIRECTION ( 'NONE',  ( 0.000000000000000000, 1.000000000000000000, 0.000000000000000000 ) ) ;
#26955=CARTESIAN_POINT ( 'NONE',  ( 0.1113553986120547346, -0.8592519683964094934, -0.1113553986120547346 ) ) ;
#26956=CARTESIAN_POINT ( 'NONE',  ( 0.1264236179284866091, 0.09793307091990532953, -0.1264236179284866091 ) ) ;
#26977=ORIENTED_EDGE ( 'NONE', *, *, #21262, .T. ) ;
#26979=CARTESIAN_POINT ( 'NONE',  ( -0.03598878106637547203, -0.09842522444525984848, 0.1542999736886214723 ) ) ;
#26983=CARTESIAN_POINT ( 'NONE',  ( -0.1574803149606297803, -0.05462598414444141265, 0.06523048226347956391 ) ) ;
#26985=VERTEX_POINT ( 'NONE', #20088 ) ;
#26994=CARTESIAN_POINT ( 'NONE',  ( 3.284318927891251994E-17, -1.030143653268608128, 0.1787899950787401882 ) ) ;
#26996=CARTESIAN_POINT ( 'NONE',  ( -0.1264236179284866091, -0.005413385773008149403, -0.1264236179284866091 ) ) ;
#27001=DIRECTION ( 'NONE',  ( 0.000000000000000000, 1.000000000000000000, 0.000000000000000000 ) ) ;
#27002=CARTESIAN_POINT ( 'NONE',  ( 0.07405724077823318263, -0.6476377952218281830, -0.1787899950787401604 ) ) ;
#27008=CARTESIAN_POINT ( 'NONE',  ( 0.1270800023317771588, -1.088626486748399680, 0.1270800023317771588 ) ) ;
#27009=CARTESIAN_POINT ( 'NONE',  ( 0.1442072231542519400, 0.1299212598425196763, -0.08784906043161684608 ) ) ;
#27013=DIRECTION ( 'NONE',  ( 0.000000000000000000, 1.000000000000000000, 0.000000000000000000 ) ) ;
#27024=CARTESIAN_POINT ( 'NONE',  ( 0.000000000000000000, -0.09842519685039370636, 0.000000000000000000 ) ) ;
#27028=CARTESIAN_POINT ( 'NONE',  ( -0.1574803149606299191, -1.671259842412157415, 0.000000000000000000 ) ) ;
#27032=CARTESIAN_POINT ( 'NONE',  ( -0.1574803149606297803, -1.757381889763778959, 0.06523048226347956391 ) ) ;
#27033=DIRECTION ( 'NONE',  ( 0.000000000000000000, -1.000000000000000000, 0.000000000000000000 ) ) ;
#27039=CARTESIAN_POINT ( 'NONE',  ( -0.1113553986120547346, -0.3671259841444414196, 0.1113553986120547346 ) ) ;
#27040=CARTESIAN_POINT ( 'NONE',  ( 0.1264236179284866091, -1.604822834591905556, 0.1264236179284866091 ) ) ;
#27046=CARTESIAN_POINT ( 'NONE',  ( -0.1787899950787401882, -0.5281751493316008128, 0.000000000000000000 ) ) ;
#27047=CARTESIAN_POINT ( 'NONE',  ( 0.1549696564520381958, -0.08956042623435592209, -0.1209032005300702678 ) ) ;
#27055=CARTESIAN_POINT ( 'NONE',  ( 0.2471918495545273320, -0.09442133267706712130, 0.03395794428076722576 ) ) ;
#27057=CARTESIAN_POINT ( 'NONE',  ( 0.1264236179284866091, -1.565452755851747924, 0.1264236179284866091 ) ) ;
#27059=CARTESIAN_POINT ( 'NONE',  ( -0.1787899950787401604, -1.612204724355685403, 0.07405724077823318263 ) ) ;
#27068=CARTESIAN_POINT ( 'NONE',  ( -0.1113553986120547346, -0.4655511811023622104, -0.1113553986120547346 ) ) ;
#27080=CARTESIAN_POINT ( 'NONE',  ( -0.1787899950787401882, -0.5516732282926929409, 0.000000000000000000 ) ) ;
#27089=CARTESIAN_POINT ( 'NONE',  ( -0.1264236179284866091, -1.649114173174582643, 0.1264236179284866091 ) ) ;
#27090=CARTESIAN_POINT ( 'NONE',  ( -1.094772975963752103E-17, -0.8813976377415118080, -0.1787899950787401882 ) ) ;
#27091=CARTESIAN_POINT ( 'NONE',  ( -0.06523048226347956391, -1.294783464566929165, -0.1574803149606300301 ) ) ;
#27101=CARTESIAN_POINT ( 'NONE',  ( 0.06523048226347956391, -1.383366141624756018, 0.1574803149606297803 ) ) ;
#27104=CARTESIAN_POINT ( 'NONE',  ( 0.06523048226347956391, -0.005413385719244616714, 0.1574803149606297803 ) ) ;
#27118=CARTESIAN_POINT ( 'NONE',  ( 0.2071770260006893793, -0.09842519685039370636, -0.0004133995244056677112 ) ) ;
#27122=CARTESIAN_POINT ( 'NONE',  ( 0.1264236179284866091, -1.004429133804503937, -0.1264236179284866091 ) ) ;
#27124=CARTESIAN_POINT ( 'NONE',  ( 0.07405724077823318263, -1.115157480261196987, -0.1787899950787401604 ) ) ;
#27127=CARTESIAN_POINT ( 'NONE',  ( 0.1797182628040039365, -0.4144138883232031390, -2.200913952912460540E-17 ) ) ;
#27129=CARTESIAN_POINT ( 'NONE',  ( -0.06523048226347956391, 0.01919291338582680348, 0.1574803149606297803 ) ) ;
#27131=CARTESIAN_POINT ( 'NONE',  ( -0.07405724077823318263, -0.1702755904974175283, -0.1787899950787401604 ) ) ;
#27141=CARTESIAN_POINT ( 'NONE',  ( -0.1264236179284866091, -0.4729330708123779536, 0.1264236179284866091 ) ) ;
#27152=CARTESIAN_POINT ( 'NONE',  ( 0.03914454236661495806, -0.09842447277515208037, -0.1744522088443405949 ) ) ;
#27157=CARTESIAN_POINT ( 'NONE',  ( 0.1878058820402545848, -0.07958416565541145959, -0.1770032286854512915 ) ) ;
#27172=CARTESIAN_POINT ( 'NONE',  ( -0.1264236179284866091, -0.4680118109698582773, 0.1264236179284866091 ) ) ;
#27180=CARTESIAN_POINT ( 'NONE',  ( -0.07405724077823318263, 0.1337342994872968427, -0.1787899950787401604 ) ) ;
#27181=CARTESIAN_POINT ( 'NONE',  ( 0.1787899950787401604, -1.789370078686394194, -0.07405724077823318263 ) ) ;
#27184=CARTESIAN_POINT ( 'NONE',  ( 0.1720202176924468251, -0.09842519685039369248, 0.03783562498418870101 ) ) ;
#27187=CARTESIAN_POINT ( 'NONE',  ( -0.06523048226347956391, -0.8075787401574794355, 0.1574803149606297803 ) ) ;
#27189=CARTESIAN_POINT ( 'NONE',  ( -0.07444174185955065859, -1.583213100921627703, -0.1797182628040039087 ) ) ;
#27202=CARTESIAN_POINT ( 'NONE',  ( -0.1574803149606300301, -0.8863188975302678241, -0.06523048226347956391 ) ) ;
#27203=CARTESIAN_POINT ( 'NONE',  ( -0.1264236179284866091, 0.02903543312462964626, -0.1264236179284866091 ) ) ;
#27214=CARTESIAN_POINT ( 'NONE',  ( 0.1787899950787401882, -1.363681102308440973, -2.189545951927503898E-17 ) ) ;
#27227=CARTESIAN_POINT ( 'NONE',  ( -0.06523048226347956391, -0.01033464556176428781, 0.1574803149606297803 ) ) ;
#27234=CARTESIAN_POINT ( 'NONE',  ( 0.1787899950787401604, -0.9440216060245140151, 0.07405724077823318263 ) ) ;
#27236=CARTESIAN_POINT ( 'NONE',  ( 0.1264236179284866091, 0.1028543307624250058, -0.1264236179284866091 ) ) ;
#27242=CARTESIAN_POINT ( 'NONE',  ( -0.1787899950787401604, -0.6722440944344262315, 0.07405724077823318263 ) ) ;
#27247=CARTESIAN_POINT ( 'NONE',  ( 0.1797182628040039087, -1.204276093047611740, 0.07444174185955046430 ) ) ;
#27248=CARTESIAN_POINT ( 'NONE',  ( 0.1746219128791692832, 0.1299212598425196763, 0.02006551292331004710 ) ) ;
#27258=CARTESIAN_POINT ( 'NONE',  ( 0.1574803149606300301, -0.7436023620971976555, -0.06523048226347956391 ) ) ;
#27268=CARTESIAN_POINT ( 'NONE',  ( 0.1113553986120547346, -1.735236220364913429, 0.1113553986120547346 ) ) ;
#27273=CARTESIAN_POINT ( 'NONE',  ( 0.1787899950787401882, 0.09793307091990532953, -2.189545951927503898E-17 ) ) ;
#27281=CARTESIAN_POINT ( 'NONE',  ( 0.06523048226347956391, -0.3597440943806616831, 0.1574803149606297803 ) ) ;
#27282=CARTESIAN_POINT ( 'NONE',  ( 0.1787899950787401882, -1.560531496009228247, -2.189545951927503898E-17 ) ) ;
#27290=CARTESIAN_POINT ( 'NONE',  ( 0.1787899950787401604, -0.5847696375205770902, -0.07405724077823318263 ) ) ;
#27291=CARTESIAN_POINT ( 'NONE',  ( -0.1179609706914375999, -0.08956081431181496522, -0.1345230454816687127 ) ) ;
#27299=CARTESIAN_POINT ( 'NONE',  ( 0.1787899950787401604, -1.484251968450174930, 0.07405724077823318263 ) ) ;
#27302=DIRECTION ( 'NONE',  ( 0.000000000000000000, 0.000000000000000000, 1.000000000000000000 ) ) ;
#27306=CARTESIAN_POINT ( 'NONE',  ( -1.100456976456230270E-17, -0.7589020772995805908, -0.1797182628040039365 ) ) ;
#27311=CARTESIAN_POINT ( 'NONE',  ( 0.1574803149606300301, -0.4778543307086612346, -0.06523048226347956391 ) ) ;
#27325=CARTESIAN_POINT ( 'NONE',  ( 0.1787899950787401604, -0.4950787401037172186, 0.07405724077823318263 ) ) ;
#27334=CARTESIAN_POINT ( 'NONE',  ( -0.07405724077823318263, -1.764763779473795813, 0.1787899950787401604 ) ) ;
#27335=CARTESIAN_POINT ( 'NONE',  ( -0.1264236179284866091, -0.9453740156942677109, 0.1264236179284866091 ) ) ;
#27336=CARTESIAN_POINT ( 'NONE',  ( -0.06523048226347956391, -1.437499999999999334, 0.1574803149606297803 ) ) ;
#27348=CARTESIAN_POINT ( 'NONE',  ( 0.000000000000000000, 0.09842519685039370636, 0.000000000000000000 ) ) ;
#27352=PLANE ( 'NONE',  #38284 ) ;
#27355=CARTESIAN_POINT ( 'NONE',  ( -0.1550283333641100658, 0.09383642490574128914, 0.1959274208663538963 ) ) ;
#27359=CARTESIAN_POINT ( 'NONE',  ( 0.2037090642851917544, -0.09842519685039370636, 0.05108520076791897568 ) ) ;
#27363=ORIENTED_EDGE ( 'NONE', *, *, #21368, .F. ) ;
#27364=CARTESIAN_POINT ( 'NONE',  ( 0.07405724077823318263, -1.001968503883243988, -0.1787899950787401604 ) ) ;
#27365=CARTESIAN_POINT ( 'NONE',  ( -0.07405724077823318263, -0.4704724408911186706, 0.1787899950787401604 ) ) ;
#27366=CARTESIAN_POINT ( 'NONE',  ( 0.07405724077823318263, -1.154527559001354842, -0.1787899950787401604 ) ) ;
#27368=CARTESIAN_POINT ( 'NONE',  ( 0.000000000000000000, 0.09842519685039370636, 0.2471922904502826812 ) ) ;
#27370=CARTESIAN_POINT ( 'NONE',  ( 0.1270800023317771588, -0.4882327859609983944, -0.1270800023317771588 ) ) ;
#27371=CARTESIAN_POINT ( 'NONE',  ( -0.1574803149606297803, -1.786909448711370585, 0.06523048226347956391 ) ) ;
#27373=CARTESIAN_POINT ( 'NONE',  ( -0.1574803149606300301, -0.06938976377952764396, -0.06523048226347956391 ) ) ;
#27374=CARTESIAN_POINT ( 'NONE',  ( 0.1787899950787401604, -0.1407480314422995815, -0.07405724077823318263 ) ) ;
#27382=CARTESIAN_POINT ( 'NONE',  ( 0.1787899950787401882, -0.4975393700249764461, -2.189545951927503898E-17 ) ) ;
#27384=CARTESIAN_POINT ( 'NONE',  ( 0.07405724077823318263, -1.430118110182456714, -0.1787899950787401604 ) ) ;
#27400=CARTESIAN_POINT ( 'NONE',  ( 4.681852760415787419E-17, -0.03219022224904102836, 0.2854330708661417804 ) ) ;
#27406=CARTESIAN_POINT ( 'NONE',  ( -0.2038129627511063025, -0.09851385024907242938, 0.1181531328361742073 ) ) ;
#27412=VERTEX_POINT ( 'NONE', #392 ) ;
#27414=CARTESIAN_POINT ( 'NONE',  ( -1.094772975963752103E-17, -0.5221456692375747721, -0.1787899950787401882 ) ) ;
#27420=CARTESIAN_POINT ( 'NONE',  ( -0.1787899950787401882, -0.2416338582139531399, 0.000000000000000000 ) ) ;
#27424=CARTESIAN_POINT ( 'NONE',  ( 3.284318927891251994E-17, -0.006521606024514312559, 0.1787899950787401882 ) ) ;
#27425=CARTESIAN_POINT ( 'NONE',  ( -0.1264236179284866091, 0.1471456693451021758, -0.1264236179284866091 ) ) ;
#27431=CARTESIAN_POINT ( 'NONE',  ( 0.06523048226347956391, -0.9060039370078742937, -0.1574803149606300301 ) ) ;
#27433=CARTESIAN_POINT ( 'NONE',  ( 0.07444174185955046430, -1.627504439504305456, -0.1797182628040039087 ) ) ;
#27443=CARTESIAN_POINT ( 'NONE',  ( 0.1787899950787401604, -0.02755905506434671789, 0.07405724077823318263 ) ) ;
#27455=CARTESIAN_POINT ( 'NONE',  ( -0.07405724077823318263, -1.390748031442299082, -0.1787899950787401604 ) ) ;
#27468=CARTESIAN_POINT ( 'NONE',  ( 0.1113553986120547346, -0.1899606298137326843, -0.1113553986120547346 ) ) ;
#27472=CARTESIAN_POINT ( 'NONE',  ( 0.1787899950787401604, -1.140871999725301844, 0.07405724077823318263 ) ) ;
#27474=CARTESIAN_POINT ( 'NONE',  ( -0.07405724077823318263, -0.1259842519147404416, -0.1787899950787401604 ) ) ;
#27483=CARTESIAN_POINT ( 'NONE',  ( -1.094772975963752103E-17, -0.6451771653005667906, -0.1787899950787401882 ) ) ;
#27489=CARTESIAN_POINT ( 'NONE',  ( 0.1797182628040039365, -1.123075305646037636, -2.200913952912460540E-17 ) ) ;
#27498=CARTESIAN_POINT ( 'NONE',  ( -0.1113553986120547346, -0.7312992124908976876, -0.1113553986120547346 ) ) ;
#27507=CARTESIAN_POINT ( 'NONE',  ( -0.1574803149606299191, -1.631889763672000004, 0.000000000000000000 ) ) ;
#27510=CARTESIAN_POINT ( 'NONE',  ( 0.06648378651154265850, -0.08350519546685050698, 0.2470477387547700132 ) ) ;
#27511=CARTESIAN_POINT ( 'NONE',  ( 0.1787899950787401604, 0.09547244099864542199, 0.07405724077823318263 ) ) ;
#27518=CARTESIAN_POINT ( 'NONE',  ( -0.07405724077823318263, -1.572834645615527327, 0.1787899950787401604 ) ) ;
#27528=CARTESIAN_POINT ( 'NONE',  ( 3.284318927891251994E-17, -0.6364428658670335803, 0.1787899950787401882 ) ) ;
#27530=CARTESIAN_POINT ( 'NONE',  ( -0.04408878395971095598, -0.08956088549465768267, -0.1785915423567586424 ) ) ;
#27532=EDGE_CURVE ( 'NONE', #30877, #5618, #1424, .T. ) ;
#27534=CARTESIAN_POINT ( 'NONE',  ( -0.07117121207836790697, -0.08956324299011318713, 0.1404802767937309016 ) ) ;
#27539=CARTESIAN_POINT ( 'NONE',  ( -0.1264236179284866091, -1.427657480261196987, -0.1264236179284866091 ) ) ;
#27543=CARTESIAN_POINT ( 'NONE',  ( -1.100456976456230270E-17, -0.7195319985594232914, -0.1797182628040039365 ) ) ;
#27546=CARTESIAN_POINT ( 'NONE',  ( -0.06523048226347956391, -0.4926181102362205966, 0.1574803149606297803 ) ) ;
#27557=CARTESIAN_POINT ( 'NONE',  ( -9.642888182262618425E-18, -0.5787401573727873894, -0.1574803149606299191 ) ) ;
#27562=CARTESIAN_POINT ( 'NONE',  ( -0.07405724077823318263, -0.5836614172690718361, 0.1787899950787401604 ) ) ;
#27569=CARTESIAN_POINT ( 'NONE',  ( -0.1787899950787401882, -1.654035433017102319, 0.000000000000000000 ) ) ;
#27570=CARTESIAN_POINT ( 'NONE',  ( 0.1264236179284866091, -1.043799212544661348, -0.1264236179284866091 ) ) ;
#27571=CARTESIAN_POINT ( 'NONE',  ( -0.1113553986120547346, -1.321850393700787496, 0.1113553986120547346 ) ) ;
#27588=CARTESIAN_POINT ( 'NONE',  ( -0.1944374611862008662, 0.07559918600398901622, -0.1731745503097413541 ) ) ;
#27593=CARTESIAN_POINT ( 'NONE',  ( -0.1787899950787401882, -0.2525845981504984405, 0.000000000000000000 ) ) ;
#27595=CARTESIAN_POINT ( 'NONE',  ( -0.01791361388587468795, -0.09842519685039370636, 0.2243562948544858549 ) ) ;
#27602=CARTESIAN_POINT ( 'NONE',  ( 0.1787899950787401882, -1.048720472387181024, -2.189545951927503898E-17 ) ) ;
#27603=CARTESIAN_POINT ( 'NONE',  ( -0.07405724077823318263, -1.188976377898991688, -0.1787899950787401604 ) ) ;
#27606=CARTESIAN_POINT ( 'NONE',  ( -1.100456976456230270E-17, -0.4439414473783212522, -0.1797182628040039365 ) ) ;
#27607=CARTESIAN_POINT ( 'NONE',  ( 0.06523048226347956391, 0.07824803149606307517, -0.1574803149606300301 ) ) ;
#27616=CARTESIAN_POINT ( 'NONE',  ( 0.07405724077823318263, -0.5049212597887556830, 0.1787899950787401604 ) ) ;
#27619=CARTESIAN_POINT ( 'NONE',  ( -0.07405724077823318263, -1.464566929080096225, -0.1787899950787401604 ) ) ;
#27632=CARTESIAN_POINT ( 'NONE',  ( 0.1327893737652135475, -0.09842568101169199557, -0.1197263300370822597 ) ) ;
#27643=CARTESIAN_POINT ( 'NONE',  ( 0.1605511194595065083, -0.09851384859890432999, 0.1447744158249297253 ) ) ;
#27645=EDGE_CURVE ( 'NONE', #44070, #3164, #2728, .T. ) ;
#27648=CARTESIAN_POINT ( 'NONE',  ( -1.094772975963752103E-17, -1.601009795000891911, -0.1787899950787401882 ) ) ;
#27649=ORIENTED_EDGE ( 'NONE', *, *, #5061, .F. ) ;
#27651=CARTESIAN_POINT ( 'NONE',  ( 0.07405724077823318263, -0.5787401574265509385, 0.1787899950787401604 ) ) ;
#27657=CARTESIAN_POINT ( 'NONE',  ( -0.1787899950787401604, -0.3622047243556850704, -0.07405724077823318263 ) ) ;
#27658=CARTESIAN_POINT ( 'NONE',  ( -0.1787899950787401604, -0.7509842519147402751, -0.07405724077823318263 ) ) ;
#27661=CARTESIAN_POINT ( 'NONE',  ( 0.1787899950787401604, 0.04515162232194235709, -0.07405724077823318263 ) ) ;
#27662=CARTESIAN_POINT ( 'NONE',  ( 0.07405724077823318263, 0.1250000000537635492, 0.1787899950787401604 ) ) ;
#27665=CARTESIAN_POINT ( 'NONE',  ( -0.1574803149606299191, -0.9724409448818898127, 0.000000000000000000 ) ) ;
#27667=CARTESIAN_POINT ( 'NONE',  ( 0.1797182628040039365, -1.634886329268084637, -2.200913952912460540E-17 ) ) ;
#27669=CARTESIAN_POINT ( 'NONE',  ( 0.1787899950787401604, -0.3720472440407247561, -0.07405724077823318263 ) ) ;
#27672=CARTESIAN_POINT ( 'NONE',  ( 0.1378230750848531139, 0.09774221684002680488, -0.2058608813653597380 ) ) ;
#27677=CARTESIAN_POINT ( 'NONE',  ( 0.1574803149606300301, -0.8617125983176697757, -0.06523048226347956391 ) ) ;
#27678=CARTESIAN_POINT ( 'NONE',  ( 0.1787899950787401604, 0.01181102367581077402, 0.07405724077823318263 ) ) ;
#27680=CARTESIAN_POINT ( 'NONE',  ( -0.1264236179284866091, -0.9010826771115905132, 0.1264236179284866091 ) ) ;
#27690=CARTESIAN_POINT ( 'NONE',  ( -1.094772975963752103E-17, -1.393208661363559031, -0.1787899950787401882 ) ) ;
#27693=DIRECTION ( 'NONE',  ( 0.000000000000000000, 0.000000000000000000, 1.000000000000000000 ) ) ;
#27706=CARTESIAN_POINT ( 'NONE',  ( -0.05938635157341645016, -0.07958416565545690935, -0.2511462791696849051 ) ) ;
#27711=CARTESIAN_POINT ( 'NONE',  ( 0.1264236179284866091, -1.064592472166246084, 0.1264236179284866091 ) ) ;
#27713=CARTESIAN_POINT ( 'NONE',  ( 0.07405724077823318263, -0.1702755904974175283, -0.1787899950787401604 ) ) ;
#27721=CARTESIAN_POINT ( 'NONE',  ( 0.1787899950787401604, -0.5787401574265509385, 0.07405724077823318263 ) ) ;
#27726=CARTESIAN_POINT ( 'NONE',  ( 0.07444174185955046430, -1.155063494622414977, -0.1797182628040039087 ) ) ;
#27735=CARTESIAN_POINT ( 'NONE',  ( 3.284318927891251994E-17, 0.1274606299750234428, 0.1787899950787401882 ) ) ;
#27746=CARTESIAN_POINT ( 'NONE',  ( 0.1574803149606299191, -1.651574803042078710, -1.928577636452523993E-17 ) ) ;
#27752=CARTESIAN_POINT ( 'NONE',  ( -9.642888182262618425E-18, -1.769685039370078705, -0.1574803149606299191 ) ) ;
#27758=CARTESIAN_POINT ( 'NONE',  ( -0.05613986198065470251, 0.07767250275969882212, 0.2530207064393422689 ) ) ;
#27760=ORIENTED_EDGE ( 'NONE', *, *, #35938, .T. ) ;
#27761=CARTESIAN_POINT ( 'NONE',  ( 0.1113553986120547346, -0.4261811022546779792, -0.1113553986120547346 ) ) ;
#27762=CARTESIAN_POINT ( 'NONE',  ( 0.1264236179284866091, -1.722933070812378009, 0.1264236179284866091 ) ) ;
#27770=CARTESIAN_POINT ( 'NONE',  ( -0.1264236179284866091, -0.6807342044497107780, 0.1264236179284866091 ) ) ;
#27773=CARTESIAN_POINT ( 'NONE',  ( 0.2037720324489346591, -0.08956011622649388826, 0.004864851714980023868 ) ) ;
#27785=CARTESIAN_POINT ( 'NONE',  ( 0.07444174185955046430, -0.7613627072208409841, -0.1797182628040039087 ) ) ;
#27786=CARTESIAN_POINT ( 'NONE',  ( 0.2471922904502827645, 0.09312491272442034729, 0.03902281811272177020 ) ) ;
#27788=CARTESIAN_POINT ( 'NONE',  ( -9.642888182262618425E-18, -0.4704724409448819422, -0.1574803149606299191 ) ) ;
#27801=CARTESIAN_POINT ( 'NONE',  ( -0.07405724077823318263, -0.5442913385289138706, 0.1787899950787401604 ) ) ;
#27811=CARTESIAN_POINT ( 'NONE',  ( 3.284318927891251994E-17, -1.644192913332062966, 0.1787899950787401882 ) ) ;
#27812=CARTESIAN_POINT ( 'NONE',  ( 0.1787899950787401604, -1.124999999946237228, -0.07405724077823318263 ) ) ;
#27813=CARTESIAN_POINT ( 'NONE',  ( 0.1574803149606300301, -1.383366141732283561, -0.06523048226347956391 ) ) ;
#27819=CARTESIAN_POINT ( 'NONE',  ( 2.892866454678787531E-17, -1.385826771546015745, 0.1574803149606299191 ) ) ;
#27826=CARTESIAN_POINT ( 'NONE',  ( 0.05612302249891599343, -0.07766248740294799668, -0.2530304272095452167 ) ) ;
#27829=CARTESIAN_POINT ( 'NONE',  ( 0.07405724077823318263, -0.2648877477567979088, -0.1787899950787401604 ) ) ;
#27831=CARTESIAN_POINT ( 'NONE',  ( -0.05991043469119292086, -0.09842519685039370636, -0.1769877046850827085 ) ) ;
#27832=CARTESIAN_POINT ( 'NONE',  ( -0.1574803149606297803, 0.01427165354330708555, 0.06523048226347956391 ) ) ;
#27838=CARTESIAN_POINT ( 'NONE',  ( 3.284318927891251994E-17, -1.289862204670645607, 0.1787899950787401882 ) ) ;
#27841=CARTESIAN_POINT ( 'NONE',  ( -0.1797182628040039087, -0.5103784552523373819, 0.07444174185955065859 ) ) ;
#27844=CARTESIAN_POINT ( 'NONE',  ( 0.06523048226347956391, 0.06348425196850393526, 0.1574803149606297803 ) ) ;
#27853=CARTESIAN_POINT ( 'NONE',  ( 0.1264236179284866091, -0.6500984251430865779, -0.1264236179284866091 ) ) ;
#27854=CARTESIAN_POINT ( 'NONE',  ( -0.1264236179284866091, -1.334153543253322916, 0.1264236179284866091 ) ) ;
#27857=ORIENTED_EDGE ( 'NONE', *, *, #43772, .T. ) ;
#27858=ORIENTED_EDGE ( 'NONE', *, *, #6862, .T. ) ;
#27866=CARTESIAN_POINT ( 'NONE',  ( 0.1796295154111492431, -0.08412760742822553151, 0.1817225848801442278 ) ) ;
#27867=CARTESIAN_POINT ( 'NONE',  ( 0.1113553986120547346, -0.09153543307086613179, 0.1113553986120547346 ) ) ;
#27871=CARTESIAN_POINT ( 'NONE',  ( 0.2074532133938310763, -0.09851384671466711929, 0.02027945527772259671 ) ) ;
#27876=CARTESIAN_POINT ( 'NONE',  ( -0.1264236179284866091, -1.596088535158372235, -0.1264236179284866091 ) ) ;
#27879=CARTESIAN_POINT ( 'NONE',  ( 0.1264236179284866091, -0.6550196849856062542, 0.1264236179284866091 ) ) ;
#27883=CARTESIAN_POINT ( 'NONE',  ( 0.1787899950787401604, -0.3031496062454492879, 0.07405724077823318263 ) ) ;
#27884=CARTESIAN_POINT ( 'NONE',  ( -0.07405724077823318263, -0.7559055117572593963, -0.1787899950787401604 ) ) ;
#27890=CARTESIAN_POINT ( 'NONE',  ( -0.1787899950787401604, 0.06483666169202111085, 0.07405724077823318263 ) ) ;
#27891=CARTESIAN_POINT ( 'NONE',  ( 0.07405724077823318263, 0.04625984257344856188, 0.1787899950787401604 ) ) ;
#27896=CARTESIAN_POINT ( 'NONE',  ( -0.06523048226347956391, -0.8223425196850393526, -0.1574803149606300301 ) ) ;
#27898=CARTESIAN_POINT ( 'NONE',  ( -0.1270800023317771588, -1.620122549740525386, -0.1270800023317771588 ) ) ;
#27899=CARTESIAN_POINT ( 'NONE',  ( -0.1574803149606300301, -0.5319881888688510196, -0.06523048226347956391 ) ) ;
#27900=CARTESIAN_POINT ( 'NONE',  ( -0.1264236179284866091, -0.3892716534895436786, 0.1264236179284866091 ) ) ;
#27909=CARTESIAN_POINT ( 'NONE',  ( 0.1264236179284866091, -0.06938976372576398377, 0.1264236179284866091 ) ) ;
#27911=CARTESIAN_POINT ( 'NONE',  ( 0.07405724077823318263, -0.8789370078202529690, -0.1787899950787401604 ) ) ;
#27919=CARTESIAN_POINT ( 'NONE',  ( -0.1113553986120547346, -1.085629921152315047, -0.1113553986120547346 ) ) ;
#27927=CARTESIAN_POINT ( 'NONE',  ( 0.07405724077823318263, 0.08562992131360593062, 0.1787899950787401604 ) ) ;
#27934=CARTESIAN_POINT ( 'NONE',  ( -0.1787899950787401882, -1.158096409174120156, 0.000000000000000000 ) ) ;
#27935=ORIENTED_EDGE ( 'NONE', *, *, #28594, .F. ) ;
#27936=CARTESIAN_POINT ( 'NONE',  ( -0.1264236179284866091, -0.07431102356828367395, 0.1264236179284866091 ) ) ;
#27949=CARTESIAN_POINT ( 'NONE',  ( -0.1797182628040039087, -1.219039872575171213, 0.07444174185955065859 ) ) ;
#27967=CARTESIAN_POINT ( 'NONE',  ( 0.1728472449644665732, -0.09617745053770661301, -0.07999999089250650619 ) ) ;
#27970=CARTESIAN_POINT ( 'NONE',  ( 0.09431337879938411772, -0.09445537554013619386, 0.2309807168374905517 ) ) ;
#27972=CARTESIAN_POINT ( 'NONE',  ( -0.07405724077823318263, 0.07086614178604697112, -0.1787899950787401604 ) ) ;
#27973=CARTESIAN_POINT ( 'NONE',  ( 0.2372856289813619346, 0.04209688371796207335, 0.1484361490989228038 ) ) ;
#27978=CARTESIAN_POINT ( 'NONE',  ( -0.1787899950787401604, -1.622047244040725866, -0.07405724077823318263 ) ) ;
#27987=CARTESIAN_POINT ( 'NONE',  ( -0.1264236179284866091, -0.6905767241347500196, -0.1264236179284866091 ) ) ;
#27989=CARTESIAN_POINT ( 'NONE',  ( 0.1783903336175657606, -0.08956053790448267882, -0.08775565328239233465 ) ) ;
#27995=CARTESIAN_POINT ( 'NONE',  ( 0.1574803149606300301, 0.07332677165354323234, -0.06523048226347956391 ) ) ;
#28002=EDGE_LOOP ( 'NONE', ( #31665, #25805, #9881 ) ) ;
#28003=CARTESIAN_POINT ( 'NONE',  ( -0.1797182628040039087, -0.6678587702129673564, 0.07444174185955065859 ) ) ;
#28006=CARTESIAN_POINT ( 'NONE',  ( -9.642888182262618425E-18, -0.5098425196850393526, -0.1574803149606299191 ) ) ;
#28007=CARTESIAN_POINT ( 'NONE',  ( -0.1713481153329562412, -0.09842519685039370636, -0.04016550290184540267 ) ) ;
#28013=EDGE_CURVE ( 'NONE', #4638, #6112, #6814, .T. ) ;
#28020=CARTESIAN_POINT ( 'NONE',  ( -0.1625082278952665604, -0.08956041897765029680, -0.06009421481027538842 ) ) ;
#28021=CARTESIAN_POINT ( 'NONE',  ( 0.1787899950787401882, -0.5713582676627716461, -2.189545951927503898E-17 ) ) ;
#28024=CARTESIAN_POINT ( 'NONE',  ( 0.1562117447733968045, 0.1299212598425196763, 0.09007225877465360742 ) ) ;
#28028=CARTESIAN_POINT ( 'NONE',  ( -0.03894127257522794067, 0.06746187776206562237, -0.2629503166622473853 ) ) ;
#28030=CARTESIAN_POINT ( 'NONE',  ( 3.301370929368692659E-17, 0.04818453687364732119, 0.1797182628040039365 ) ) ;
#28031=CARTESIAN_POINT ( 'NONE',  ( -0.1787899950787401604, -0.9921259841982054128, -0.07405724077823318263 ) ) ;
#28032=CARTESIAN_POINT ( 'NONE',  ( 0.1574803149606300301, -1.309547244094489082, 0.06523048226347956391 ) ) ;
#28039=CARTESIAN_POINT ( 'NONE',  ( 0.1113553986120547346, -1.420275590443653480, 0.1113553986120547346 ) ) ;
#28051=CARTESIAN_POINT ( 'NONE',  ( -0.07405724077823318263, -0.2993365666544354209, -0.1787899950787401604 ) ) ;
#28052=CARTESIAN_POINT ( 'NONE',  ( 0.08748153575225099676, -0.09842519685039370636, 0.2018362251056389500 ) ) ;
#28055=AXIS2_PLACEMENT_3D ( 'NONE', #44116, #36249, #36481 ) ;
#28060=CARTESIAN_POINT ( 'NONE',  ( -0.1787899950787401604, -1.065944881836000224, 0.07405724077823318263 ) ) ;
#28061=CARTESIAN_POINT ( 'NONE',  ( 0.1787899950787401604, -1.159448818843874074, -0.07405724077823318263 ) ) ;
#28063=CARTESIAN_POINT ( 'NONE',  ( 0.07444174185955046430, -0.4464020772995807018, -0.1797182628040039087 ) ) ;
#28066=CARTESIAN_POINT ( 'NONE',  ( 0.1574803149606299191, -0.007874015748031495954, -1.928577636452523993E-17 ) ) ;
#28075=CARTESIAN_POINT ( 'NONE',  ( 0.1264236179284866091, -0.6599409448281259305, 0.1264236179284866091 ) ) ;
#28076=CARTESIAN_POINT ( 'NONE',  ( 0.07405724077823318263, -1.326771653489542402, 0.1787899950787401604 ) ) ;
#28083=DIRECTION ( 'NONE',  ( 0.000000000000000000, -1.000000000000000000, 0.000000000000000000 ) ) ;
#28086=CARTESIAN_POINT ( 'NONE',  ( 0.1227919659947372816, -0.09843992453377478635, -0.1299906436365789453 ) ) ;
#28096=CARTESIAN_POINT ( 'NONE',  ( -0.2009589076016815024, -0.09851385032380531592, 0.1224783046148972404 ) ) ;
#28101=CARTESIAN_POINT ( 'NONE',  ( -0.07405724077823318263, -1.598549165079632406, -0.1787899950787401604 ) ) ;
#28103=CARTESIAN_POINT ( 'NONE',  ( 0.07405724077823318263, -0.5246062991588343882, -0.1787899950787401604 ) ) ;
#28109=CARTESIAN_POINT ( 'NONE',  ( 0.07405724077823318263, -0.3080708660879689087, 0.1787899950787401604 ) ) ;
#28110=CARTESIAN_POINT ( 'NONE',  ( 0.1264236179284866091, -0.7632874015210393548, -0.1264236179284866091 ) ) ;
#28112=CARTESIAN_POINT ( 'NONE',  ( 0.1787899950787401604, 0.04023036247942270160, 0.07405724077823318263 ) ) ;
#28113=CARTESIAN_POINT ( 'NONE',  ( 0.07405724077823318263, 0.06102362210100767403, -0.1787899950787401604 ) ) ;
#28120=CARTESIAN_POINT ( 'NONE',  ( -0.06523048226347956391, -0.9256889763779536651, 0.1574803149606297803 ) ) ;
#28122=CARTESIAN_POINT ( 'NONE',  ( 0.1797182628040039087, -1.755457195409817928, 0.07444174185955046430 ) ) ;
#28125=CARTESIAN_POINT ( 'NONE',  ( 0.1711856790334206346, 0.08819060268784824352, -0.1865989729947874209 ) ) ;
#28130=DIRECTION ( 'NONE',  ( 0.000000000000000000, -1.000000000000000000, 0.000000000000000000 ) ) ;
#28132=CARTESIAN_POINT ( 'NONE',  ( 0.1574803149606300301, -0.9060039369003467513, 0.06523048226347956391 ) ) ;
#28133=CARTESIAN_POINT ( 'NONE',  ( 0.1787899950787401882, -0.1432086613635592531, -2.189545951927503898E-17 ) ) ;
#28135=CARTESIAN_POINT ( 'NONE',  ( -1.094772975963752103E-17, -0.9552165353793071745, -0.1787899950787401882 ) ) ;
#28136=DIRECTION ( 'NONE',  ( 0.000000000000000000, 1.000000000000000000, 0.000000000000000000 ) ) ;
#28160=CARTESIAN_POINT ( 'NONE',  ( -0.1264236179284866091, -1.084277511536324790, -0.1264236179284866091 ) ) ;
#28162=CARTESIAN_POINT ( 'NONE',  ( -0.1264236179284866091, -0.1628937007336379861, -0.1264236179284866091 ) ) ;
#28169=CARTESIAN_POINT ( 'NONE',  ( 0.1797182628040039087, -0.2593942032838327805, 0.07444174185955046430 ) ) ;
#28170=CARTESIAN_POINT ( 'NONE',  ( 0.1787899950787401882, -0.8124999999462361178, -2.189545951927503898E-17 ) ) ;
#28172=CARTESIAN_POINT ( 'NONE',  ( -0.07444174185955065859, -1.332228848953123990, 0.1797182628040039087 ) ) ;
#28184=CARTESIAN_POINT ( 'NONE',  ( 0.1787899950787401882, -0.02017716530056720692, -2.189545951927503898E-17 ) ) ;
#28192=CARTESIAN_POINT ( 'NONE',  ( 0.1574803149606300301, -1.019192913278299528, -0.06523048226347956391 ) ) ;
#28197=CARTESIAN_POINT ( 'NONE',  ( -0.1787899950787401604, -0.03740157474938609478, 0.07405724077823318263 ) ) ;
#28204=CARTESIAN_POINT ( 'NONE',  ( 0.07405724077823318263, -1.764763779473795813, 0.1787899950787401604 ) ) ;
#28210=CIRCLE ( 'NONE', #9832, 0.2471922904502826812 ) ;
#28214=CARTESIAN_POINT ( 'NONE',  ( -0.03548959504743665755, -0.08956203235299665943, 0.1510601953534446984 ) ) ;
#28215=CARTESIAN_POINT ( 'NONE',  ( -0.06008722723381313552, -0.08905839832210296625, 0.1460962461687339564 ) ) ;
#28218=ADVANCED_FACE ( 'NONE', ( #47075 ), #7764, .F. ) ;
#28227=CARTESIAN_POINT ( 'NONE',  ( 0.1797182628040039365, -0.7293745182444626440, -2.200913952912460540E-17 ) ) ;
#28228=CARTESIAN_POINT ( 'NONE',  ( 0.2471922904502826812, 0.03219022224904106305, 0.1427165354330708902 ) ) ;
#28231=CARTESIAN_POINT ( 'NONE',  ( -0.1574803149606300301, -0.6205708661417322913, -0.06523048226347956391 ) ) ;
#28232=CARTESIAN_POINT ( 'NONE',  ( 0.2471922904502825702, 0.05534442469270777626, -0.1143959998688843099 ) ) ;
#28235=B_SPLINE_CURVE_WITH_KNOTS ( 'NONE', 3,
 ( #13594, #21011, #28232, #23093, #44631, #31014, #45580, #16155, #44872, #23570, #45354, #11846, #40162, #30549, #4618, #4864, #5101, #7995, #30100, #22620 ),
 .UNSPECIFIED., .F., .F.,
 ( 4, 1, 1, 1, 1, 1, 2, 2, 1, 1, 1, 2, 2, 4 ),
 ( 0.000000000000000000, 0.2499999999999993339, 0.3749999999999988898, 0.4374999999999986677, 0.4687499999999986122, 0.4843749999999986677, 0.4921874999999986122, 0.4999999999999986122, 0.6249999999999983347, 0.6874999999999982236, 0.7187499999999982236, 0.7343749999999982236, 0.7499999999999983347, 1.000000000000000000 ),
 .UNSPECIFIED. ) ;
#28252=CARTESIAN_POINT ( 'NONE',  ( -0.07444174185955065859, 0.1490703636453008241, -0.1797182628040039087 ) ) ;
#28253=CARTESIAN_POINT ( 'NONE',  ( 0.07405724077823318263, -1.095472440891117838, 0.1787899950787401604 ) ) ;
#28254=CARTESIAN_POINT ( 'NONE',  ( -9.642888182262618425E-18, -1.572834645669291431, -0.1574803149606299191 ) ) ;
#28274=CARTESIAN_POINT ( 'NONE',  ( -1.094772975963752103E-17, -0.2624271178355381817, -0.1787899950787401882 ) ) ;
#28275=CARTESIAN_POINT ( 'NONE',  ( -0.1299468115398441093, -0.09842519685039370636, 0.1029827665312899737 ) ) ;
#28284=CARTESIAN_POINT ( 'NONE',  ( 0.1787899950787401882, -1.206200787347811110, -2.189545951927503898E-17 ) ) ;
#28285=CARTESIAN_POINT ( 'NONE',  ( -0.1264236179284866091, -1.294783464513165283, 0.1264236179284866091 ) ) ;
#28287=CARTESIAN_POINT ( 'NONE',  ( -0.1270800023317771588, -0.4291776678507621678, 0.1270800023317771588 ) ) ;
#28292=CARTESIAN_POINT ( 'NONE',  ( -0.1113553986120547346, -0.1407480314960629919, 0.1113553986120547346 ) ) ;
#28301=CARTESIAN_POINT ( 'NONE',  ( 0.07405724077823318263, -0.5442913385289138706, 0.1787899950787401604 ) ) ;
#28302=CARTESIAN_POINT ( 'NONE',  ( 0.1787899950787401604, -1.395669291284819868, -0.07405724077823318263 ) ) ;
#28310=CARTESIAN_POINT ( 'NONE',  ( -9.642888182262618425E-18, -1.287401574695621997, -0.1574803149606299191 ) ) ;
#28312=CARTESIAN_POINT ( 'NONE',  ( 0.1348365057045624593, -0.09842519898778306908, -0.1174095120931970271 ) ) ;
#28320=CARTESIAN_POINT ( 'NONE',  ( -0.1574803149606299191, -0.2539370077664885872, 0.000000000000000000 ) ) ;
#28324=CARTESIAN_POINT ( 'NONE',  ( 0.2064083604912952674, -0.09851384708312717342, -0.01080128761237854514 ) ) ;
#28327=CARTESIAN_POINT ( 'NONE',  ( -0.1787899950787401604, -1.746186960355224027, 0.07405724077823318263 ) ) ;
#28329=CARTESIAN_POINT ( 'NONE',  ( -0.1264236179284866091, -0.6648622046706456068, 0.1264236179284866091 ) ) ;
#28335=CARTESIAN_POINT ( 'NONE',  ( 0.1787899950787401604, -0.2637795275052916555, 0.07405724077823318263 ) ) ;
#28336=CARTESIAN_POINT ( 'NONE',  ( 3.284318927891251994E-17, -0.6993110235682834519, 0.1787899950787401882 ) ) ;
#28342=CARTESIAN_POINT ( 'NONE',  ( -0.1264236179284866091, 0.05745477192824158252, -0.1264236179284866091 ) ) ;
#28343=CARTESIAN_POINT ( 'NONE',  ( 0.1787899950787401604, 0.01181102367581077402, 0.07405724077823318263 ) ) ;
#28348=DIMENSIONAL_EXPONENTS ( 1.000000000000000000, 0.000000000000000000, 0.000000000000000000, 0.000000000000000000, 0.000000000000000000, 0.000000000000000000, 0.000000000000000000 ) ;
#28350=CARTESIAN_POINT ( 'NONE',  ( 0.1113553986120547346, -0.8395669291338583307, 0.1113553986120547346 ) ) ;
#28351=CARTESIAN_POINT ( 'NONE',  ( -0.1270800023317771588, -1.728390266275958709, 0.1270800023317771588 ) ) ;
#28353=CARTESIAN_POINT ( 'NONE',  ( -0.1113553986120547346, -0.4852362203649134287, 0.1113553986120547346 ) ) ;
#28354=CARTESIAN_POINT ( 'NONE',  ( 0.1787899950787401882, -0.3351377952218271283, -2.189545951927503898E-17 ) ) ;
#28363=CARTESIAN_POINT ( 'NONE',  ( 0.1574803149606300301, -0.9010826770578276301, -0.06523048226347956391 ) ) ;
#28364=CARTESIAN_POINT ( 'NONE',  ( -0.1787899950787401604, -0.04232283459190575720, 0.07405724077823318263 ) ) ;
#28366=CARTESIAN_POINT ( 'NONE',  ( 0.1787899950787401604, -0.8838582676627719792, -0.07405724077823318263 ) ) ;
#28377=CARTESIAN_POINT ( 'NONE',  ( -0.1574803149606299191, -1.120078740049952781, 0.000000000000000000 ) ) ;
#28389=CARTESIAN_POINT ( 'NONE',  ( -0.07405724077823318263, 0.1053149606836847191, -0.1787899950787401604 ) ) ;
#28395=CARTESIAN_POINT ( 'NONE',  ( -0.2471922904502826812, 0.09336655125506151953, -0.03811874944176997515 ) ) ;
#28397=CARTESIAN_POINT ( 'NONE',  ( -0.07405724077823318263, -1.362328692638688388, -0.1787899950787401604 ) ) ;
#28399=CARTESIAN_POINT ( 'NONE',  ( -0.1787899950787401882, -0.1186023621509610243, 0.000000000000000000 ) ) ;
#28406=CARTESIAN_POINT ( 'NONE',  ( -1.094772975963752103E-17, -1.471948818843874074, -0.1787899950787401882 ) ) ;
#28407=CARTESIAN_POINT ( 'NONE',  ( -0.1787899950787401604, -0.7116141731745821986, 0.07405724077823318263 ) ) ;
#28421=CARTESIAN_POINT ( 'NONE',  ( -0.1574803149606299191, -0.7657480313885355327, 0.000000000000000000 ) ) ;
#28423=CARTESIAN_POINT ( 'NONE',  ( 3.284318927891251994E-17, 0.009350393754550925460, 0.1787899950787401882 ) ) ;
#28434=CARTESIAN_POINT ( 'NONE',  ( -0.06523048226347956391, -1.033956692805859445, 0.1574803149606297803 ) ) ;
#28436=ORIENTED_EDGE ( 'NONE', *, *, #19900, .T. ) ;
#28442=CARTESIAN_POINT ( 'NONE',  ( -1.094772975963752103E-17, -0.04970472435568527164, -0.1787899950787401882 ) ) ;
#28449=CARTESIAN_POINT ( 'NONE',  ( 0.1787899950787401882, -1.639271653489543290, -2.189545951927503898E-17 ) ) ;
#28456=CARTESIAN_POINT ( 'NONE',  ( -0.07405724077823318263, -0.7324074327961683784, -0.1787899950787401604 ) ) ;
#28467=CARTESIAN_POINT ( 'NONE',  ( 0.1574803149606299191, -0.007874015748031495954, -1.928577636452523993E-17 ) ) ;
#28473=CARTESIAN_POINT ( 'NONE',  ( -0.07444174185955065859, -0.8745516835987940940, -0.1797182628040039087 ) ) ;
#28477=CARTESIAN_POINT ( 'NONE',  ( 0.1574803149606300301, -0.5565944881889764995, -0.06523048226347956391 ) ) ;
#28484=CARTESIAN_POINT ( 'NONE',  ( 2.892866454678787531E-17, -0.6377952754830236159, 0.1574803149606299191 ) ) ;
#28501=CARTESIAN_POINT ( 'NONE',  ( -0.1797182628040039365, 0.1170821746689230392, 0.000000000000000000 ) ) ;
#28502=CARTESIAN_POINT ( 'NONE',  ( 0.1787899950787401882, -1.009350393647023614, -2.189545951927503898E-17 ) ) ;
#28503=CARTESIAN_POINT ( 'NONE',  ( 0.1113553986120547346, -1.587598425196850460, 0.1113553986120547346 ) ) ;
#28517=CARTESIAN_POINT ( 'NONE',  ( 0.1787899950787401604, -0.1959901099615224129, 0.07405724077823318263 ) ) ;
#28518=CARTESIAN_POINT ( 'NONE',  ( -0.1699099310998980483, -0.09842519685039370636, 0.02539414388011468349 ) ) ;
#28528=CARTESIAN_POINT ( 'NONE',  ( 0.1787899950787401882, -1.127460629867496067, -2.189545951927503898E-17 ) ) ;
#28529=CARTESIAN_POINT ( 'NONE',  ( 0.1787899950787401604, -1.356299212544662014, -0.07405724077823318263 ) ) ;
#28531=CARTESIAN_POINT ( 'NONE',  ( 0.07444174185955046430, -0.6038823922602111205, -0.1797182628040039087 ) ) ;
#28536=CARTESIAN_POINT ( 'NONE',  ( 0.1574803149606299191, -0.1259842519685039353, -1.928577636452523993E-17 ) ) ;
#28548=EDGE_LOOP ( 'NONE', ( #4792, #43689, #37925, #4423, #3886 ) ) ;
#28551=CARTESIAN_POINT ( 'NONE',  ( -0.06523048226347956391, -1.506397637687749702, 0.1574803149606297803 ) ) ;
#28552=CARTESIAN_POINT ( 'NONE',  ( 3.284318927891251994E-17, -0.5467519684501732646, 0.1787899950787401882 ) ) ;
#28555=VECTOR ( 'NONE', #24306, 39.37007874015748143 ) ;
#28568=CARTESIAN_POINT ( 'NONE',  ( 0.1675084398155860799, -0.08956740676346343355, 0.1887210895736453897 ) ) ;
#28570=CARTESIAN_POINT ( 'NONE',  ( 2.892866454678787531E-17, -0.1653543306011344416, 0.1574803149606299191 ) ) ;
#28577=CARTESIAN_POINT ( 'NONE',  ( -0.1674288283605931127, -0.09851383564138858906, -0.05723794432179189068 ) ) ;
#28581=CARTESIAN_POINT ( 'NONE',  ( -0.1787899950787401604, -1.711738141457585627, -0.07405724077823318263 ) ) ;
#28587=CARTESIAN_POINT ( 'NONE',  ( 0.1264236179284866091, -0.2662401574265516047, 0.1264236179284866091 ) ) ;
#28588=CARTESIAN_POINT ( 'NONE',  ( 0.1787899950787401604, -0.9232283464029299447, -0.07405724077823318263 ) ) ;
#28590=CARTESIAN_POINT ( 'NONE',  ( -0.2471902767489406183, -0.09658829859166317977, -0.02317992046427616928 ) ) ;
#28594=EDGE_CURVE ( 'NONE', #46609, #43211, #37477, .T. ) ;
#28597=CARTESIAN_POINT ( 'NONE',  ( 3.284318927891251994E-17, -0.1640019209851442950, 0.1787899950787401882 ) ) ;
#28598=CARTESIAN_POINT ( 'NONE',  ( 0.1787899950787401604, 0.09055118115612580121, 0.07405724077823318263 ) ) ;
#28606=CARTESIAN_POINT ( 'NONE',  ( -0.1797182628040039087, -1.775142234779896411, -0.07444174185955065859 ) ) ;
#28614=CARTESIAN_POINT ( 'NONE',  ( -0.1594432092296970138, -0.09246610911301904323, -0.1933784749626324961 ) ) ;
#28617=CARTESIAN_POINT ( 'NONE',  ( -0.1787899950787401604, -0.1653543306548978520, -0.07405724077823318263 ) ) ;
#28619=CARTESIAN_POINT ( 'NONE',  ( 0.1787899950787401604, -1.120078740103715997, -0.07405724077823318263 ) ) ;
#28640=CARTESIAN_POINT ( 'NONE',  ( 0.1264236179284866091, 0.01919291343959031448, -0.1264236179284866091 ) ) ;
#28647=CARTESIAN_POINT ( 'NONE',  ( -0.1264236179284866091, -1.320497983977269918, -0.1264236179284866091 ) ) ;
#28649=CARTESIAN_POINT ( 'NONE',  ( 0.1264236179284866091, -0.2613188975840319284, 0.1264236179284866091 ) ) ;
#28654=CARTESIAN_POINT ( 'NONE',  ( -0.2471922931865199735, -0.07794380098772846210, 0.07736948232528978453 ) ) ;
#28657=CARTESIAN_POINT ( 'NONE',  ( -0.1787899950787401604, -1.420275590497418250, 0.07405724077823318263 ) ) ;
#28658=CARTESIAN_POINT ( 'NONE',  ( -0.1787899950787401604, -0.7903543306548983516, 0.07405724077823318263 ) ) ;
#28665=CARTESIAN_POINT ( 'NONE',  ( -0.01411529459472660869, 0.1299212598425194265, 0.1732737445343259797 ) ) ;
#28677=ORIENTED_EDGE ( 'NONE', *, *, #39158, .T. ) ;
#28680=CARTESIAN_POINT ( 'NONE',  ( 0.1574803149606300301, -1.024114173120818982, 0.06523048226347956391 ) ) ;
#28686=CARTESIAN_POINT ( 'NONE',  ( -0.07405724077823318263, -0.007874015694267993623, -0.1787899950787401604 ) ) ;
#28691=CARTESIAN_POINT ( 'NONE',  ( 0.1235961452251413406, -0.09842519685039370636, -0.2140748031496062798 ) ) ;
#28695=CARTESIAN_POINT ( 'NONE',  ( 0.1574803149606299191, 0.1200787402650072971, -1.928577636452523993E-17 ) ) ;
#28702=CARTESIAN_POINT ( 'NONE',  ( -0.1264236179284866091, -0.7693168816150650624, -0.1264236179284866091 ) ) ;
#28704=CARTESIAN_POINT ( 'NONE',  ( -0.02028039986305122527, -0.08956190947767678212, 0.1525088234432795398 ) ) ;
#28722=CARTESIAN_POINT ( 'NONE',  ( -0.1797182628040039365, -0.9065398725751713238, 0.000000000000000000 ) ) ;
#28726=CARTESIAN_POINT ( 'NONE',  ( 0.1113553986120547346, -0.5147637795275590289, -0.1113553986120547346 ) ) ;
#28727=CARTESIAN_POINT ( 'NONE',  ( -0.05777579460957081581, 0.1215522599344571048, -0.1483226373755269778 ) ) ;
#28736=CARTESIAN_POINT ( 'NONE',  ( -0.07405724077823318263, -0.6624015747493856576, 0.1787899950787401604 ) ) ;
#28746=CARTESIAN_POINT ( 'NONE',  ( -0.1797182628040039365, 0.07771209592876555938, 0.000000000000000000 ) ) ;
#28747=CARTESIAN_POINT ( 'NONE',  ( -0.1787899950787401604, -1.149606299158835387, -0.07405724077823318263 ) ) ;
#28748=CARTESIAN_POINT ( 'NONE',  ( 0.1574803149606299191, -1.503937007874015741, -1.928577636452523993E-17 ) ) ;
#28758=CARTESIAN_POINT ( 'NONE',  ( -0.1910524284696294706, 0.07767250275969714290, -0.1751288998598694580 ) ) ;
#28762=CARTESIAN_POINT ( 'NONE',  ( 0.1787899950787401604, -0.4272893225599475042, -0.07405724077823318263 ) ) ;
#28763=CARTESIAN_POINT ( 'NONE',  ( -0.1585347235887767658, -0.09842519685039370636, -0.08158260120612992328 ) ) ;
#28772=CIRCLE ( 'NONE', #8067, 0.2471922904502826812 ) ;
#28774=CARTESIAN_POINT ( 'NONE',  ( 0.07405724077823318263, -1.198818897584032150, -0.1787899950787401604 ) ) ;
#28775=CARTESIAN_POINT ( 'NONE',  ( 0.1787899950787401604, -1.400590551127339323, 0.07405724077823318263 ) ) ;
#28777=SHAPE_REPRESENTATION_RELATIONSHIP ( 'NONE' , 'NONE' ,  #45408, #24384 ) ;
#28788=CARTESIAN_POINT ( 'NONE',  ( -0.1574803149606297803, -0.06446850393700777337, 0.06523048226347956391 ) ) ;
#28790=LINE ( 'NONE', #17259, #42222 ) ;
#28796=CARTESIAN_POINT ( 'NONE',  ( 0.1113553986120547346, -1.489173228238929170, -0.1113553986120547346 ) ) ;
#28797=CARTESIAN_POINT ( 'NONE',  ( -0.1787899950787401604, -0.6377952755367874982, -0.07405724077823318263 ) ) ;
#28798=CARTESIAN_POINT ( 'NONE',  ( -0.1113553986120547346, -1.125000000000000000, 0.1113553986120547346 ) ) ;
#28809=CARTESIAN_POINT ( 'NONE',  ( -0.1574803149606300301, -1.280019684931841706, -0.06523048226347956391 ) ) ;
#28817=CARTESIAN_POINT ( 'NONE',  ( 0.06523048226347956391, -0.2810039369003468623, 0.1574803149606297803 ) ) ;
#28822=CARTESIAN_POINT ( 'NONE',  ( 0.0007072645643074310616, -0.09851384404544488715, -0.1904345280194874035 ) ) ;
#28827=CARTESIAN_POINT ( 'NONE',  ( -0.07405724077823318263, -1.716659401300104193, -0.1787899950787401604 ) ) ;
#28829=CARTESIAN_POINT ( 'NONE',  ( -0.1787899950787401882, -0.6697834645131652831, 0.000000000000000000 ) ) ;
#28835=CARTESIAN_POINT ( 'NONE',  ( -0.1787899950787401604, -0.9478346456155283262, -0.07405724077823318263 ) ) ;
#28839=CARTESIAN_POINT ( 'NONE',  ( -0.07405724077823318263, -0.1024861729536482163, -0.1787899950787401604 ) ) ;
#28840=CARTESIAN_POINT ( 'NONE',  ( -0.1787899950787401604, -0.002952755851748290004, 0.07405724077823318263 ) ) ;
#28841=CARTESIAN_POINT ( 'NONE',  ( 0.2471922466705862576, -0.08138981793850655344, -0.07067796049199921715 ) ) ;
#28845=CARTESIAN_POINT ( 'NONE',  ( 0.1797182628040039087, -1.711165856827140619, -0.07444174185955065859 ) ) ;
#28846=CARTESIAN_POINT ( 'NONE',  ( 0.000000000000000000, -0.09842519685039370636, 0.000000000000000000 ) ) ;
#28848=CARTESIAN_POINT ( 'NONE',  ( -0.1293255151917100387, -0.09842519685039366473, 0.2107669498571209110 ) ) ;
#28854=CARTESIAN_POINT ( 'NONE',  ( -0.1574803149606299191, -0.9232283463491653963, 0.000000000000000000 ) ) ;
#28855=CARTESIAN_POINT ( 'NONE',  ( 0.07405724077823318263, -0.09645669285962235606, -0.1787899950787401604 ) ) ;
#28859=CARTESIAN_POINT ( 'NONE',  ( -0.1787899950787401604, -1.021653543253323138, 0.07405724077823318263 ) ) ;
#28863=VERTEX_POINT ( 'NONE', #44126 ) ;
#28879=CARTESIAN_POINT ( 'NONE',  ( 0.07405724077823318263, 0.06102362210100767403, -0.1787899950787401604 ) ) ;
#28889=CARTESIAN_POINT ( 'NONE',  ( -0.07405724077823318263, -1.229454676890656684, 0.1787899950787401604 ) ) ;
#28891=CARTESIAN_POINT ( 'NONE',  ( -0.07405724077823318263, -0.3080708660879689087, 0.1787899950787401604 ) ) ;
#28898=CARTESIAN_POINT ( 'NONE',  ( 3.284318927891251994E-17, -1.609744094434425232, 0.1787899950787401882 ) ) ;
#28899=CARTESIAN_POINT ( 'NONE',  ( -0.07405724077823318263, -0.7460629920722210429, 0.1787899950787401604 ) ) ;
#28927=CARTESIAN_POINT ( 'NONE',  ( 0.1787899950787401604, -0.01771653537930737918, -0.07405724077823318263 ) ) ;
#28932=CARTESIAN_POINT ( 'NONE',  ( 0.2227678560578173761, 0.05525422739377827686, 0.1568179892043651547 ) ) ;
#28933=CARTESIAN_POINT ( 'NONE',  ( 0.1550311931539155308, -0.09383642490574112260, -0.1959255884474807308 ) ) ;
#28938=CARTESIAN_POINT ( 'NONE',  ( -0.1574803149606297803, 0.1028543308161884856, 0.06523048226347956391 ) ) ;
#28947=CARTESIAN_POINT ( 'NONE',  ( -0.1787899950787401604, -0.8406751493316020341, 0.07405724077823318263 ) ) ;
#28949=CARTESIAN_POINT ( 'NONE',  ( 0.02510167551635381772, -0.08956215230678916950, 0.1488583647765791274 ) ) ;
#28957=EDGE_CURVE ( 'NONE', #10382, #36909, #2958, .T. ) ;
#28964=CARTESIAN_POINT ( 'NONE',  ( -0.07444174185955065859, -0.7958115261184778300, -0.1797182628040039087 ) ) ;
#28968=CARTESIAN_POINT ( 'NONE',  ( -0.06523048226347956391, -0.6648622047244090449, -0.1574803149606300301 ) ) ;
#28969=CARTESIAN_POINT ( 'NONE',  ( -0.1203200820771420931, 0.1234194735009758043, -0.1070349918020434971 ) ) ;
#28974=CARTESIAN_POINT ( 'NONE',  ( 0.2471922904502826812, -0.03219022224904102836, -0.1427165354330708902 ) ) ;
#28976=CARTESIAN_POINT ( 'NONE',  ( -0.06523048226347956391, -0.6402559054042833431, 0.1574803149606297803 ) ) ;
#28979=CARTESIAN_POINT ( 'NONE',  ( 0.1264236179284866091, -0.6845472440407243120, -0.1264236179284866091 ) ) ;
#28987=CARTESIAN_POINT ( 'NONE',  ( 0.1787899950787401604, -1.287401574749386768, 0.07405724077823318263 ) ) ;
#28988=CARTESIAN_POINT ( 'NONE',  ( 0.1113553986120547346, -1.469488188976377785, 0.1113553986120547346 ) ) ;
#28995=EDGE_LOOP ( 'NONE', ( #16257, #24419, #20932, #18466 ) ) ;
#28996=CARTESIAN_POINT ( 'NONE',  ( -0.06523048226347956391, -1.427657480207433771, 0.1574803149606297803 ) ) ;
#29006=CARTESIAN_POINT ( 'NONE',  ( 0.1787899950787401604, -0.4322105824024667364, 0.07405724077823318263 ) ) ;
#29007=CARTESIAN_POINT ( 'NONE',  ( -0.03606586445802484331, -0.09842519685039370636, 0.1546304134225889859 ) ) ;
#29016=CARTESIAN_POINT ( 'NONE',  ( -0.1787899950787401604, -1.110236220418677533, -0.07405724077823318263 ) ) ;
#29017=CARTESIAN_POINT ( 'NONE',  ( -0.1264236179284866091, -1.383366141678519678, -0.1264236179284866091 ) ) ;
#29023=CARTESIAN_POINT ( 'NONE',  ( -0.1113553986120547346, -0.1505905511811023723, -0.1113553986120547346 ) ) ;
#29034=CARTESIAN_POINT ( 'NONE',  ( 0.1264236179284866091, -0.02509842514308689362, 0.1264236179284866091 ) ) ;
#29038=CARTESIAN_POINT ( 'NONE',  ( 0.1574803149606300301, -1.457185039262550719, 0.06523048226347956391 ) ) ;
#29039=CARTESIAN_POINT ( 'NONE',  ( 0.1787899950787401604, -0.6968503936470246130, 0.07405724077823318263 ) ) ;
#29041=CARTESIAN_POINT ( 'NONE',  ( -0.1574803149606300301, -1.053641732283463917, -0.06523048226347956391 ) ) ;
#29061=CARTESIAN_POINT ( 'NONE',  ( 0.1574803149606300301, -0.2317913384751499328, -0.06523048226347956391 ) ) ;
#29066=CARTESIAN_POINT ( 'NONE',  ( 0.1352647019381153504, -0.09851384554447126241, -0.1450745768490925292 ) ) ;
#29070=CARTESIAN_POINT ( 'NONE',  ( 0.1264236179284866091, -1.694513732008765983, 0.1264236179284866091 ) ) ;
#29072=VECTOR ( 'NONE', #19801, 39.37007874015748143 ) ;
#29076=CARTESIAN_POINT ( 'NONE',  ( -0.07405724077823318263, -0.9773622046706458288, 0.1787899950787401604 ) ) ;
#29081=CARTESIAN_POINT ( 'NONE',  ( -0.1270800023317771588, -0.2421697938350141632, -0.1270800023317771588 ) ) ;
#29082=CARTESIAN_POINT ( 'NONE',  ( 3.284318927891251994E-17, -0.1246318422449868152, 0.1787899950787401882 ) ) ;
#29083=CARTESIAN_POINT ( 'NONE',  ( 0.1787899950787401882, -0.2957677164816697180, -2.189545951927503898E-17 ) ) ;
#29084=CARTESIAN_POINT ( 'NONE',  ( 0.1787899950787401882, -0.02509842514308689362, -2.189545951927503898E-17 ) ) ;
#29090=CARTESIAN_POINT ( 'NONE',  ( 0.1270800023317771588, -1.787445384386197045, -0.1270800023317771588 ) ) ;
#29099=CARTESIAN_POINT ( 'NONE',  ( 3.284318927891251994E-17, -0.3105314960092286913, 0.1787899950787401882 ) ) ;
#29104=CARTESIAN_POINT ( 'NONE',  ( 0.07405724077823318263, -1.011811023568284451, 0.1787899950787401604 ) ) ;
#29110=EDGE_LOOP ( 'NONE', ( #18451, #41348, #31687, #7599, #21667, #7972, #31266, #24821, #38580, #40584, #18132, #2456, #37205, #42148, #40962, #30689 ) ) ;
#29125=CARTESIAN_POINT ( 'NONE',  ( 0.1264236179284866091, 0.05856299217974780119, -0.1264236179284866091 ) ) ;
#29133=CARTESIAN_POINT ( 'NONE',  ( -0.1787899950787401604, -1.313116094213492069, 0.07405724077823318263 ) ) ;
#29135=CARTESIAN_POINT ( 'NONE',  ( 0.07405724077823318263, -0.2637795275052916555, 0.1787899950787401604 ) ) ;
#29136=CARTESIAN_POINT ( 'NONE',  ( -0.1574803149606299191, 0.02165354341461366364, 0.000000000000000000 ) ) ;
#29141=CARTESIAN_POINT ( 'NONE',  ( -0.2471922026429036467, -0.09209855619639897850, 0.04265916558023801625 ) ) ;
#29144=CARTESIAN_POINT ( 'NONE',  ( 0.1264236179284866091, -1.673720472387181024, -0.1264236179284866091 ) ) ;
#29145=CARTESIAN_POINT ( 'NONE',  ( 0.1264236179284866091, -1.629429133804503937, -0.1264236179284866091 ) ) ;
#29148=CARTESIAN_POINT ( 'NONE',  ( -0.07444174185955065859, -1.292858770212966135, 0.1797182628040039087 ) ) ;
#29157=CARTESIAN_POINT ( 'NONE',  ( -0.1113553986120547346, -0.7706692912310552090, -0.1113553986120547346 ) ) ;
#29173=CARTESIAN_POINT ( 'NONE',  ( -0.1113553986120547346, -1.036417322727118062, 0.1113553986120547346 ) ) ;
#29184=CARTESIAN_POINT ( 'NONE',  ( -0.1787899950787401882, -0.07923228341080354453, 0.000000000000000000 ) ) ;
#29189=CARTESIAN_POINT ( 'NONE',  ( 0.000000000000000000, 0.1299212598425196763, 0.000000000000000000 ) ) ;
#29193=CARTESIAN_POINT ( 'NONE',  ( 0.1574803149606300301, 0.1176181103437474174, 0.06523048226347956391 ) ) ;
#29201=CARTESIAN_POINT ( 'NONE',  ( -0.07405724077823318263, -0.7717775115363263438, -0.1787899950787401604 ) ) ;
#29217=CARTESIAN_POINT ( 'NONE',  ( -0.1270800023317771588, -0.9114611324176910001, -0.1270800023317771588 ) ) ;
#29231=EDGE_CURVE ( 'NONE', #6080, #802, #25212, .T. ) ;
#29240=CARTESIAN_POINT ( 'NONE',  ( 0.1574803149606299191, -1.464566929133858109, -1.928577636452523993E-17 ) ) ;
#29247=CARTESIAN_POINT ( 'NONE',  ( 0.1574803149606299191, 0.1102362204724409434, -1.928577636452523993E-17 ) ) ;
#29257=CARTESIAN_POINT ( 'NONE',  ( 0.1006676817877055763, -0.09658349877441900488, -0.2273124399501114945 ) ) ;
#29258=CARTESIAN_POINT ( 'NONE',  ( 0.08837071341806096436, 0.09266989036297287874, -0.2344122156857449679 ) ) ;
#29260=CARTESIAN_POINT ( 'NONE',  ( -0.1264236179284866091, -0.3362460154733335482, -0.1264236179284866091 ) ) ;
#29261=CARTESIAN_POINT ( 'NONE',  ( -0.1127940203827588611, -0.09842519685039370636, -0.1442820423458218704 ) ) ;
#29270=CARTESIAN_POINT ( 'NONE',  ( 0.1264236179284866091, -1.171751968450173154, 0.1264236179284866091 ) ) ;
#29271=CARTESIAN_POINT ( 'NONE',  ( 3.284318927891251994E-17, -1.329232283410803239, 0.1787899950787401882 ) ) ;
#29275=CARTESIAN_POINT ( 'NONE',  ( -0.1574803149606300301, -0.1087598425196850405, -0.06523048226347956391 ) ) ;
#29280=CARTESIAN_POINT ( 'NONE',  ( -0.1787899950787401604, -0.1998031495525358359, 0.07405724077823318263 ) ) ;
#29290=CARTESIAN_POINT ( 'NONE',  ( 3.284318927891251994E-17, -1.526082677111590513, 0.1787899950787401882 ) ) ;
#29291=CARTESIAN_POINT ( 'NONE',  ( -0.06523048226347956391, -1.599901574695621109, -0.1574803149606300301 ) ) ;
#29292=CARTESIAN_POINT ( 'NONE',  ( 0.1787899950787401882, -0.7731299212060788184, -2.189545951927503898E-17 ) ) ;
#29294=CARTESIAN_POINT ( 'NONE',  ( -0.1574803149606299191, -1.011811023622047223, 0.000000000000000000 ) ) ;
#29314=ORIENTED_EDGE ( 'NONE', *, *, #26497, .F. ) ;
#29318=CARTESIAN_POINT ( 'NONE',  ( -0.1516630832887128078, -0.09851383746137795661, -0.09563143930829449968 ) ) ;
#29328=CARTESIAN_POINT ( 'NONE',  ( 0.07405724077823318263, -0.8395669290800948925, -0.1787899950787401604 ) ) ;
#29334=CARTESIAN_POINT ( 'NONE',  ( -0.07444174185955065859, -0.1658902662759589863, -0.1797182628040039087 ) ) ;
#29336=CARTESIAN_POINT ( 'NONE',  ( -0.07405724077823318263, -0.1270924721662466672, 0.1787899950787401604 ) ) ;
#29337=CARTESIAN_POINT ( 'NONE',  ( -0.1787899950787401882, -0.3154527558517483676, 0.000000000000000000 ) ) ;
#29338=CARTESIAN_POINT ( 'NONE',  ( 0.1787899950787401604, -0.1062992125446616531, 0.07405724077823318263 ) ) ;
#29339=CARTESIAN_POINT ( 'NONE',  ( 0.2471911387363326384, -0.08795568039105847169, -0.05508755932581143461 ) ) ;
#29347=CARTESIAN_POINT ( 'NONE',  ( -0.1878058820398608997, -0.07958416565558186495, 0.1770032286857264603 ) ) ;
#29350=AXIS2_PLACEMENT_3D ( 'NONE', #24179, #7766, #36774 ) ;
#29354=CARTESIAN_POINT ( 'NONE',  ( 0.1264236179284866091, -0.2268700786863941110, 0.1264236179284866091 ) ) ;
#29356=CARTESIAN_POINT ( 'NONE',  ( 0.07405724077823318263, -1.129921259788756682, 0.1787899950787401604 ) ) ;
#29365=CARTESIAN_POINT ( 'NONE',  ( 0.1574803149606300301, -1.142224409341292768, 0.06523048226347956391 ) ) ;
#29375=ORIENTED_EDGE ( 'NONE', *, *, #19965, .T. ) ;
#29376=CARTESIAN_POINT ( 'NONE',  ( 0.07405724077823318263, -0.01771653537930735142, -0.1787899950787401604 ) ) ;
#29383=CARTESIAN_POINT ( 'NONE',  ( -0.1787899950787401604, -1.273746015473333992, 0.07405724077823318263 ) ) ;
#29385=CARTESIAN_POINT ( 'NONE',  ( -1.094772975963752103E-17, -0.3252952755367877757, -0.1787899950787401882 ) ) ;
#29390=CARTESIAN_POINT ( 'NONE',  ( -0.2471883443660232993, -0.06218794471711499433, 0.1039611462668204589 ) ) ;
#29393=CARTESIAN_POINT ( 'NONE',  ( 0.1787899950787401604, -1.597440944828127485, -0.07405724077823318263 ) ) ;
#29394=CARTESIAN_POINT ( 'NONE',  ( -0.07405724077823318263, -1.725393700733637958, 0.1787899950787401604 ) ) ;
#29398=CARTESIAN_POINT ( 'NONE',  ( -0.08595198851647926908, -0.09842519685039370636, 0.1380468394703990020 ) ) ;
#29399=CARTESIAN_POINT ( 'NONE',  ( -0.1797182628040039365, -1.457720974937376068, 0.000000000000000000 ) ) ;
#29416=ORIENTED_EDGE ( 'NONE', *, *, #28594, .T. ) ;
#29425=CARTESIAN_POINT ( 'NONE',  ( 0.1787899950787401604, -0.2194881889226144023, 0.07405724077823318263 ) ) ;
#29429=CARTESIAN_POINT ( 'NONE',  ( -9.642888182262618425E-18, 0.08070866141732284393, -0.1574803149606299191 ) ) ;
#29430=CARTESIAN_POINT ( 'NONE',  ( -0.1235961452251413406, 0.09842519685039370636, 0.2140748031496062798 ) ) ;
#29434=CARTESIAN_POINT ( 'NONE',  ( -0.06523048226347956391, 0.05364173239099160467, -0.1574803149606300301 ) ) ;
#29439=CARTESIAN_POINT ( 'NONE',  ( -1.094772975963752103E-17, -0.8923483776780569698, -0.1787899950787401882 ) ) ;
#29452=CARTESIAN_POINT ( 'NONE',  ( -0.1797182628040039087, -0.9090005024964308289, -0.07444174185955065859 ) ) ;
#29463=CARTESIAN_POINT ( 'NONE',  ( -0.1574803149606300301, -0.6500984250893240279, -0.06523048226347956391 ) ) ;
#29465=CARTESIAN_POINT ( 'NONE',  ( -0.1264236179284866091, -0.7534448818360000022, -0.1264236179284866091 ) ) ;
#29472=CARTESIAN_POINT ( 'NONE',  ( 0.1574803149606300301, -1.703248031496063408, 0.06523048226347956391 ) ) ;
#29476=VECTOR ( 'NONE', #8211, 39.37007874015748143 ) ;
#29479=ORIENTED_EDGE ( 'NONE', *, *, #4304, .F. ) ;
#29489=CARTESIAN_POINT ( 'NONE',  ( 0.05557684098944757484, 0.07733267719194691914, -0.2533457667601751173 ) ) ;
#29492=CARTESIAN_POINT ( 'NONE',  ( -0.07405724077823318263, -0.3387066453945931643, -0.1787899950787401604 ) ) ;
#29493=CARTESIAN_POINT ( 'NONE',  ( 0.1110370215561167356, -0.09842519685039370636, 0.09588239823699959419 ) ) ;
#29502=CARTESIAN_POINT ( 'NONE',  ( 0.1787899950787401604, -1.400590551127339323, -0.07405724077823318263 ) ) ;
#29503=CARTESIAN_POINT ( 'NONE',  ( 0.1787899950787401882, -1.437499999946236340, -2.189545951927503898E-17 ) ) ;
#29511=CARTESIAN_POINT ( 'NONE',  ( -0.1574803149606300301, -0.3449803149606298636, -0.06523048226347956391 ) ) ;
#29521=CARTESIAN_POINT ( 'NONE',  ( -0.1574803149606300301, 0.09793307097366883707, -0.06523048226347956391 ) ) ;
#29522=CARTESIAN_POINT ( 'NONE',  ( -1.094772975963752103E-17, -1.585137795221826629, -0.1787899950787401882 ) ) ;
#29523=CARTESIAN_POINT ( 'NONE',  ( -0.1113553986120547346, -1.469488188868850465, 0.1113553986120547346 ) ) ;
#29524=CARTESIAN_POINT ( 'NONE',  ( -0.1264236179284866091, -0.7977362204186770889, -0.1264236179284866091 ) ) ;
#29525=CARTESIAN_POINT ( 'NONE',  ( -0.1574803149606299191, -1.090551181102362266, 0.000000000000000000 ) ) ;
#29551=CARTESIAN_POINT ( 'NONE',  ( -0.06938717807759606226, -0.09851383877177855020, -0.1728648718439755871 ) ) ;
#29558=ORIENTED_EDGE ( 'NONE', *, *, #2117, .F. ) ;
#29561=CARTESIAN_POINT ( 'NONE',  ( -0.07405724077823318263, -0.4458661416785199560, -0.1787899950787401604 ) ) ;
#29562=CARTESIAN_POINT ( 'NONE',  ( -0.07405724077823318263, -0.9379921259304876413, 0.1787899950787401604 ) ) ;
#29567=CARTESIAN_POINT ( 'NONE',  ( -0.1797182628040039087, -0.1166776678507620985, 0.07444174185955065859 ) ) ;
#29575=DIRECTION ( 'NONE',  ( 0.000000000000000000, -1.000000000000000000, 0.000000000000000000 ) ) ;
#29585=CARTESIAN_POINT ( 'NONE',  ( -0.1113553986120547346, -0.9576771652468032414, 0.1113553986120547346 ) ) ;
#29586=CARTESIAN_POINT ( 'NONE',  ( -0.07405724077823318263, -0.2883858267178899260, -0.1787899950787401604 ) ) ;
#29589=CARTESIAN_POINT ( 'NONE',  ( -0.07405724077823318263, -1.095472440891117838, 0.1787899950787401604 ) ) ;
#29614=CARTESIAN_POINT ( 'NONE',  ( -0.1787899950787401882, -1.433686960355222473, 0.000000000000000000 ) ) ;
#29617=CARTESIAN_POINT ( 'NONE',  ( 0.1264236179284866091, -0.2514763778989925203, -0.1264236179284866091 ) ) ;
#29626=CARTESIAN_POINT ( 'NONE',  ( -0.1787899950787401882, -1.658956692859621995, 0.000000000000000000 ) ) ;
#29627=CARTESIAN_POINT ( 'NONE',  ( -0.1787899950787401882, -1.654035433017102319, 0.000000000000000000 ) ) ;
#29630=CARTESIAN_POINT ( 'NONE',  ( 3.301370929368692659E-17, -1.408508376512179083, 0.1797182628040039365 ) ) ;
#29634=CARTESIAN_POINT ( 'NONE',  ( -0.09686282429646721204, 0.1299212598425196763, 0.1372510960255870494 ) ) ;
#29649=CARTESIAN_POINT ( 'NONE',  ( 0.1797182628040039087, -0.09699262848068328224, -0.07444174185955065859 ) ) ;
#29658=CARTESIAN_POINT ( 'NONE',  ( 0.1787899950787401604, -0.1407480314422995815, 0.07405724077823318263 ) ) ;
#29662=CARTESIAN_POINT ( 'NONE',  ( -0.08837038158045873448, -0.09266989036297303139, 0.2344124146308562417 ) ) ;
#29667=CARTESIAN_POINT ( 'NONE',  ( 0.1574803149606299191, 0.04133858278469235842, -1.928577636452523993E-17 ) ) ;
#29674=FACE_OUTER_BOUND ( 'NONE', #28995, .T. ) ;
#29675=CARTESIAN_POINT ( 'NONE',  ( 0.1264236179284866091, -0.9071121572056161098, 0.1264236179284866091 ) ) ;
#29684=CARTESIAN_POINT ( 'NONE',  ( 0.1270800023317771588, -1.009886329268084637, 0.1270800023317771588 ) ) ;
#29697=CARTESIAN_POINT ( 'NONE',  ( 0.1264236179284866091, -0.7239173227808818334, -0.1264236179284866091 ) ) ;
#29708=CARTESIAN_POINT ( 'NONE',  ( -9.642888182262618425E-18, 0.05118110246973173183, -0.1574803149606299191 ) ) ;
#29716=DIRECTION ( 'NONE',  ( 0.000000000000000000, 0.000000000000000000, 1.000000000000000000 ) ) ;
#29717=CARTESIAN_POINT ( 'NONE',  ( -1.094772975963752103E-17, -0.3805373540560102463, -0.1787899950787401882 ) ) ;
#29718=CARTESIAN_POINT ( 'NONE',  ( -0.2212350913337720881, -0.08955973899257303750, -0.09908300582586200556 ) ) ;
#29728=CARTESIAN_POINT ( 'NONE',  ( -0.1264236179284866091, -1.309547244040724312, -0.1264236179284866091 ) ) ;
#29730=CARTESIAN_POINT ( 'NONE',  ( -0.07405724077823318263, -1.489173228292693718, 0.1787899950787401604 ) ) ;
#29738=CARTESIAN_POINT ( 'NONE',  ( 0.1574803149606300301, -0.2465551181102364486, 0.06523048226347956391 ) ) ;
#29746=CARTESIAN_POINT ( 'NONE',  ( -0.1670491933469263335, -0.08956140236111079234, 0.01966157176086386418 ) ) ;
#29751=CARTESIAN_POINT ( 'NONE',  ( 0.1787899950787401604, -1.592519684985606254, -0.07405724077823318263 ) ) ;
#29752=CARTESIAN_POINT ( 'NONE',  ( -0.1787899950787401604, -0.7559055117572593963, -0.07405724077823318263 ) ) ;
#29753=CARTESIAN_POINT ( 'NONE',  ( -0.1574803149606300301, -1.171751968503937924, -0.06523048226347956391 ) ) ;
#29777=CARTESIAN_POINT ( 'NONE',  ( -0.1028960859539838624, -0.09851383303946475989, 0.1274171143542842388 ) ) ;
#29783=CARTESIAN_POINT ( 'NONE',  ( -0.1264236179284866091, -0.8272637794737952577, 0.1264236179284866091 ) ) ;
#29785=CARTESIAN_POINT ( 'NONE',  ( 0.1264236179284866091, -0.4138779527021417826, -0.1264236179284866091 ) ) ;
#29786=CARTESIAN_POINT ( 'NONE',  ( -0.1264236179284866091, -1.107775590497417362, -0.1264236179284866091 ) ) ;
#29791=CARTESIAN_POINT ( 'NONE',  ( 0.07444174185955046430, -0.1708115261184786626, -0.1797182628040039087 ) ) ;
#29795=SURFACE_STYLE_FILL_AREA ( #7464 ) ;
#29796=CARTESIAN_POINT ( 'NONE',  ( -0.1797182628040039365, -1.812051683598795648, 0.000000000000000000 ) ) ;
#29804=CARTESIAN_POINT ( 'NONE',  ( -0.07405724077823318263, -0.2096456692375751329, -0.1787899950787401604 ) ) ;
#29806=CARTESIAN_POINT ( 'NONE',  ( -0.1264236179284866091, -1.176673228292692830, 0.1264236179284866091 ) ) ;
#29816=CARTESIAN_POINT ( 'NONE',  ( -9.642888182262618425E-18, -1.169291338475149544, -0.1574803149606299191 ) ) ;
#29827=CARTESIAN_POINT ( 'NONE',  ( -0.1787899950787401882, -0.08415354325332302654, 0.000000000000000000 ) ) ;
#29836=CARTESIAN_POINT ( 'NONE',  ( -0.1264236179284866091, -1.477978298937899559, -0.1264236179284866091 ) ) ;
#29838=CARTESIAN_POINT ( 'NONE',  ( 0.1787899950787401604, -0.4950787401037172186, 0.07405724077823318263 ) ) ;
#29840=ORIENTED_EDGE ( 'NONE', *, *, #2059, .T. ) ;
#29847=CARTESIAN_POINT ( 'NONE',  ( -0.1787899950787401604, -1.577755905458046115, 0.07405724077823318263 ) ) ;
#29848=CARTESIAN_POINT ( 'NONE',  ( 0.1787899950787401604, -1.676181102308441639, 0.07405724077823318263 ) ) ;
#29854=CARTESIAN_POINT ( 'NONE',  ( -9.642888182262618425E-18, -0.5492125984251968740, -0.1574803149606299191 ) ) ;
#29856=CARTESIAN_POINT ( 'NONE',  ( 0.1797182628040039365, -1.359295778086982320, -2.200913952912460540E-17 ) ) ;
#29874=CARTESIAN_POINT ( 'NONE',  ( 0.1270800023317771588, -0.02563436076414791348, 0.1270800023317771588 ) ) ;
#29875=CARTESIAN_POINT ( 'NONE',  ( 0.1574803149606300301, -1.058562992018457827, -0.06523048226347956391 ) ) ;
#29876=CARTESIAN_POINT ( 'NONE',  ( 0.1787899950787401882, -1.206200787347811110, -2.189545951927503898E-17 ) ) ;
#29882=CARTESIAN_POINT ( 'NONE',  ( -0.1787899950787401882, -0.1186023621509610243, 0.000000000000000000 ) ) ;
#29887=CARTESIAN_POINT ( 'NONE',  ( -0.06215339161682907620, -0.08126078924469150311, 0.2495487439735979418 ) ) ;
#29889=CARTESIAN_POINT ( 'NONE',  ( 2.892866454678787531E-17, -0.007874015640504449659, 0.1574803149606299191 ) ) ;
#29896=CARTESIAN_POINT ( 'NONE',  ( 0.07405724077823318263, -0.9341790863394755506, -0.1787899950787401604 ) ) ;
#29903=CARTESIAN_POINT ( 'NONE',  ( 3.284318927891251994E-17, -0.5073818897100158543, 0.1787899950787401882 ) ) ;
#29909=CARTESIAN_POINT ( 'NONE',  ( 0.07444174185955046430, -1.076323337142101266, -0.1797182628040039087 ) ) ;
#29925=CARTESIAN_POINT ( 'NONE',  ( 0.07405724077823318263, -0.7214566928596228834, -0.1787899950787401604 ) ) ;
#29931=CARTESIAN_POINT ( 'NONE',  ( 0.1574803149606299191, -1.661417322834645827, -1.928577636452523993E-17 ) ) ;
#29934=FACE_OUTER_BOUND ( 'NONE', #34545, .T. ) ;
#29937=CARTESIAN_POINT ( 'NONE',  ( -0.1113553986120547346, 0.05610236231225141507, -0.1113553986120547346 ) ) ;
#29938=CARTESIAN_POINT ( 'NONE',  ( -0.1113553986120547346, -0.2883858266641263768, 0.1113553986120547346 ) ) ;
#29945=CARTESIAN_POINT ( 'NONE',  ( 0.08776479879009585483, 0.09247100924357745666, -0.2347620406593065867 ) ) ;
#29947=CARTESIAN_POINT ( 'NONE',  ( -0.1264236179284866091, -0.4937263304339629677, -0.1264236179284866091 ) ) ;
#29948=CARTESIAN_POINT ( 'NONE',  ( -0.2086609251499436934, -0.08955986906679389015, 0.1029602451354245940 ) ) ;
#29949=FACE_OUTER_BOUND ( 'NONE', #18000, .T. ) ;
#29960=CARTESIAN_POINT ( 'NONE',  ( -0.1264236179284866091, -1.260334645615527549, 0.1264236179284866091 ) ) ;
#29961=CARTESIAN_POINT ( 'NONE',  ( -0.1264236179284866091, -1.580216535379306952, -0.1264236179284866091 ) ) ;
#29970=CARTESIAN_POINT ( 'NONE',  ( 0.06523048226347956391, -0.2367125984251967630, -0.1574803149606300301 ) ) ;
#29980=CARTESIAN_POINT ( 'NONE',  ( -0.1512883101241234984, -0.08956046692967721545, 0.06580901924223876709 ) ) ;
#29988=CARTESIAN_POINT ( 'NONE',  ( -0.1264236179284866091, -1.619586614119464585, -0.1264236179284866091 ) ) ;
#29989=CARTESIAN_POINT ( 'NONE',  ( 0.07405724077823318263, -0.8051181101824581576, -0.1787899950787401604 ) ) ;
#29991=CARTESIAN_POINT ( 'NONE',  ( 0.1574803149606300301, -1.152066929133859219, 0.06523048226347956391 ) ) ;
#29995=ORIENTED_EDGE ( 'NONE', *, *, #21087, .F. ) ;
#29998=CARTESIAN_POINT ( 'NONE',  ( 0.1574803149606300301, -1.334153543199559699, -0.06523048226347956391 ) ) ;
#30012=CARTESIAN_POINT ( 'NONE',  ( -0.2245921208055326745, -0.09842519685039370636, -0.1004051365227200815 ) ) ;
#30021=CARTESIAN_POINT ( 'NONE',  ( 0.07405724077823318263, -0.8986220471903317852, 0.1787899950787401604 ) ) ;
#30022=CARTESIAN_POINT ( 'NONE',  ( 0.1787899950787401882, -1.004429133804503937, -2.189545951927503898E-17 ) ) ;
#30027=CARTESIAN_POINT ( 'NONE',  ( 0.07444174185955065859, -0.3036855418665100892, 0.1797182628040039087 ) ) ;
#30039=CARTESIAN_POINT ( 'NONE',  ( -0.1787899950787401604, -0.2785433070328505734, 0.07405724077823318263 ) ) ;
#30041=CARTESIAN_POINT ( 'NONE',  ( -0.1264236179284866091, -1.294783464513165283, 0.1264236179284866091 ) ) ;
#30049=CARTESIAN_POINT ( 'NONE',  ( 0.1574803149606300301, -1.220964566821607145, 0.06523048226347956391 ) ) ;
#30054=CARTESIAN_POINT ( 'NONE',  ( -0.1076092635444119150, -0.09842303418682271654, -0.1430890476085535934 ) ) ;
#30059=ORIENTED_EDGE ( 'NONE', *, *, #4790, .T. ) ;
#30067=CARTESIAN_POINT ( 'NONE',  ( -0.2087179188330661184, -0.09851385215208996460, -0.1330443330087964504 ) ) ;
#30072=CARTESIAN_POINT ( 'NONE',  ( 0.07405724077823318263, -1.406620031221363476, -0.1787899950787401604 ) ) ;
#30074=CARTESIAN_POINT ( 'NONE',  ( -0.1787899950787401604, -0.5098425196312756924, 0.07405724077823318263 ) ) ;
#30076=CARTESIAN_POINT ( 'NONE',  ( 2.892866454678787531E-17, 0.03149606309965303358, 0.1574803149606299191 ) ) ;
#30083=EDGE_CURVE ( 'NONE', #40254, #6080, #25607, .T. ) ;
#30088=CARTESIAN_POINT ( 'NONE',  ( -0.1787899950787401604, 0.1042067404321787294, 0.07405724077823318263 ) ) ;
#30089=CARTESIAN_POINT ( 'NONE',  ( 0.1787899950787401604, -1.636811023568283341, 0.07405724077823318263 ) ) ;
#30095=CARTESIAN_POINT ( 'NONE',  ( 0.06523048226347956391, -0.7239173228346461597, 0.1574803149606297803 ) ) ;
#30097=CARTESIAN_POINT ( 'NONE',  ( -0.1797182628040039087, -1.455260345016115231, 0.07444174185955065859 ) ) ;
#30098=FACE_OUTER_BOUND ( 'NONE', #23586, .T. ) ;
#30099=CONICAL_SURFACE ( 'NONE', #36187, 0.2471922904502826812, 0.5235987755982992597 ) ;
#30100=CARTESIAN_POINT ( 'NONE',  ( 0.2471922904502826257, 0.09842519685039370636, -0.01310751975302622621 ) ) ;
#30105=CARTESIAN_POINT ( 'NONE',  ( 0.1787899950787401882, 0.1323818898175431191, -2.189545951927503898E-17 ) ) ;
#30116=CARTESIAN_POINT ( 'NONE',  ( -0.1270800023317771588, -0.005949321394069172729, -0.1270800023317771588 ) ) ;
#30117=CARTESIAN_POINT ( 'NONE',  ( 0.07405724077823318263, -1.213582677111591623, 0.1787899950787401604 ) ) ;
#30120=CARTESIAN_POINT ( 'NONE',  ( -0.1113553986120547346, 0.05610236220472441387, 0.1113553986120547346 ) ) ;
#30123=CARTESIAN_POINT ( 'NONE',  ( 0.1787899950787401604, -0.1801181101824570474, 0.07405724077823318263 ) ) ;
#30124=B_SPLINE_CURVE_WITH_KNOTS ( 'NONE', 3,
 ( #21114, #3569, #14593, #11009, #25629, #27055, #34009, #4974, #37818, #11721, #37327, #26341, #22717, #23443, #40902, #30892, #19354, #4729, #9053, #38048, #891 ),
 .UNSPECIFIED., .F., .F.,
 ( 4, 2, 1, 1, 2, 2, 2, 1, 1, 1, 2, 2, 4 ),
 ( 0.000000000000000000, 0.1249999999999998890, 0.1874999999999997780, 0.2187499999999997502, 0.2343749999999997780, 0.2499999999999997780, 0.3750000000000000000, 0.4375000000000002220, 0.4687500000000002220, 0.4843750000000002220, 0.4921875000000001665, 0.5000000000000001110, 1.000000000000000000 ),
 .UNSPECIFIED. ) ;
#30126=CARTESIAN_POINT ( 'NONE',  ( 0.06523048226347956391, -0.1087598424121580948, -0.1574803149606300301 ) ) ;
#30133=CARTESIAN_POINT ( 'NONE',  ( 0.07405724077823318263, -1.027683023347349289, 0.1787899950787401604 ) ) ;
#30135=CARTESIAN_POINT ( 'NONE',  ( 0.1787899950787401882, 0.05856299217974772486, -2.189545951927503898E-17 ) ) ;
#30142=CARTESIAN_POINT ( 'NONE',  ( -1.094772975963752103E-17, -0.4876968503399370380, -0.1787899950787401882 ) ) ;
#30148=CARTESIAN_POINT ( 'NONE',  ( -0.1797182628040039087, -1.022189478874383495, 0.07444174185955065859 ) ) ;
#30160=CARTESIAN_POINT ( 'NONE',  ( -0.07405724077823318263, -0.7559055117572593963, -0.1787899950787401604 ) ) ;
#30169=CARTESIAN_POINT ( 'NONE',  ( 2.892866454678787531E-17, -1.710629921259842590, 0.1574803149606299191 ) ) ;
#30178=VERTEX_POINT ( 'NONE', #47159 ) ;
#30179=CARTESIAN_POINT ( 'NONE',  ( 0.07405724077823318263, -1.489173228292693718, 0.1787899950787401604 ) ) ;
#30187=CARTESIAN_POINT ( 'NONE',  ( 0.1787899950787401604, -0.6290609761032543990, 0.07405724077823318263 ) ) ;
#30188=CARTESIAN_POINT ( 'NONE',  ( 0.05257954919166763635, -0.08956008031886615595, 0.2115869642176704812 ) ) ;
#30189=CARTESIAN_POINT ( 'NONE',  ( 0.1574803149606300301, 0.03887795286343254109, 0.06523048226347956391 ) ) ;
#30199=CARTESIAN_POINT ( 'NONE',  ( -0.1787899950787401604, -1.385826771599779184, -0.07405724077823318263 ) ) ;
#30200=CARTESIAN_POINT ( 'NONE',  ( -0.1264236179284866091, -1.491633858213953001, 0.1264236179284866091 ) ) ;
#30208=CARTESIAN_POINT ( 'NONE',  ( 0.1113553986120547346, -0.3179133858267716994, -0.1113553986120547346 ) ) ;
#30217=CARTESIAN_POINT ( 'NONE',  ( -0.1556638648389445378, -0.08956154917608123711, 0.05664513584083256947 ) ) ;
#30222=CARTESIAN_POINT ( 'NONE',  ( -0.1787899950787401604, -1.612204724355685403, 0.07405724077823318263 ) ) ;
#30223=CARTESIAN_POINT ( 'NONE',  ( 0.1787899950787401604, -0.8937007873478103326, 0.07405724077823318263 ) ) ;
#30224=CARTESIAN_POINT ( 'NONE',  ( -0.1574803149606299191, -1.208661417322834719, 0.000000000000000000 ) ) ;
#30246=CARTESIAN_POINT ( 'NONE',  ( -0.1637653116087653404, -0.09842519685039370636, 0.1653323808283389817 ) ) ;
#30251=ORIENTED_EDGE ( 'NONE', *, *, #15672, .T. ) ;
#30257=CARTESIAN_POINT ( 'NONE',  ( 0.1787899950787401604, -0.9330708660879686311, 0.07405724077823318263 ) ) ;
#30258=CARTESIAN_POINT ( 'NONE',  ( -0.07405724077823318263, -1.016732283410803905, 0.1787899950787401604 ) ) ;
#30261=CARTESIAN_POINT ( 'NONE',  ( -0.07444174185955065859, -0.2840005024964313840, -0.1797182628040039087 ) ) ;
#30263=CARTESIAN_POINT ( 'NONE',  ( 0.1787899950787401604, -0.1456692912848192578, 0.07405724077823318263 ) ) ;
#30272=CARTESIAN_POINT ( 'NONE',  ( -0.1787899950787401604, -0.4360236219934807145, 0.07405724077823318263 ) ) ;
#30274=CARTESIAN_POINT ( 'NONE',  ( -0.1787899950787401604, -1.302165354276944242, -0.07405724077823318263 ) ) ;
#30282=CARTESIAN_POINT ( 'NONE',  ( -0.1574803149606300301, -1.201279527451527995, -0.06523048226347956391 ) ) ;
#30287=CARTESIAN_POINT ( 'NONE',  ( -0.03626583649048213676, -0.09844386080825558161, -0.1760747600047917194 ) ) ;
#30297=CARTESIAN_POINT ( 'NONE',  ( -0.2341231448849070973, -0.09851385138007755227, -0.07098514503060590619 ) ) ;
#30303=CARTESIAN_POINT ( 'NONE',  ( -0.1787899950787401604, -1.470596409174119934, 0.07405724077823318263 ) ) ;
#30305=CARTESIAN_POINT ( 'NONE',  ( -0.07405724077823318263, -0.4261811023084413064, 0.1787899950787401604 ) ) ;
#30315=CARTESIAN_POINT ( 'NONE',  ( -0.07405724077823318263, -1.745078740103716886, -0.1787899950787401604 ) ) ;
#30316=CARTESIAN_POINT ( 'NONE',  ( -0.1787899950787401882, -1.811515747977732405, 0.000000000000000000 ) ) ;
#30321=CARTESIAN_POINT ( 'NONE',  ( 0.1574803149606300301, -0.7534448818897636624, -0.06523048226347956391 ) ) ;
#30323=CARTESIAN_POINT ( 'NONE',  ( -0.1797182628040039365, -1.378980817457061026, 0.000000000000000000 ) ) ;
#30344=CARTESIAN_POINT ( 'NONE',  ( -1.100456976456230270E-17, -0.01087058123658885857, -0.1797182628040039365 ) ) ;
#30346=CARTESIAN_POINT ( 'NONE',  ( 3.284318927891251994E-17, -1.137303149552535420, 0.1787899950787401882 ) ) ;
#30358=CARTESIAN_POINT ( 'NONE',  ( -0.07051875723980910449, -0.08549467455823119011, -0.2447177463901700212 ) ) ;
#30359=CARTESIAN_POINT ( 'NONE',  ( -0.1113553986120547346, -0.05216535422318158144, 0.1113553986120547346 ) ) ;
#30369=CARTESIAN_POINT ( 'NONE',  ( -1.094772975963752103E-17, -1.049828692638687055, -0.1787899950787401882 ) ) ;
#30370=CARTESIAN_POINT ( 'NONE',  ( 0.07405724077823318263, 0.01181102367581074800, 0.1787899950787401604 ) ) ;
#30379=CARTESIAN_POINT ( 'NONE',  ( 0.07444174185955065859, -0.9729768804491867318, 0.1797182628040039087 ) ) ;
#30389=CARTESIAN_POINT ( 'NONE',  ( -0.1787899950787401882, 0.1176181102899840625, 0.000000000000000000 ) ) ;
#30393=CARTESIAN_POINT ( 'NONE',  ( -0.1787899950787401882, -0.9060039369541103005, 0.000000000000000000 ) ) ;
#30397=CARTESIAN_POINT ( 'NONE',  ( -0.06523048226347956391, -1.742618110128693276, 0.1574803149606297803 ) ) ;
#30401=CARTESIAN_POINT ( 'NONE',  ( -0.1113553986120547346, -1.676181102362204856, 0.1113553986120547346 ) ) ;
#30407=CARTESIAN_POINT ( 'NONE',  ( 3.284318927891251994E-17, -1.491633858213953001, 0.1787899950787401882 ) ) ;
#30413=DIRECTION ( 'NONE',  ( 0.000000000000000000, -1.000000000000000000, 0.000000000000000000 ) ) ;
#30416=CARTESIAN_POINT ( 'NONE',  ( -1.094772975963752103E-17, -0.4986475902764826995, -0.1787899950787401882 ) ) ;
#30417=CARTESIAN_POINT ( 'NONE',  ( -0.1613434097111628163, -0.08955965769485689509, 0.1626613769059765680 ) ) ;
#30424=CARTESIAN_POINT ( 'NONE',  ( 0.1787899950787401604, -1.287401574749386768, 0.07405724077823318263 ) ) ;
#30425=CARTESIAN_POINT ( 'NONE',  ( 0.1264236179284866091, -1.560531496009228247, 0.1264236179284866091 ) ) ;
#30432=CARTESIAN_POINT ( 'NONE',  ( 0.1574803149606300301, -0.2810039370078740162, -0.06523048226347956391 ) ) ;
#30435=ORIENTED_EDGE ( 'NONE', *, *, #15672, .F. ) ;
#30437=CARTESIAN_POINT ( 'NONE',  ( -0.1191479377955081548, -0.09019619403132914104, -0.1333268377994320797 ) ) ;
#30440=CARTESIAN_POINT ( 'NONE',  ( 0.000000000000000000, 0.09842519685039370636, 0.000000000000000000 ) ) ;
#30441=CARTESIAN_POINT ( 'NONE',  ( -0.1355115267431857007, -0.08956120344901688513, 0.09056412678083718137 ) ) ;
#30449=CARTESIAN_POINT ( 'NONE',  ( 0.1787899950787401604, -1.715551181048599716, 0.07405724077823318263 ) ) ;
#30450=CARTESIAN_POINT ( 'NONE',  ( 0.1787899950787401604, -0.9330708660879686311, 0.07405724077823318263 ) ) ;
#30451=CARTESIAN_POINT ( 'NONE',  ( -9.642888182262618425E-18, -1.257874015748031482, -0.1574803149606299191 ) ) ;
#30458=CARTESIAN_POINT ( 'NONE',  ( 0.1574803149606300301, -1.378444881782237008, 0.06523048226347956391 ) ) ;
#30467=CARTESIAN_POINT ( 'NONE',  ( 4.801428276353606495E-17, 0.03219022224904102836, 0.2854330708661417804 ) ) ;
#30473=CARTESIAN_POINT ( 'NONE',  ( -0.1264342353168110278, -0.09851383435030748592, 0.1068074073256397583 ) ) ;
#30477=CARTESIAN_POINT ( 'NONE',  ( 3.284318927891251994E-17, -0.8223425196312754704, 0.1787899950787401882 ) ) ;
#30478=( BOUNDED_CURVE ( )  B_SPLINE_CURVE ( 2, ( #20998, #17184, #39208, #21240, #28467, #14064, #35413, #2552, #31819 ),
 .UNSPECIFIED., .F., .T. ) 
 B_SPLINE_CURVE_WITH_KNOTS ( ( 3, 2, 2, 2, 3 ),
 ( 0.08500000000000000611, 0.08749999999999999445, 0.08999999999999999667, 0.09249999999999999889, 0.09500000000000000111 ),
 .UNSPECIFIED. ) 
 CURVE ( )  GEOMETRIC_REPRESENTATION_ITEM ( )  RATIONAL_B_SPLINE_CURVE ( ( 1.000000000000000000, 0.9238795325112869605, 1.000000000000000000, 0.9238795325112869605, 1.000000000000000000, 0.9238795325112869605, 1.000000000000000000, 0.9238795325112869605, 1.000000000000000000 ) ) 
 REPRESENTATION_ITEM ( '' )  ) ;
#30479=CARTESIAN_POINT ( 'NONE',  ( -0.1787899950787401882, -1.102854330654897685, 0.000000000000000000 ) ) ;
#30482=CARTESIAN_POINT ( 'NONE',  ( -0.1270800023317771588, -0.2716973528901322488, 0.1270800023317771588 ) ) ;
#30496=CARTESIAN_POINT ( 'NONE',  ( 0.1787899950787401604, -0.4163385826234020093, -0.07405724077823318263 ) ) ;
#30498=CARTESIAN_POINT ( 'NONE',  ( -1.094772975963752103E-17, -1.309547244040724312, -0.1787899950787401882 ) ) ;
#30508=CARTESIAN_POINT ( 'NONE',  ( 0.05252291220399905175, -0.09842554669817424329, -0.1709337162269513322 ) ) ;
#30525=CARTESIAN_POINT ( 'NONE',  ( -0.1787899950787401604, -1.475517669016641165, -0.07405724077823318263 ) ) ;
#30528=CARTESIAN_POINT ( 'NONE',  ( 0.1264236179284866091, -0.3794291338045042705, 0.1264236179284866091 ) ) ;
#30533=CARTESIAN_POINT ( 'NONE',  ( 0.1787899950787401604, -0.2194881889226144023, -0.07405724077823318263 ) ) ;
#30537=CARTESIAN_POINT ( 'NONE',  ( 3.284318927891251994E-17, -1.727854330654897685, 0.1787899950787401882 ) ) ;
#30540=VERTEX_POINT ( 'NONE', #5423 ) ;
#30544=CARTESIAN_POINT ( 'NONE',  ( 2.892866454678787531E-17, -0.7657480314960629642, 0.1574803149606299191 ) ) ;
#30546=CARTESIAN_POINT ( 'NONE',  ( -0.1270800023317771588, -1.580752471000367976, -0.1270800023317771588 ) ) ;
#30548=CARTESIAN_POINT ( 'NONE',  ( 0.06523048226347956391, -0.4384842518609765039, 0.1574803149606297803 ) ) ;
#30549=CARTESIAN_POINT ( 'NONE',  ( 0.2471922904502826257, 0.09142184925108906568, -0.04493454898960681093 ) ) ;
#30558=CARTESIAN_POINT ( 'NONE',  ( -0.1787899950787401604, 0.1151574803687242243, 0.07405724077823318263 ) ) ;
#30568=CARTESIAN_POINT ( 'NONE',  ( 0.07444174185955046430, -0.09207136863816363370, -0.1797182628040039087 ) ) ;
#30569=CARTESIAN_POINT ( 'NONE',  ( 3.284318927891251994E-17, -1.373523621993480326, 0.1787899950787401882 ) ) ;
#30571=CYLINDRICAL_SURFACE ( 'NONE', #31649, 0.1574803149606299191 ) ;
#30579=CARTESIAN_POINT ( 'NONE',  ( -0.03313107868980413873, -0.09812580651453278735, 0.1546376223675618999 ) ) ;
#30581=CARTESIAN_POINT ( 'NONE',  ( 0.06523048226347956391, -0.08415354319955967166, 0.1574803149606297803 ) ) ;
#30589=CARTESIAN_POINT ( 'NONE',  ( 0.000000000000000000, 0.09842519685039370636, 0.000000000000000000 ) ) ;
#30590=CARTESIAN_POINT ( 'NONE',  ( 0.1264236179284866091, -0.9464822359457736312, 0.1264236179284866091 ) ) ;
#30592=CARTESIAN_POINT ( 'NONE',  ( 0.1264236179284866091, -0.01525590545804753929, -0.1264236179284866091 ) ) ;
#30597=CARTESIAN_POINT ( 'NONE',  ( 0.1787899950787401604, -0.6574803149068665364, 0.07405724077823318263 ) ) ;
#30598=EDGE_CURVE ( 'NONE', #14105, #27412, #6109, .T. ) ;
#30601=CARTESIAN_POINT ( 'NONE',  ( 0.1797182628040039087, -1.046795778086983653, 0.07444174185955046430 ) ) ;
#30610=CARTESIAN_POINT ( 'NONE',  ( 0.1574803149606299191, -0.7066929132782991951, -1.928577636452523993E-17 ) ) ;
#30612=CARTESIAN_POINT ( 'NONE',  ( 0.1264236179284866091, 0.1028543307624250058, -0.1264236179284866091 ) ) ;
#30616=CARTESIAN_POINT ( 'NONE',  ( 0.07405724077823318263, -0.9724409448281265966, 0.1787899950787401604 ) ) ;
#30621=CARTESIAN_POINT ( 'NONE',  ( 0.1574803149606300301, -1.693405511703496957, 0.06523048226347956391 ) ) ;
#30625=CARTESIAN_POINT ( 'NONE',  ( -0.07405724077823318263, 0.1250000000537635492, 0.1787899950787401604 ) ) ;
#30628=( BOUNDED_CURVE ( )  B_SPLINE_CURVE ( 2, ( #39048, #10316, #42857, #28788, #18205, #10070, #24686, #46954, #46476 ),
 .UNSPECIFIED., .F., .F. ) 
 B_SPLINE_CURVE_WITH_KNOTS ( ( 3, 2, 2, 2, 3 ),
 ( 0.1150000000000000050, 0.1174999999999999933, 0.1199999999999999956, 0.1224999999999999978, 0.1250000000000000000 ),
 .UNSPECIFIED. ) 
 CURVE ( )  GEOMETRIC_REPRESENTATION_ITEM ( )  RATIONAL_B_SPLINE_CURVE ( ( 1.000000000000000000, 0.9238795325112869605, 1.000000000000000000, 0.9238795325112869605, 1.000000000000000000, 0.9238795325112869605, 1.000000000000000000, 0.9238795325112869605, 1.000000000000000000 ) ) 
 REPRESENTATION_ITEM ( '' )  ) ;
#30635=CARTESIAN_POINT ( 'NONE',  ( -0.07405724077823318263, -1.494094488135213394, 0.1787899950787401604 ) ) ;
#30641=CARTESIAN_POINT ( 'NONE',  ( -0.07405724077823318263, -0.5207932595678214094, 0.1787899950787401604 ) ) ;
#30642=CARTESIAN_POINT ( 'NONE',  ( -0.1639078578912291362, -0.08956131775089744285, -0.05627608123246346378 ) ) ;
#30650=FACE_OUTER_BOUND ( 'NONE', #32944, .T. ) ;
#30653=CARTESIAN_POINT ( 'NONE',  ( -0.1787899950787401882, -1.501476377898992354, 0.000000000000000000 ) ) ;
#30655=CARTESIAN_POINT ( 'NONE',  ( 0.1264236179284866091, -1.599901574749385880, 0.1264236179284866091 ) ) ;
#30664=CARTESIAN_POINT ( 'NONE',  ( -0.06523048226347956391, -0.4680118110236219930, -0.1574803149606300301 ) ) ;
#30676=CARTESIAN_POINT ( 'NONE',  ( -0.07117121207836790697, -0.08956324299011318713, 0.1404802767937309016 ) ) ;
#30677=CARTESIAN_POINT ( 'NONE',  ( 0.07405724077823318263, -0.4852362204186770889, -0.1787899950787401604 ) ) ;
#30684=CARTESIAN_POINT ( 'NONE',  ( 0.1787899950787401882, -1.752460629867496067, -2.189545951927503898E-17 ) ) ;
#30685=CARTESIAN_POINT ( 'NONE',  ( -0.1264236179284866091, -0.9552165353793071745, -0.1264236179284866091 ) ) ;
#30686=CARTESIAN_POINT ( 'NONE',  ( -0.06523048226347956391, -1.280019685039369470, 0.1574803149606297803 ) ) ;
#30689=ORIENTED_EDGE ( 'NONE', *, *, #15019, .F. ) ;
#30700=CARTESIAN_POINT ( 'NONE',  ( -0.2064293380533802347, 0.06762482675900732820, -0.1662510369723865233 ) ) ;
#30706=CARTESIAN_POINT ( 'NONE',  ( -0.2281650204108027769, -0.09842519685039370636, -0.09074154274604251391 ) ) ;
#30712=CARTESIAN_POINT ( 'NONE',  ( -0.1787899950787401604, -1.026574803095842370, -0.07405724077823318263 ) ) ;
#30715=CARTESIAN_POINT ( 'NONE',  ( -0.1797182628040039087, -0.3184493213940693401, -0.07444174185955065859 ) ) ;
#30716=CARTESIAN_POINT ( 'NONE',  ( 0.1574803149606299191, -1.769685039262551163, -1.928577636452523993E-17 ) ) ;
#30718=CARTESIAN_POINT ( 'NONE',  ( -0.1574803149606299191, 0.1692913385826771699, 0.000000000000000000 ) ) ;
#30720=CARTESIAN_POINT ( 'NONE',  ( 0.07405724077823318263, -0.1899606298674962612, 0.1787899950787401604 ) ) ;
#30730=DIRECTION ( 'NONE',  ( 1.000000000000000000, -0.000000000000000000, 1.224646799147353207E-16 ) ) ;
#30731=CARTESIAN_POINT ( 'NONE',  ( -0.07405724077823318263, -0.4064960629383624346, -0.1787899950787401604 ) ) ;
#30733=CARTESIAN_POINT ( 'NONE',  ( 0.1264236179284866091, -1.196358267662771757, -0.1264236179284866091 ) ) ;
#30742=CARTESIAN_POINT ( 'NONE',  ( 0.03732658744263399331, -0.09842026076056133166, -0.1748521113903349911 ) ) ;
#30751=VERTEX_POINT ( 'NONE', #47094 ) ;
#30766=CARTESIAN_POINT ( 'NONE',  ( 0.1264236179284866091, -1.566560976103254177, -0.1264236179284866091 ) ) ;
#30769=CARTESIAN_POINT ( 'NONE',  ( 0.07405724077823318263, -0.4064960629383624346, -0.1787899950787401604 ) ) ;
#30777=CARTESIAN_POINT ( 'NONE',  ( 0.1264236179284866091, -1.801673228292693052, 0.1264236179284866091 ) ) ;
#30782=CARTESIAN_POINT ( 'NONE',  ( 0.1574803149606300301, -0.7189960629921270385, 0.06523048226347956391 ) ) ;
#30784=CARTESIAN_POINT ( 'NONE',  ( -0.07444174185955065859, -1.647189478874384605, 0.1797182628040039087 ) ) ;
#30786=CARTESIAN_POINT ( 'NONE',  ( -0.1113553986120547346, -0.4557086613097952599, -0.1113553986120547346 ) ) ;
#30793=CARTESIAN_POINT ( 'NONE',  ( 0.000000000000000000, 0.1299212598425196763, 0.000000000000000000 ) ) ;
#30797=CARTESIAN_POINT ( 'NONE',  ( -1.094772975963752103E-17, 0.1028543307624250058, -0.1787899950787401882 ) ) ;
#30809=CARTESIAN_POINT ( 'NONE',  ( 0.000000000000000000, -0.09842519685039370636, 0.000000000000000000 ) ) ;
#30821=CARTESIAN_POINT ( 'NONE',  ( -0.1113553986120547346, 0.02657480325713335034, 0.1113553986120547346 ) ) ;
#30830=CARTESIAN_POINT ( 'NONE',  ( -0.07405724077823318263, -1.047368062717428217, -0.1787899950787401604 ) ) ;
#30832=CARTESIAN_POINT ( 'NONE',  ( -1.094772975963752103E-17, 0.1077755906049446960, -0.1787899950787401882 ) ) ;
#30841=CARTESIAN_POINT ( 'NONE',  ( 3.284318927891251994E-17, -0.6648622046706456068, 0.1787899950787401882 ) ) ;
#30844=CARTESIAN_POINT ( 'NONE',  ( 0.1797182628040039087, -1.086165856827139509, 0.07444174185955046430 ) ) ;
#30845=CARTESIAN_POINT ( 'NONE',  ( 0.1321676148590689159, 0.1299212598425196763, -0.1026092226670043267 ) ) ;
#30852=CARTESIAN_POINT ( 'NONE',  ( -0.1574803149606300301, -0.7288385825696378495, -0.06523048226347956391 ) ) ;
#30853=CARTESIAN_POINT ( 'NONE',  ( 0.07405724077823318263, 0.06594488194352732258, -0.1787899950787401604 ) ) ;
#30863=CARTESIAN_POINT ( 'NONE',  ( -9.642888182262618425E-18, -1.720472440837354400, -0.1574803149606299191 ) ) ;
#30867=CARTESIAN_POINT ( 'NONE',  ( 0.07051875723996789413, -0.08549467455831237517, 0.2447177463900755412 ) ) ;
#30868=CARTESIAN_POINT ( 'NONE',  ( -0.1264236179284866091, 0.1225393701325037388, 0.1264236179284866091 ) ) ;
#30874=CARTESIAN_POINT ( 'NONE',  ( -0.1574803149606299191, -0.3720472439869610404, 0.000000000000000000 ) ) ;
#30875=CARTESIAN_POINT ( 'NONE',  ( 0.07405724077823318263, -1.474409448765133801, -0.1787899950787401604 ) ) ;
#30877=VERTEX_POINT ( 'NONE', #32750 ) ;
#30883=CARTESIAN_POINT ( 'NONE',  ( -0.07405724077823318263, -0.4814231808276640545, 0.1787899950787401604 ) ) ;
#30884=CARTESIAN_POINT ( 'NONE',  ( 0.2001661423152484298, -0.08956032108766456834, 0.05039172328576543847 ) ) ;
#30890=CARTESIAN_POINT ( 'NONE',  ( -0.1787899950787401882, -1.827387747756799241, 0.000000000000000000 ) ) ;
#30892=CARTESIAN_POINT ( 'NONE',  ( 0.2471922732848571835, -0.07885118474260616184, 0.07559718168574836028 ) ) ;
#30896=CARTESIAN_POINT ( 'NONE',  ( -0.1787899950787401882, -1.422736220418677311, 0.000000000000000000 ) ) ;
#30900=CARTESIAN_POINT ( 'NONE',  ( -0.1270800023317771588, -0.7539808174570609145, -0.1270800023317771588 ) ) ;
#30914=CARTESIAN_POINT ( 'NONE',  ( 0.1787899950787401882, -0.5319881889226142357, -2.189545951927503898E-17 ) ) ;
#30920=CARTESIAN_POINT ( 'NONE',  ( -0.07405724077823318263, -1.779527559001355952, -0.1787899950787401604 ) ) ;
#30921=CARTESIAN_POINT ( 'NONE',  ( 0.1787899950787401604, -0.8887795275052913224, -0.07405724077823318263 ) ) ;
#30922=CARTESIAN_POINT ( 'NONE',  ( -0.1574803149606299191, -1.405511811023622215, 0.000000000000000000 ) ) ;
#30933=FACE_OUTER_BOUND ( 'NONE', #14928, .T. ) ;
#30938=DIRECTION ( 'NONE',  ( 0.000000000000000000, -1.000000000000000000, 0.000000000000000000 ) ) ;
#30944=CARTESIAN_POINT ( 'NONE',  ( -0.02314857569221047059, -0.09842519685039370636, 0.2241248956163086614 ) ) ;
#30950=CARTESIAN_POINT ( 'NONE',  ( -0.1787899950787401882, -1.029035433017102319, 0.000000000000000000 ) ) ;
#30951=CARTESIAN_POINT ( 'NONE',  ( 0.07405724077823318263, -1.169291338528914537, 0.1787899950787401604 ) ) ;
#30953=CARTESIAN_POINT ( 'NONE',  ( 3.301370929368692659E-17, -0.3061461717877700939, 0.1797182628040039365 ) ) ;
#30954=CARTESIAN_POINT ( 'NONE',  ( -0.1113553986120547346, -0.03248031496062991907, -0.1113553986120547346 ) ) ;
#30962=CARTESIAN_POINT ( 'NONE',  ( 0.1264236179284866091, -0.4926181101824567143, -0.1264236179284866091 ) ) ;
#30964=CARTESIAN_POINT ( 'NONE',  ( 0.1264236179284866091, -1.324311023568283341, 0.1264236179284866091 ) ) ;
#30978=CARTESIAN_POINT ( 'NONE',  ( -0.08774906724784053980, -0.09246610911299792124, 0.2347711071351809009 ) ) ;
#30984=CARTESIAN_POINT ( 'NONE',  ( -0.2415982954816964789, -0.09851385206391319316, -0.02995337850299783361 ) ) ;
#30992=CARTESIAN_POINT ( 'NONE',  ( 0.1787899950787401604, -1.652683023347347957, 0.07405724077823318263 ) ) ;
#30995=CARTESIAN_POINT ( 'NONE',  ( -0.07405724077823318263, -0.5196850393163150450, -0.1787899950787401604 ) ) ;
#31001=CARTESIAN_POINT ( 'NONE',  ( 0.1787899950787401604, -1.799212598371432659, 0.07405724077823318263 ) ) ;
#31006=CARTESIAN_POINT ( 'NONE',  ( -9.642888182262618425E-18, -0.7460629921259843700, -0.1574803149606299191 ) ) ;
#31008=CARTESIAN_POINT ( 'NONE',  ( 0.07444174185955065859, -1.524157982811393586, 0.1797182628040039087 ) ) ;
#31010=CARTESIAN_POINT ( 'NONE',  ( -0.1113553986120547346, -0.06200787390822106587, -0.1113553986120547346 ) ) ;
#31011=CARTESIAN_POINT ( 'NONE',  ( 2.892866454678787531E-17, -0.4803149605223936969, 0.1574803149606299191 ) ) ;
#31013=CARTESIAN_POINT ( 'NONE',  ( 0.1264236179284866091, -0.4187992125446614589, 0.1264236179284866091 ) ) ;
#31014=CARTESIAN_POINT ( 'NONE',  ( 0.2471922904502827090, 0.07573437638785612824, -0.08155181604444516896 ) ) ;
#31025=CARTESIAN_POINT ( 'NONE',  ( -0.1787899950787401604, 0.1102362205262043815, -0.07405724077823318263 ) ) ;
#31036=CARTESIAN_POINT ( 'NONE',  ( 3.284318927891251994E-17, -1.334153543253322916, 0.1787899950787401882 ) ) ;
#31048=CARTESIAN_POINT ( 'NONE',  ( -0.1264236179284866091, 0.07824803154982658271, 0.1264236179284866091 ) ) ;
#31053=CARTESIAN_POINT ( 'NONE',  ( 0.1113553986120547346, -0.1505905510735753849, -0.1113553986120547346 ) ) ;
#31060=CARTESIAN_POINT ( 'NONE',  ( 0.1264236179284866091, -1.094120031221364142, -0.1264236179284866091 ) ) ;
#31062=CARTESIAN_POINT ( 'NONE',  ( -0.1787899950787401882, -0.03986220467064590517, 0.000000000000000000 ) ) ;
#31069=CARTESIAN_POINT ( 'NONE',  ( -0.07405724077823318263, -0.5639763778989922427, -0.1787899950787401604 ) ) ;
#31073=CARTESIAN_POINT ( 'NONE',  ( 0.07444174185955065859, -1.209197352890132970, 0.1797182628040039087 ) ) ;
#31083=CARTESIAN_POINT ( 'NONE',  ( -0.1787899950787401604, 0.1200787402112438867, 0.07405724077823318263 ) ) ;
#31094=CARTESIAN_POINT ( 'NONE',  ( 0.06523048226347956391, -1.619586614065700036, 0.1574803149606297803 ) ) ;
#31098=CARTESIAN_POINT ( 'NONE',  ( 0.08995663987707425147, -0.09317336072452189755, 0.2334965874938940145 ) ) ;
#31099=CARTESIAN_POINT ( 'NONE',  ( 0.1264236179284866091, 0.1323818898175431191, 0.1264236179284866091 ) ) ;
#31104=CARTESIAN_POINT ( 'NONE',  ( -0.1264236179284866091, -1.496555118056472677, 0.1264236179284866091 ) ) ;
#31109=VERTEX_POINT ( 'NONE', #40912 ) ;
#31111=CARTESIAN_POINT ( 'NONE',  ( 0.1264236179284866091, -0.7397893225599468936, -0.1264236179284866091 ) ) ;
#31113=CARTESIAN_POINT ( 'NONE',  ( 0.1731537741114069218, -0.08956052929350570568, -0.09650519479221614239 ) ) ;
#31123=CARTESIAN_POINT ( 'NONE',  ( -1.094772975963752103E-17, -1.511318897584031484, -0.1787899950787401882 ) ) ;
#31127=CARTESIAN_POINT ( 'NONE',  ( -0.1797182628040039365, -0.7096894788743838278, 0.000000000000000000 ) ) ;
#31130=CARTESIAN_POINT ( 'NONE',  ( -0.1113553986120547346, -0.4163385826771653364, 0.1113553986120547346 ) ) ;
#31140=CARTESIAN_POINT ( 'NONE',  ( -0.06523048226347956391, -0.5762795274515275512, -0.1574803149606300301 ) ) ;
#31144=CARTESIAN_POINT ( 'NONE',  ( -0.07405724077823318263, -0.5984251967966303098, -0.1787899950787401604 ) ) ;
#31151=CARTESIAN_POINT ( 'NONE',  ( 0.07405724077823318263, -1.784448818843874962, -0.1787899950787401604 ) ) ;
#31152=CARTESIAN_POINT ( 'NONE',  ( 0.07405724077823318263, -0.8986220471903317852, 0.1787899950787401604 ) ) ;
#31153=CARTESIAN_POINT ( 'NONE',  ( 0.06523048226347956391, -1.314468503937008093, 0.1574803149606297803 ) ) ;
#31160=ORIENTED_EDGE ( 'NONE', *, *, #19593, .F. ) ;
#31161=CARTESIAN_POINT ( 'NONE',  ( 0.1574803149606299191, -1.375984251860976393, -1.928577636452523993E-17 ) ) ;
#31170=CARTESIAN_POINT ( 'NONE',  ( 0.04509681258129913384, -0.07057211410339600532, -0.2593943580756443157 ) ) ;
#31174=CARTESIAN_POINT ( 'NONE',  ( 0.1642845807979765871, -0.09842519685039370636, -0.1153058249971240234 ) ) ;
#31179=CARTESIAN_POINT ( 'NONE',  ( 0.1787899950787401882, -1.088090551127338657, -2.189545951927503898E-17 ) ) ;
#31180=CARTESIAN_POINT ( 'NONE',  ( 0.1264236179284866091, -1.275098425143086578, -0.1264236179284866091 ) ) ;
#31182=CARTESIAN_POINT ( 'NONE',  ( 0.1797182628040039087, -0.4562445969846198879, 0.07444174185955046430 ) ) ;
#31185=CARTESIAN_POINT ( 'NONE',  ( 0.06523048226347956391, -0.0004921259842519828086, -0.1574803149606300301 ) ) ;
#31186=CARTESIAN_POINT ( 'NONE',  ( -0.1264236179284866091, -0.1579724408911182820, 0.1264236179284866091 ) ) ;
#31195=CARTESIAN_POINT ( 'NONE',  ( 0.1264236179284866091, -0.5024606298674960669, 0.1264236179284866091 ) ) ;
#31197=CARTESIAN_POINT ( 'NONE',  ( -0.07405724077823318263, -1.410433070812377565, 0.1787899950787401604 ) ) ;
#31207=CARTESIAN_POINT ( 'NONE',  ( 2.892866454678787531E-17, -1.228346456585385882, 0.1574803149606299191 ) ) ;
#31210=CARTESIAN_POINT ( 'NONE',  ( 0.09469176317940933285, -0.09842519655130997636, -0.1516944367183098441 ) ) ;
#31213=CARTESIAN_POINT ( 'NONE',  ( 0.1574803149606299191, -0.08661417322834646937, -1.928577636452523993E-17 ) ) ;
#31217=CARTESIAN_POINT ( 'NONE',  ( 0.1467038341990881956, -0.09851384883411416771, 0.1600693656517706842 ) ) ;
#31222=CARTESIAN_POINT ( 'NONE',  ( -0.07405724077823318263, -1.544415306811916633, 0.1787899950787401604 ) ) ;
#31225=CARTESIAN_POINT ( 'NONE',  ( -0.1787899950787401604, -0.5541338582139530011, -0.07405724077823318263 ) ) ;
#31228=LINE ( 'NONE', #45337, #368 ) ;
#31229=CARTESIAN_POINT ( 'NONE',  ( 0.1787899950787401882, -0.2219488188438744347, -2.189545951927503898E-17 ) ) ;
#31230=CARTESIAN_POINT ( 'NONE',  ( -0.1787899950787401604, -0.8297244093950564281, -0.07405724077823318263 ) ) ;
#31235=CARTESIAN_POINT ( 'NONE',  ( 0.07405724077823318263, -0.004060976103254483952, 0.1787899950787401604 ) ) ;
#31236=CARTESIAN_POINT ( 'NONE',  ( 0.1264236179284866091, -1.757381889710015965, 0.1264236179284866091 ) ) ;
#31242=CARTESIAN_POINT ( 'NONE',  ( 0.1113553986120547346, -0.9576771653543306728, 0.1113553986120547346 ) ) ;
#31244=CARTESIAN_POINT ( 'NONE',  ( -0.1797182628040039365, -1.615201289898005710, 0.000000000000000000 ) ) ;
#31246=CARTESIAN_POINT ( 'NONE',  ( -0.06523048226347956391, -0.4434055117034965132, 0.1574803149606297803 ) ) ;
#31254=CARTESIAN_POINT ( 'NONE',  ( 0.06523048226347956391, -0.8567913384751505435, -0.1574803149606300301 ) ) ;
#31255=CARTESIAN_POINT ( 'NONE',  ( -0.1787899950787401604, 0.07578740162856664742, 0.07405724077823318263 ) ) ;
#31266=ORIENTED_EDGE ( 'NONE', *, *, #9215, .T. ) ;
#31267=CARTESIAN_POINT ( 'NONE',  ( -0.1264236179284866091, -1.299704724355684959, 0.1264236179284866091 ) ) ;
#31277=EDGE_LOOP ( 'NONE', ( #46675, #45714, #14633, #31160, #36500 ) ) ;
#31282=CARTESIAN_POINT ( 'NONE',  ( -9.642888182262618425E-18, -0.2244094487113704739, -0.1574803149606299191 ) ) ;
#31287=CARTESIAN_POINT ( 'NONE',  ( 0.1264236179284866091, -1.182702708386718538, 0.1264236179284866091 ) ) ;
#31289=CARTESIAN_POINT ( 'NONE',  ( -0.1787899950787401882, -0.07923228341080354453, 0.000000000000000000 ) ) ;
#31293=DIRECTION ( 'NONE',  ( 0.000000000000000000, -1.000000000000000000, 0.000000000000000000 ) ) ;
#31297=CARTESIAN_POINT ( 'NONE',  ( 0.1787899950787401604, -0.6525590550643474153, -0.07405724077823318263 ) ) ;
#31301=CARTESIAN_POINT ( 'NONE',  ( 0.07444174185955046430, -1.194433573362573497, -0.1797182628040039087 ) ) ;
#31312=CARTESIAN_POINT ( 'NONE',  ( 0.06523048226347956391, -0.7534448817822362310, 0.1574803149606297803 ) ) ;
#31313=CARTESIAN_POINT ( 'NONE',  ( 0.06841996760812382727, 0.1299212598425196763, 0.1651804176431311000 ) ) ;
#31321=CARTESIAN_POINT ( 'NONE',  ( 2.892866454678787531E-17, -1.700787401467275473, 0.1574803149606299191 ) ) ;
#31326=CARTESIAN_POINT ( 'NONE',  ( 0.1264236179284866091, 0.06348425202226751218, -0.1264236179284866091 ) ) ;
#31330=CARTESIAN_POINT ( 'NONE',  ( -0.07034821948466075947, 0.08559642391438677944, 0.2448175074096620163 ) ) ;
#31331=CARTESIAN_POINT ( 'NONE',  ( -1.094772975963752103E-17, -1.708169291284818980, -0.1787899950787401882 ) ) ;
#31338=CARTESIAN_POINT ( 'NONE',  ( -1.094772975963752103E-17, -0.6954979839772696959, -0.1787899950787401882 ) ) ;
#31340=CARTESIAN_POINT ( 'NONE',  ( 0.1797904941528189193, -0.08956025049567893637, 0.1078749962962417402 ) ) ;
#31349=EDGE_CURVE ( 'NONE', #26985, #39269, #2369, .T. ) ;
#31354=ORIENTED_EDGE ( 'NONE', *, *, #44041, .T. ) ;
#31361=CARTESIAN_POINT ( 'NONE',  ( -0.07444174185955065859, -0.6629375103704481242, 0.1797182628040039087 ) ) ;
#31362=CARTESIAN_POINT ( 'NONE',  ( 0.2471922904502827090, 0.09773636000336977103, 0.01649811039745145355 ) ) ;
#31365=CARTESIAN_POINT ( 'NONE',  ( -0.1574803149606297803, -0.4187992125984250080, 0.06523048226347956391 ) ) ;
#31366=CARTESIAN_POINT ( 'NONE',  ( -0.03598878106637547203, -0.09842522444525984848, 0.1542999736886214723 ) ) ;
#31372=CARTESIAN_POINT ( 'NONE',  ( 0.1113553986120547346, 0.08562992136736949367, -0.1113553986120547346 ) ) ;
#31374=FACE_OUTER_BOUND ( 'NONE', #34679, .T. ) ;
#31377=CARTESIAN_POINT ( 'NONE',  ( -0.06523048226347956391, -0.6008858266641260437, 0.1574803149606297803 ) ) ;
#31381=CARTESIAN_POINT ( 'NONE',  ( -0.1659561666016914627, -0.08956010649363622955, -0.04686757988705942540 ) ) ;
#31382=CARTESIAN_POINT ( 'NONE',  ( 0.1264236179284866091, -0.4876968503399370380, -0.1264236179284866091 ) ) ;
#31385=CARTESIAN_POINT ( 'NONE',  ( 0.06841996760812382727, 0.1299212598425196763, 0.1651804176431311000 ) ) ;
#31388=ORIENTED_EDGE ( 'NONE', *, *, #45584, .T. ) ;
#31391=CARTESIAN_POINT ( 'NONE',  ( 0.1787899950787401604, -1.710629921206078041, -0.07405724077823318263 ) ) ;
#31392=CARTESIAN_POINT ( 'NONE',  ( 0.1787899950787401882, -1.048720472387181024, -2.189545951927503898E-17 ) ) ;
#31393=CARTESIAN_POINT ( 'NONE',  ( -0.06523048226347956391, -1.373523622047243320, -0.1574803149606300301 ) ) ;
#31406=CARTESIAN_POINT ( 'NONE',  ( 0.04858533447342753414, -0.07294156354243669371, -0.2573812140284293393 ) ) ;
#31409=CARTESIAN_POINT ( 'NONE',  ( 0.1787899950787401604, -0.2747302674418372059, 0.07405724077823318263 ) ) ;
#31411=CARTESIAN_POINT ( 'NONE',  ( -0.04012737397972362258, -0.09842519685039370636, -0.1835268552075023374 ) ) ;
#31418=CARTESIAN_POINT ( 'NONE',  ( -0.07405724077823318263, -0.9822834645131651721, 0.1787899950787401604 ) ) ;
#31419=CARTESIAN_POINT ( 'NONE',  ( 0.07405724077823318263, -1.208661417269070393, 0.1787899950787401604 ) ) ;
#31421=CARTESIAN_POINT ( 'NONE',  ( -0.07444174185955065859, -0.4660871166696600731, 0.1797182628040039087 ) ) ;
#31425=CARTESIAN_POINT ( 'NONE',  ( 0.06523048226347956391, -0.01525590551181101734, 0.1574803149606297803 ) ) ;
#31431=CARTESIAN_POINT ( 'NONE',  ( -1.094772975963752103E-17, -0.6451771653005667906, -0.1787899950787401882 ) ) ;
#31433=CARTESIAN_POINT ( 'NONE',  ( 0.1264236179284866091, -1.314468503883243988, -0.1264236179284866091 ) ) ;
#31438=LINE ( 'NONE', #35501, #2968 ) ;
#31441=CARTESIAN_POINT ( 'NONE',  ( 0.1697303854094444342, -0.09842519689050829856, -0.05760433632937374260 ) ) ;
#31446=CARTESIAN_POINT ( 'NONE',  ( 0.06523048226347956391, -0.07923228346456692717, -0.1574803149606300301 ) ) ;
#31450=CARTESIAN_POINT ( 'NONE',  ( 0.2014638753618972489, -0.09851384545634704615, 0.06137933528758169471 ) ) ;
#31454=ADVANCED_FACE ( 'NONE', ( #10860 ), #6, .T. ) ;
#31456=CARTESIAN_POINT ( 'NONE',  ( -0.1264236179284866091, -1.546875936733175250, 0.1264236179284866091 ) ) ;
#31459=CARTESIAN_POINT ( 'NONE',  ( -0.07405724077823318263, -0.6230314960092281362, 0.1787899950787401604 ) ) ;
#31465=CARTESIAN_POINT ( 'NONE',  ( -1.094772975963752103E-17, -0.2908464566391499861, -0.1787899950787401882 ) ) ;
#31466=CARTESIAN_POINT ( 'NONE',  ( -0.07405724077823318263, -0.7805118109698575557, 0.1787899950787401604 ) ) ;
#31469=CARTESIAN_POINT ( 'NONE',  ( -0.07405724077823318263, 0.06975792153454075939, 0.1787899950787401604 ) ) ;
#31475=CARTESIAN_POINT ( 'NONE',  ( 0.1113553986120547346, -0.9084645669291337988, -0.1113553986120547346 ) ) ;
#31477=CARTESIAN_POINT ( 'NONE',  ( -0.1797182628040039087, -1.538921762338951060, -0.07444174185955065859 ) ) ;
#31488=CARTESIAN_POINT ( 'NONE',  ( -0.07405724077823318263, 0.08070866147108628208, 0.1787899950787401604 ) ) ;
#31490=CARTESIAN_POINT ( 'NONE',  ( 0.1787899950787401604, -0.05708661411946481384, -0.07405724077823318263 ) ) ;
#31493=CARTESIAN_POINT ( 'NONE',  ( -0.1264236179284866091, -0.9404527558517480346, 0.1264236179284866091 ) ) ;
#31499=DIRECTION ( 'NONE',  ( -0.000000000000000000, -1.000000000000000000, -0.000000000000000000 ) ) ;
#31514=CARTESIAN_POINT ( 'NONE',  ( -0.07405724077823318263, 0.08070866147108628208, 0.1787899950787401604 ) ) ;
#31523=CARTESIAN_POINT ( 'NONE',  ( -0.1787899950787401604, -1.121186960355223139, -0.07405724077823318263 ) ) ;
#31525=CARTESIAN_POINT ( 'NONE',  ( 0.1787899950787401882, -0.1382874015210395768, -2.189545951927503898E-17 ) ) ;
#31532=EDGE_CURVE ( 'NONE', #27412, #34797, #5267, .T. ) ;
#31536=CARTESIAN_POINT ( 'NONE',  ( -0.1264236179284866091, -0.6796259841982046357, -0.1264236179284866091 ) ) ;
#31539=CARTESIAN_POINT ( 'NONE',  ( 0.1797182628040039365, -1.083705226905880004, -2.200913952912460540E-17 ) ) ;
#31550=CARTESIAN_POINT ( 'NONE',  ( -0.06523048226347956391, -0.7189960628845993851, 0.1574803149606297803 ) ) ;
#31551=CARTESIAN_POINT ( 'NONE',  ( -0.1787899950787401604, 0.04133858273092887170, 0.07405724077823318263 ) ) ;
#31565=CARTESIAN_POINT ( 'NONE',  ( 0.1264236179284866091, 0.1422244095025824717, -0.1264236179284866091 ) ) ;
#31573=CARTESIAN_POINT ( 'NONE',  ( 0.1787899950787401604, -1.715551181048599716, -0.07405724077823318263 ) ) ;
#31580=CARTESIAN_POINT ( 'NONE',  ( 3.284318927891251994E-17, -0.6758129446071911017, 0.1787899950787401882 ) ) ;
#31582=CARTESIAN_POINT ( 'NONE',  ( 0.1289854442636478304, -0.08956037640241240605, -0.1454962696668769817 ) ) ;
#31599=CARTESIAN_POINT ( 'NONE',  ( -0.1574803149606297803, -0.4975393700787406059, 0.06523048226347956391 ) ) ;
#31613=CARTESIAN_POINT ( 'NONE',  ( 0.1787899950787401604, -0.5688976377415115859, -0.07405724077823318263 ) ) ;
#31615=CONICAL_SURFACE ( 'NONE', #14007, 0.2471922904502826812, 0.5235987755982992597 ) ;
#31619=CARTESIAN_POINT ( 'NONE',  ( -0.05837987205261271212, 0.07899857248962625922, -0.2517274360213099804 ) ) ;
#31621=CARTESIAN_POINT ( 'NONE',  ( -0.07444174185955065859, 0.1097002849051434414, -0.1797182628040039087 ) ) ;
#31622=CARTESIAN_POINT ( 'NONE',  ( -1.094772975963752103E-17, -1.078248031442299304, -0.1787899950787401882 ) ) ;
#31623=CARTESIAN_POINT ( 'NONE',  ( 0.1113553986120547346, -1.351377952755905554, 0.1113553986120547346 ) ) ;
#31632=CARTESIAN_POINT ( 'NONE',  ( -0.1113553986120547346, -1.430118110128692832, 0.1113553986120547346 ) ) ;
#31640=CARTESIAN_POINT ( 'NONE',  ( -0.1378230750848668529, 0.09774221684002683264, 0.2058608813653518832 ) ) ;
#31643=CARTESIAN_POINT ( 'NONE',  ( -0.1787899950787401604, -0.2894940469693961238, 0.07405724077823318263 ) ) ;
#31644=CARTESIAN_POINT ( 'NONE',  ( 0.1954512992741562760, -0.09842519685039370636, 0.08123841634054980443 ) ) ;
#31645=CARTESIAN_POINT ( 'NONE',  ( -0.1574803149606299191, 0.01181102362204724393, 0.000000000000000000 ) ) ;
#31649=AXIS2_PLACEMENT_3D ( 'NONE', #30809, #2012, #27693 ) ;
#31650=ORIENTED_EDGE ( 'NONE', *, *, #6862, .F. ) ;
#31652=CARTESIAN_POINT ( 'NONE',  ( -0.07405724077823318263, -1.061023621993481214, 0.1787899950787401604 ) ) ;
#31653=CARTESIAN_POINT ( 'NONE',  ( 0.1787899950787401882, -1.201279527505291433, -2.189545951927503898E-17 ) ) ;
#31655=CARTESIAN_POINT ( 'NONE',  ( 0.07444174185955065859, -0.5399060143074553286, 0.1797182628040039087 ) ) ;
#31659=CARTESIAN_POINT ( 'NONE',  ( 2.892866454678787531E-17, 0.02165354330708661734, 0.1574803149606299191 ) ) ;
#31665=ORIENTED_EDGE ( 'NONE', *, *, #42772, .T. ) ;
#31666=ORIENTED_EDGE ( 'NONE', *, *, #14771, .T. ) ;
#31669=CARTESIAN_POINT ( 'NONE',  ( -0.1787899950787401604, -0.5541338582139530011, 0.07405724077823318263 ) ) ;
#31670=CARTESIAN_POINT ( 'NONE',  ( -0.1787899950787401604, -1.341535433017102541, -0.07405724077823318263 ) ) ;
#31682=CARTESIAN_POINT ( 'NONE',  ( 0.1781957201322358353, -0.09842519685039370636, -0.01456528979491370120 ) ) ;
#31687=ORIENTED_EDGE ( 'NONE', *, *, #3121, .T. ) ;
#31693=CARTESIAN_POINT ( 'NONE',  ( 0.03861100025345957226, -0.09851384863655454627, 0.2192374635482165490 ) ) ;
#31694=ORIENTED_EDGE ( 'NONE', *, *, #25596, .F. ) ;
#31698=CARTESIAN_POINT ( 'NONE',  ( -0.1787899950787401604, -0.5885826771115909573, 0.07405724077823318263 ) ) ;
#31702=CARTESIAN_POINT ( 'NONE',  ( -0.1787899950787401604, -0.7903543306548983516, -0.07405724077823318263 ) ) ;
#31706=CARTESIAN_POINT ( 'NONE',  ( -0.1787899950787401604, -0.01390349578829383655, 0.07405724077823318263 ) ) ;
#31707=CARTESIAN_POINT ( 'NONE',  ( -1.094772975963752103E-17, 0.02411417328210995956, -0.1787899950787401882 ) ) ;
#31709=CARTESIAN_POINT ( 'NONE',  ( 0.08053768427153103204, -0.09842519685039369248, 0.1460475935136278658 ) ) ;
#31713=CARTESIAN_POINT ( 'NONE',  ( 0.06523048226347956391, -0.9453740157480327033, -0.1574803149606300301 ) ) ;
#31715=CARTESIAN_POINT ( 'NONE',  ( 0.07444174185955065859, -1.799748533992495014, 0.1797182628040039087 ) ) ;
#31724=CARTESIAN_POINT ( 'NONE',  ( -0.1787899950787401604, -0.1210629920722208208, 0.07405724077823318263 ) ) ;
#31726=CARTESIAN_POINT ( 'NONE',  ( 0.1787899950787401882, -0.9256889763241890057, -2.189545951927503898E-17 ) ) ;
#31736=CARTESIAN_POINT ( 'NONE',  ( -9.642888182262618425E-18, -1.090551180994834723, -0.1574803149606299191 ) ) ;
#31748=CARTESIAN_POINT ( 'NONE',  ( -0.1787899950787401604, 0.1102362205262043815, -0.07405724077823318263 ) ) ;
#31756=CARTESIAN_POINT ( 'NONE',  ( -1.094772975963752103E-17, -1.128568850119001876, -0.1787899950787401882 ) ) ;
#31757=ORIENTED_EDGE ( 'NONE', *, *, #35766, .F. ) ;
#31758=CARTESIAN_POINT ( 'NONE',  ( 3.284318927891251994E-17, -0.1874999999462366451, 0.1787899950787401882 ) ) ;
#31767=CARTESIAN_POINT ( 'NONE',  ( -0.1797182628040039365, -0.1585083765121793331, 0.000000000000000000 ) ) ;
#31768=CARTESIAN_POINT ( 'NONE',  ( -0.1264236179284866091, -0.7189960629383621571, -0.1264236179284866091 ) ) ;
#31772=CARTESIAN_POINT ( 'NONE',  ( -0.07444174185955065859, -1.174748533992494126, 0.1797182628040039087 ) ) ;
#31799=CARTESIAN_POINT ( 'NONE',  ( 3.284318927891251994E-17, 0.04872047249470835839, 0.1787899950787401882 ) ) ;
#31806=CARTESIAN_POINT ( 'NONE',  ( 0.1264236179284866091, -1.673720472387181024, -0.1264236179284866091 ) ) ;
#31819=CARTESIAN_POINT ( 'NONE',  ( 2.892866454678787531E-17, -0.01771653543307086590, 0.1574803149606299191 ) ) ;
#31824=CARTESIAN_POINT ( 'NONE',  ( 0.1797182628040039365, -0.6900044395043051226, -2.200913952912460540E-17 ) ) ;
#31825=CARTESIAN_POINT ( 'NONE',  ( 0.2471922904502826812, 0.09442133267706716293, 0.03395025085954773980 ) ) ;
#31829=CARTESIAN_POINT ( 'NONE',  ( 0.06523048226347956391, -0.6304133858267716439, -0.1574803149606300301 ) ) ;
#31840=CARTESIAN_POINT ( 'NONE',  ( 0.1574803149606299191, -0.5885826770578268530, -1.928577636452523993E-17 ) ) ;
#31846=CARTESIAN_POINT ( 'NONE',  ( -0.1158283541424031532, -0.08956345598586890056, -0.1361971163587911426 ) ) ;
#31854=CARTESIAN_POINT ( 'NONE',  ( -0.1264236179284866091, -1.806594488135212728, 0.1264236179284866091 ) ) ;
#31855=CARTESIAN_POINT ( 'NONE',  ( 0.1787899950787401604, -1.051181102308440529, 0.07405724077823318263 ) ) ;
#31856=CARTESIAN_POINT ( 'NONE',  ( 0.1574803149606300301, -1.462106299212597493, -0.06523048226347956391 ) ) ;
#31868=CARTESIAN_POINT ( 'NONE',  ( -0.1235961452251413406, 0.09842519685039370636, -0.2140748031496062798 ) ) ;
#31873=CARTESIAN_POINT ( 'NONE',  ( 0.1264236179284866091, -0.1984507398827823066, 0.1264236179284866091 ) ) ;
#31874=CARTESIAN_POINT ( 'NONE',  ( 0.1267115641817155580, -0.09842519685039370636, 0.1767117842128110017 ) ) ;
#31885=CARTESIAN_POINT ( 'NONE',  ( -0.1264236179284866091, -1.191437007820251859, -0.1264236179284866091 ) ) ;
#31886=CARTESIAN_POINT ( 'NONE',  ( -0.07405724077823318263, -1.292322834591905778, 0.1787899950787401604 ) ) ;
#31887=CARTESIAN_POINT ( 'NONE',  ( -0.1270800023317771588, -0.5571304237562740846, -0.1270800023317771588 ) ) ;
#31891=CARTESIAN_POINT ( 'NONE',  ( 0.1113553986120547346, -0.1309055118110236116, 0.1113553986120547346 ) ) ;
#31903=CARTESIAN_POINT ( 'NONE',  ( 0.07405724077823318263, -0.6082677164816695514, -0.1787899950787401604 ) ) ;
#31904=CARTESIAN_POINT ( 'NONE',  ( -0.1787899950787401604, -1.415354330654897019, 0.07405724077823318263 ) ) ;
#31923=CARTESIAN_POINT ( 'NONE',  ( 0.08749754606363346898, -0.09851384719155904801, 0.2018685754223755735 ) ) ;
#31927=CARTESIAN_POINT ( 'NONE',  ( -0.07405724077823318263, -0.5984251967966303098, -0.1787899950787401604 ) ) ;
#31938=CARTESIAN_POINT ( 'NONE',  ( -1.094772975963752103E-17, 0.01316343334556440911, -0.1787899950787401882 ) ) ;
#31946=CARTESIAN_POINT ( 'NONE',  ( 0.1574803149606300301, -0.8371062992125989366, 0.06523048226347956391 ) ) ;
#31948=CARTESIAN_POINT ( 'NONE',  ( -0.07444174185955065859, -1.686559557614542459, 0.1797182628040039087 ) ) ;
#31950=CARTESIAN_POINT ( 'NONE',  ( 0.1574803149606300301, -0.5073818896562523051, -0.06523048226347956391 ) ) ;
#31951=CARTESIAN_POINT ( 'NONE',  ( -0.1787899950787401882, -0.3941929133320630219, 0.000000000000000000 ) ) ;
#31957=CARTESIAN_POINT ( 'NONE',  ( -0.1916485431826253083, -0.07731288306168948576, -0.1747847109491778572 ) ) ;
#31959=CARTESIAN_POINT ( 'NONE',  ( 0.1787899950787401882, -0.1038385826234017734, -2.189545951927503898E-17 ) ) ;
#31960=CARTESIAN_POINT ( 'NONE',  ( 0.1787899950787401604, -0.9232283464029299447, -0.07405724077823318263 ) ) ;
#31974=CARTESIAN_POINT ( 'NONE',  ( 0.000000000000000000, 0.1102362204724409434, 0.000000000000000000 ) ) ;
#31977=CARTESIAN_POINT ( 'NONE',  ( 0.07405724077823318263, 0.1250000000537635492, 0.1787899950787401604 ) ) ;
#31984=CARTESIAN_POINT ( 'NONE',  ( 0.000000000000000000, -0.09842519685039370636, 0.2471922904502826812 ) ) ;
#31985=CARTESIAN_POINT ( 'NONE',  ( 3.284318927891251994E-17, -1.069513732008765761, 0.1787899950787401882 ) ) ;
#31987=CARTESIAN_POINT ( 'NONE',  ( 0.1264236179284866091, -0.06446850388324429360, 0.1264236179284866091 ) ) ;
#31994=CARTESIAN_POINT ( 'NONE',  ( 0.07405724077823318263, -1.474409448765133801, -0.1787899950787401604 ) ) ;
#32004=CARTESIAN_POINT ( 'NONE',  ( 0.1113553986120547346, -0.7903543306011338032, 0.1113553986120547346 ) ) ;
#32007=CARTESIAN_POINT ( 'NONE',  ( 0.1787899950787401604, 0.01673228351833044164, 0.07405724077823318263 ) ) ;
#32023=CARTESIAN_POINT ( 'NONE',  ( 3.284318927891251994E-17, 0.009350393754550925460, 0.1787899950787401882 ) ) ;
#32028=CARTESIAN_POINT ( 'NONE',  ( 0.1588215770322271292, 0.09266989036297287874, 0.1937373906134645662 ) ) ;
#32032=CARTESIAN_POINT ( 'NONE',  ( 0.1574803149606299191, -0.3917322833570398011, -1.928577636452523993E-17 ) ) ;
#32033=CARTESIAN_POINT ( 'NONE',  ( 0.1264236179284866091, -1.683562992072220599, 0.1264236179284866091 ) ) ;
#32040=CARTESIAN_POINT ( 'NONE',  ( -0.1787899950787401604, -0.7225649131111276935, 0.07405724077823318263 ) ) ;
#32042=CARTESIAN_POINT ( 'NONE',  ( -0.1113553986120547346, -0.02263779516806350284, -0.1113553986120547346 ) ) ;
#32049=CARTESIAN_POINT ( 'NONE',  ( -9.642888182262618425E-18, 0.08070866141732284393, -0.1574803149606299191 ) ) ;
#32052=DIRECTION ( 'NONE',  ( 0.000000000000000000, 0.000000000000000000, 1.000000000000000000 ) ) ;
#32057=CARTESIAN_POINT ( 'NONE',  ( 0.1797182628040039365, -0.8081146757247775758, -2.200913952912460540E-17 ) ) ;
#32058=CARTESIAN_POINT ( 'NONE',  ( 0.2471922904502827090, 0.08082342248660308315, 0.07163232281567669113 ) ) ;
#32061=CARTESIAN_POINT ( 'NONE',  ( 0.1574803149606299191, -0.5196850393700787052, -1.928577636452523993E-17 ) ) ;
#32071=CARTESIAN_POINT ( 'NONE',  ( 0.07405724077823318263, -0.6427165353793066194, -0.1787899950787401604 ) ) ;
#32079=CARTESIAN_POINT ( 'NONE',  ( -0.1797182628040039087, 0.08017272585002534202, 0.07444174185955065859 ) ) ;
#32080=CARTESIAN_POINT ( 'NONE',  ( 0.1787899950787401604, -1.006889763725763220, -0.07405724077823318263 ) ) ;
#32081=CARTESIAN_POINT ( 'NONE',  ( -0.1113553986120547346, -1.558070866141732180, 0.1113553986120547346 ) ) ;
#32092=CARTESIAN_POINT ( 'NONE',  ( -0.1465299180647509913, 0.09658349877441911591, -0.2008339832271239522 ) ) ;
#32094=CARTESIAN_POINT ( 'NONE',  ( 0.1120715992852186343, -0.09842519685039369248, -0.2207285028503088720 ) ) ;
#32098=CARTESIAN_POINT ( 'NONE',  ( -0.1730231402413970609, -0.09842519685039370636, 0.004655736871993992367 ) ) ;
#32100=CARTESIAN_POINT ( 'NONE',  ( 2.892866454678787531E-17, -0.09645669291338582196, 0.1574803149606299191 ) ) ;
#32107=CARTESIAN_POINT ( 'NONE',  ( 0.07405724077823318263, -1.252952755851747924, 0.1787899950787401604 ) ) ;
#32109=CARTESIAN_POINT ( 'NONE',  ( 0.1264236179284866091, -1.324311023568283341, 0.1264236179284866091 ) ) ;
#32111=DIRECTION ( 'NONE',  ( 0.000000000000000000, 0.000000000000000000, 1.000000000000000000 ) ) ;
#32112=CARTESIAN_POINT ( 'NONE',  ( -0.1797182628040039087, -0.5940398725751709907, -0.07444174185955065859 ) ) ;
#32115=CARTESIAN_POINT ( 'NONE',  ( 0.06523048226347956391, -0.1973425196850395746, -0.1574803149606300301 ) ) ;
#32127=CARTESIAN_POINT ( 'NONE',  ( 0.1264236179284866091, -0.5319881889226142357, -0.1264236179284866091 ) ) ;
#32128=CARTESIAN_POINT ( 'NONE',  ( 0.06523048226347956391, -1.117618110236220152, 0.1574803149606297803 ) ) ;
#32142=CARTESIAN_POINT ( 'NONE',  ( 0.000000000000000000, 0.1299212598425196763, 0.2007874015748031815 ) ) ;
#32148=CARTESIAN_POINT ( 'NONE',  ( -0.1574803149606297803, -0.1727362203649139838, 0.06523048226347956391 ) ) ;
#32155=CARTESIAN_POINT ( 'NONE',  ( -0.1643945842212350683, -0.09851383576920552665, -0.06716829673107893584 ) ) ;
#32164=CARTESIAN_POINT ( 'NONE',  ( -0.1264236179284866091, -0.2859251967966303098, -0.1264236179284866091 ) ) ;
#32165=CARTESIAN_POINT ( 'NONE',  ( 0.1787899950787401604, -0.8100393700249772788, 0.07405724077823318263 ) ) ;
#32172=CARTESIAN_POINT ( 'NONE',  ( -0.1264236179284866091, -0.1393956217725458580, -0.1264236179284866091 ) ) ;
#32173=CARTESIAN_POINT ( 'NONE',  ( 0.1264236179284866091, -0.2613188975840319284, 0.1264236179284866091 ) ) ;
#32174=CARTESIAN_POINT ( 'NONE',  ( -1.094772975963752103E-17, 0.1028543307624250058, -0.1787899950787401882 ) ) ;
#32181=CARTESIAN_POINT ( 'NONE',  ( 0.06523048226347956391, -0.8813976377952761343, 0.1574803149606297803 ) ) ;
#32183=CARTESIAN_POINT ( 'NONE',  ( 0.1270800023317771588, -1.757917825331076767, 0.1270800023317771588 ) ) ;
#32184=CARTESIAN_POINT ( 'NONE',  ( 0.1574803149606300301, -0.5123031494987715373, 0.06523048226347956391 ) ) ;
#32185=CARTESIAN_POINT ( 'NONE',  ( -0.1787899950787401882, -0.4335629920722205433, 0.000000000000000000 ) ) ;
#32187=CARTESIAN_POINT ( 'NONE',  ( 0.1877875577363964654, 0.07959431159475735540, -0.1770138738565708303 ) ) ;
#32193=CARTESIAN_POINT ( 'NONE',  ( -1.094772975963752103E-17, -0.1727362204186775607, -0.1787899950787401882 ) ) ;
#32195=CARTESIAN_POINT ( 'NONE',  ( 0.1264236179284866091, -1.088090551127338657, 0.1264236179284866091 ) ) ;
#32220=CARTESIAN_POINT ( 'NONE',  ( 0.1787899950787401882, 0.05364173233722811102, -2.189545951927503898E-17 ) ) ;
#32230=CARTESIAN_POINT ( 'NONE',  ( 0.1787899950787401882, -1.335261763504828947, -2.189545951927503898E-17 ) ) ;
#32233=CARTESIAN_POINT ( 'NONE',  ( -1.094772975963752103E-17, -0.1678149605761578844, -0.1787899950787401882 ) ) ;
#32239=CARTESIAN_POINT ( 'NONE',  ( 0.1264236179284866091, -1.526082677111590513, 0.1264236179284866091 ) ) ;
#32240=CARTESIAN_POINT ( 'NONE',  ( -0.1264236179284866091, -0.7485236219934803259, 0.1264236179284866091 ) ) ;
#32242=CARTESIAN_POINT ( 'NONE',  ( 0.1797182628040039365, -1.241185541866509645, -2.200913952912460540E-17 ) ) ;
#32256=CARTESIAN_POINT ( 'NONE',  ( 0.1787899950787401604, -0.02263779522182702425, 0.07405724077823318263 ) ) ;
#32270=CARTESIAN_POINT ( 'NONE',  ( 0.1264236179284866091, -0.06446850388324429360, 0.1264236179284866091 ) ) ;
#32281=CARTESIAN_POINT ( 'NONE',  ( 0.1574803149606300301, -0.4286417321759371513, -0.06523048226347956391 ) ) ;
#32282=CARTESIAN_POINT ( 'NONE',  ( 0.1787899950787401604, -1.754921259788755128, -0.07405724077823318263 ) ) ;
#32286=ADVANCED_FACE ( 'NONE', ( #16402 ), #26113, .T. ) ;
#32291=CARTESIAN_POINT ( 'NONE',  ( 0.07405724077823318263, -0.8702027083867192037, 0.1787899950787401604 ) ) ;
#32301=( BOUNDED_SURFACE ( )  B_SPLINE_SURFACE ( 1, 2, ( 
 ( #40145, #4194, #18822, #7100, #14778, #22179, #25804, #7804, #21726, #596, #39667, #36814, #47365, #6853, #43989, #3970, #18588, #33246, #36358, #14539, #30832, #37513, #27236, #15492, #37990, #44917, #15968, #1313, #22665, #828, #37268, #33721, #26750, #8747, #20003, #34403, #26515, #19296, #40843, #19534, #30135, #12612, #41309, #8036, #45626, #1548, #8989, #33952, #12129, #23387, #4422, #8511, #16197, #26284, #41790, #44676, #4669, #41076, #8273, #30370, #23611, #1073, #15734, #45401, #23141, #37757, #26996, #4912, #16433, #34184, #30592, #45155, #12372, #41544, #5150, #19772, #38223, #5383, #34642, #1794, #31062, #24546, #34888, #6565, #20941, #6318, #39148, #20706, #42723, #24782, #31987, #17589, #13307, #46107, #27936, #2952, #31289, #24092, #9940, #35580, #16661, #46576, #13759, #2722, #42502, #2031, #42025, #38701, #12843, #10176, #20478, #17353, #28399, #20239, #16883, #27474, #2492, #9708, #42966, #39380, #31525, #5630, #24321, #38919, #45867, #6081, #21174, #35808, #13082, #35347, #28162, #46341, #32233, #27713, #9231, #23846, #38459, #5873, #42276, #17119, #31758, #2260, #13526, #9477, #35115, #3910, #10654, #309, #36043, #11129, #18062, #36524, #21901, #43206, #21414, #10420, #6795, #7504, #43930, #32708, #3202, #33185, #14478, #14000, #18760, #22123, #29617, #39851, #47301, #25749, #28649, #29135, #36751, #46813, #14955, #17830, #43451, #25020, #32475, #3450, #44158, #39618, #47054, #18531, #25262, #14249, #66, #43690, #36981, #28891, #10896, #25519, #32945, #40087, #40319, #7040, #29385, #11358, #21666, #25966, #3679, #40549, #36298, #7742, #22356, #4139, #7284, #18303, #14710, #45333, #5086, #38157, #33890, #19234, #1011, #23553, #4356, #44612, #30528, #15904, #37212, #19708, #34349, #8684, #15668, #22599, #15190, #11829, #33420, #30769, #41017, #45088, #37933, #40783, #37449, #534, #23077, #30305, #12305, #23320, #4600, #26216, #44855, #12065, #18992, #26689, #16137, #12550, #33651, #41240, #1250, #19470, #1480, #765, #27172, #41725, #26927, #26452, #8929, #8445, #37691, #22834, #4844, #34122, #41478, #29838, #8207, #44381, #15426, #11591, #7977, #30074, #42439, #16371, #41958, #30995, #27414, #28103, #17057, #38631, #20415, #2431, #13694, #42663, #5564, #13008, #34573, #13250, #42901, #31225, #9165, #24720, #13472, #6025, #20646, #45801, #23780, #2199, #5805, #27651, #9879, #38394, #10111, #31698, #16819, #39320, #17294, #31927, #9645, #39083, #24263, #24489, #42207, #16599, #19937, #1726, #35050, #31459, #46043, #45558, #6255, #12778, #20881, #35291, #20174, #9409, #38859, #46282, #24027, #35523, #27879, #2663, #46515, #34825, #28329, #1968, #28829, #11300, #11070, #17525, #40261, #13938, #17999, #32651, #10356, #17298, #35530, #9416, #28336, #24268, #16823, #13255, #9652, #38639, #21122, #38865, #10116, #34830, #2895, #13015, #41964, #6028, #5812, #20421, #42671, #42214, #24036, #46521, #20650, #27658, #24726, #27884, #2205, #35296, #28110, #35055, #39327, #2435, #46757, #42445, #42908, #31466, #46048, #24496, #17060, #31702, #46287, #39090, #13943, #23788, #6503, #6262, #35755, #32165, #20888, #38400, #2668, #5571, #20182, #1974, #16604, #31230, #10362, #46995, #21358, #29328, #40266, #43873, #6739, #255, #7451, #35985, #36471, #25203, #24968, #3146, #33367, #22072, #14657, #11076, #6983, #17770, #10843, #47242, #39788, #18480, #32418, #18706, #25695, #25458, #485, #25917, #40499, #18247, #14901, #32889, #33130, #21606, #36241, #28588, #43152, #14424, #43633, #40030, #39563, #29562, #14188, #44112, #36700, #28835, #3391, #3626, #5, #18003, #3859, #7225, #11305, #7685, #43392, #22304, #32656, #29076, #36936, #4086, #10605, #21848, #22544, #715, #41192, #11536, #37884, #8634, #30022, #34302, #44806, #37390, #33841, #30258, #11785, #41674, #12018, #30712, #7926, #23513, #33602, #15140, #26642, #26403, #40965, #15857, #15372, #44569, #19660, #8397, #18940, #45283, #959, #22782, #23024, #34075, #8156, #12500, #37639, #19892, #15617, #5040, #4548, #19180, #45039, #4794, #19420, #1202, #30479, #34522, #29786, #1429, #12255, #27124, #16091, #26874, #44334, #41437, #23268, #8879, #38115, #26162, #5278, #40731, #37162, #4308, #2378, #13431, #17016, #27366, #20834, #28061, #41909, #9599, #45752, #30951, #9120, #24676, #12963, #23737, #45516, #38341, #39273, #27603, #5518, #6448, #42621, #35244, #31653, #42152, #20133, #31419, #20367, #9361, #39039, #34778, #21064, #46226, #45995, #1679, #46463, #13647, #38818, #35474, #5978, #6204, #23983, #38584, #16325, #12736, #35005, #16779, #13205, #1918, #2612, #16552, #17249, #9831, #31180, #5758, #24219, #20599, #2152, #24438, #27838, #31886, #28285, #42399, #42849, #10058, #10544, #36641, #39975, #3802, #22015, #43098, #21299, #14371, #32109, #11015, #29271, #3088, #7402, #17942, #25141, #6919, #3339, #32364, #14837, #32600, #18419, #28529, #44050, #6681, #35702, #47189, #46941, #14130, #36417, #35925, #17710, #40210, #29017, #39507, #33067, #21543, #43343, #43574, #7167, #28775, #191, #10787, #40440, #36181, #25634, #39733, #25396, #18192, #21792, #3574, #32831, #47427, #7628, #2839, #29503, #14598, #11249, #25859, #43816, #17473, #46696, #13886, #10304, #24917, #4028, #26098, #18647, #40669, #15083, #22965, #34014, #37573, #431, #41372, #1139, #29730, #30200, #18883, #8338, #8572, #7866, #23208, #34243, #4733, #15309, #12188, #37333, #15561, #11726, #897, #41138, #11963, #26815, #33540, #37822, #11474, #15799, #40905, #26582, #44744, #33304, #44272, #22483, #37099, #30425, #19358, #8103, #22723, #44975, #16029, #4979, #4248, #29961, #36873, #19601, #654, #1372, #4480, #44508, #41609, #30655, #45216, #26345, #19121, #12436, #27059, #22243, #37223, #19242, #15435, #36534, #43940, #29145, #18314, #3918, #30089, #43699, #40097, #22610, #25757, #25532, #543, #29627, #37460, #14722, #18542, #25976, #33430, #33197, #44391, #3690, #29848, #11605, #11138, #26227, #36992, #40792, #21911, #41026, #7986, #4369, #19000, #7751, #33661, #11837, #775, #4610, #318, #14971, #40560, #47311, #29394, #40327, #26466, #8221, #7513, #22846, #14485, #7292, #22368, #36762, #4147, #18774, #15199, #31236, #41489, #45570, #38404, #41253, #37945, #1022, #5327, #45344, #16381, #9173, #5094, #26699, #27181, #41736, #37702, #8938, #16609, #13021, #1258, #19947, #12790, #30316 ),
 ( #23793, #34585, #27425, #23330, #41968, #5577, #34834, #1979, #45101, #45813, #23084, #27662, #42219, #9424, #24042, #44865, #8455, #12074, #12319, #5818, #32174, #39096, #20896, #2902, #14195, #28598, #6032, #13484, #35059, #13707, #42451, #21365, #2673, #2210, #39797, #43160, #3152, #28113, #6267, #46763, #16829, #17304, #24974, #27891, #35993, #9657, #17067, #24273, #38869, #46527, #32425, #35301, #31707, #39569, #46292, #42676, #21127, #28343, #10609, #9888, #24733, #35761, #47002, #28840, #43399, #10852, #36939, #18712, #3633, #4090, #44115, #33372, #29084, #720, #15146, #490, #11545, #14907, #26168, #33607, #40737, #26408, #22080, #40273, #3867, #44572, #25465, #18255, #7932, #15380, #7234, #6989, #21614, #36248, #18486, #43642, #3399, #32897, #18010, #47250, #14664, #21854, #36480, #15, #11082, #29338, #11310, #43881, #33134, #25702, #262, #25924, #40506, #7695, #22309, #19899, #45521, #12743, #965, #27374, #5524, #30263, #1437, #37645, #22789, #44812, #31186, #23274, #41196, #12970, #20138, #27131, #1925, #37889, #8402, #5047, #19667, #16097, #40973, #30720, #8161, #11259, #11026, #29280, #25643, #441, #15094, #45565, #1487, #16376, #15910, #30533, #31229, #11834, #8690, #23324, #45339, #4606, #12784, #41730, #27420, #8934, #26460, #23559, #38162, #34579, #20649, #13701, #13478, #28335, #28587, #3144, #21121, #42443, #35295, #46756, #42907, #43151, #32164, #5811, #31465, #24495, #42213, #2893, #39326, #27883, #17532, #28109, #2434, #46286, #42670, #9651, #24967, #9882, #10361, #38638, #21356, #46047, #45807, #39089, #24267, #6261, #10115, #20887, #6501, #39562, #17769, #2204, #13014, #27657, #9415, #24034, #20420, #25457, #15139, #25694, #4307, #18246, #22303, #47240, #43632, #14900, #40029, #21847, #40265, #18002, #32417, #25202, #36935, #4, #29785, #4085, #7450, #36240, #21605, #36699, #3858, #33129, #44111, #253, #18479, #18704, #11304, #29561, #25916, #40497, #7684, #33366, #7925, #11535, #26161, #40730, #22543, #27365, #26291, #379, #11199, #22425, #11423, #15033, #30142, #135, #3749, #22671, #4200, #18371, #37519, #19304, #29903, #41082, #44453, #8280, #44222, #26042, #25812, #40616, #7811, #18829, #33485, #8042, #22907, #33727, #33959, #836, #1081, #15742, #1802, #16441, #34411, #45632, #41798, #31069, #42285, #16891, #2037, #23393, #1553, #27721, #12852, #9484, #13089, #34191, #12381, #5390, #23148, #16667, #20250, #41549, #45877, #8997, #16208, #45407, #23620, #37997, #5879, #38232, #24102, #19543, #35121, #45160, #26759, #20010, #5157, #19778, #27483, #27002, #8754, #31297, #42035, #30597, #38709, #12621, #30841, #9237, #23856, #27242, #20486, #38467, #31536, #5638, #2270, #34896, #46117, #41316, #8519, #37763, #4921, #1318, #15975, #18072, #32483, #28407, #10664, #47066, #31768, #42511, #17598, #39159, #21183, #36051, #9716, #3460, #25271, #39859, #2962, #28899, #32240, #43458, #6329, #9946, #32719, #13314, #10185, #24791, #35814, #24329, #7051, #38928, #21675, #14009, #6090, #35591, #46822, #28658, #43221, #10428, #36306, #35358, #2503, #17126, #46351, #24551, #28170, #45036, #958, #12254, #30477, #4084, #29783, #22781, #40496, #19419, #37638, #11534, #15856, #26402, #18939, #15370, #11784, #40729, #23267, #40964, #26873, #36934, #5039, #15138, #44110, #8154, #7924, #22542, #44805, #44333, #26160, #1201, #37388, #484, #41436, #30021, #4306, #4547, #15616, #37159, #8631, #19178, #1427, #44568, #34074, #33600, #714, #26640, #33840, #30257, #12016, #41190, #16089, #11302, #37883, #8396, #19659, #34301, #23023, #25915, #4793, #7683, #22302, #18702, #33365, #34520, #12499, #1678, #23512, #31418, #9598, #45994, #8878, #2377, #24218, #38114, #38583, #27364, #27122, #5275, #6203, #41908, #19891, #35473, #38817, #13204, #5976, #9118, #30950, #12961, #1917, #23736, #20597, #45515, #20833, #35243, #27602, #42151, #12735, #45282, #41673, #31652, #16550, #28060, #13430, #38340, #5517, #35004, #20132, #9360, #42620, #34777, #31179, #45751, #23982, #5757, #24437, #39038, #2151, #42847, #36416, #29016, #24675, #25140, #13884, #46462, #39272, #40208, #28528, #6447, #22014, #10786, #3337, #17941, #43097, #21063, #46940, #35924, #10303, #7166, #35701, #7401, #47188, #14129, #36640, #14597, #29270, #6918, #3573, #21542, #21790, #24916, #39506, #17248, #31885, #3087, #32362, #28774, #13646, #18191, #28284, #32830, #32599, #2838, #21298, #39732, #36180, #17709, #14370, #43342, #43572, #47425, #17472, #39974, #10543, #25395, #43815, #11014, #25633, #32107, #46695, #36872, #29960, #190, #26581, #44743, #18646, #22964, #33539, #26097, #22482, #18882, #430, #30424, #652, #19357, #44049, #12187, #22242, #3800, #15307, #15082, #29728, #4479, #4027, #33303, #8337, #44507, #7626, #34013, #37098, #11472, #11725, #22722, #44271, #1138, #26344, #8570, #4247, #41137, #40668, #7865, #896, #40904, #8102, #41371, #15560, #37332, #23207, #15798, #44974, #19119, #37571, #30199, #4732, #11962, #26813, #33066, #14836, #29502, #11247, #25858, #40439, #42975, #19600, #10184, #38525, #28657, #30896, #12908, #27539, #45452, #9297, #5453, #42092, #6571, #43220, #13766, #34462, #12674, #39388, #23917, #21181, #24790, #45215, #23448, #16490, #34242, #28406, #31994, #5207, #35813, #20070, #27299, #9055, #34715, #1612, #17597, #1854, #2961, #30653, #46821, #8810, #37821, #31123, #16261, #41851, #5695, #38050, #19832, #32239, #45686, #41608, #14008, #23676, #38283, #20305, #34945, #2092, #10427, #16721, #4978, #46585, #1371, #16028, #12435, #27057, #39858, #25270, #21910, #43457, #29847, #44390, #14970, #43698, #22367, #11366, #10663, #39624, #29393, #3459, #3689, #3917, #6802, #28898, #21422, #7050, #17839, #7512, #36761, #22133, #3209, #25975, #33196, #32482, #32953, #36305, #36050, #47065, #542, #18071, #14256, #25028, #317, #29626, #40559, #32718, #47310, #7291, #10908, #29144, #7750, #25531, #40096, #36533, #36991, #4146, #18313, #74, #18773, #33429, #15198, #14721, #43939, #23562, #26936, #4609, #1490, #26698, #4856, #1021, #23083, #30537, #1257, #16147, #22845, #12556, #774, #23329, #30315, #15912, #34130, #7985, #33660, #22609, #18999, #19716, #8694, #44864, #12073, #41488, #5326, #34355, #44623, #19241, #26226, #19478, #15434, #45343, #41252, #40791, #31001, #30777, #41735, #33902, #8454, #37944, #37222, #37701 ),
 ( #11836, #45100, #4368, #27180, #5093, #26465, #8937, #12318, #15678, #38164, #19946, #8220, #34584, #1737, #16380, #30088, #11604, #41025, #37459, #9656, #9423, #24041, #46291, #45812, #13020, #2672, #13262, #1978, #13706, #31469, #5817, #27890, #17066, #38643, #28342, #42450, #2900, #16828, #35533, #27661, #42218, #28112, #20425, #35058, #24272, #16608, #17537, #45569, #17303, #38868, #12789, #46052, #31938, #2209, #6031, #42675, #20655, #35300, #2438, #31235, #27424, #41967, #46526, #31706, #42914, #10123, #13483, #9172, #9887, #24501, #39095, #6266, #23792, #24732, #38403, #39330, #5576, #6509, #21126, #35759, #20185, #34833, #36478, #10368, #47248, #32424, #46761, #43158, #3865, #47000, #39567, #33133, #18253, #25463, #40037, #14193, #6744, #3397, #39796, #28839, #13, #24972, #18485, #7233, #18008, #261, #40272, #7458, #29082, #29336, #43639, #14662, #43397, #10608, #32172, #13947, #36246, #32662, #14430, #21363, #11081, #35990, #25700, #21853, #28597, #10850, #32895, #43879, #3631, #22079, #36704, #3151, #17776, #25207, #6988, #21612, #2367, #28517, #31873, #43089, #13874, #34997, #13193, #20822, #23972, #2830, #21053, #42389, #10293, #9825, #17004, #46219, #42610, #24207, #6672, #24430, #39498, #2142, #35914, #45984, #27593, #39030, #5969, #20588, #28274, #27829, #9588, #21290, #35461, #31409, #3072, #13419, #35235, #2605, #46452, #31643, #17702, #32350, #16768, #28051, #42142, #17237, #13635, #10048, #17463, #42838, #39261, #6438, #35693, #46929, #9351, #11462, #40656, #47175, #29260, #29492, #178, #418, #17934, #15070, #26081, #44036, #7155, #4016, #43804, #7394, #3565, #25622, #33058, #3792, #18635, #25386, #29717, #3321, #25848, #32819, #18409, #36629, #10534, #36167, #25131, #21529, #22228, #11237, #47412, #14586, #40430, #7853, #36861, #14358, #21779, #28762, #22004, #29006, #22471, #11004, #43332, #33526, #33295, #37089, #36407, #40197, #4237, #39721, #14825, #18867, #14120, #6907, #43563, #10775, #39962, #18178, #4722, #30883, #44492, #40895, #23432, #26569, #29947, #1364, #30416, #38273, #19107, #19346, #44965, #34233, #34000, #45202, #4466, #30641, #12426, #44732, #27046, #37809, #41594, #22711, #41839, #8799, #38040, #5197, #8561, #19823, #12665, #34451, #5440, #1128, #15787, #12176, #20057, #33772, #11948, #1597, #16251, #883, #45443, #27290, #9044, #26800, #37317, #11709, #41124, #642, #23665, #8321, #15295, #26334, #15543, #8088, #41358, #22952, #23195, #4962, #37562, #30187, #19589, #16018, #27528, #43025, #5682, #34700, #46163, #45921, #13136, #35405, #34935, #16709, #39200, #2310, #20292, #2777, #16940, #42330, #31580, #2545, #27770, #17401, #13359, #39440, #27987, #24601, #31338, #9525, #17176, #42554, #9760, #42775, #9991, #6620, #1844, #6377, #20988, #32040, #46631, #13815, #16482, #28456, #10231, #24839, #31111, #45676, #42080, #9285, #23904, #14055, #21957, #33003, #36577, #46870, #40376, #125, #28702, #29201, #17882, #3011, #43275, #44213, #32527, #10476, #26031, #14775, #7344, #3739, #47113, #25074, #3509, #39909, #14304, #11191, #39664, #11413, #18360, #18120, #40606, #18586, #33244, #10951, #7563, #25571, #25802, #28947, #43508, #21233, #35859, #7097, #36356, #32766, #17645, #22176, #36812, #6849, #10717, #32291, #21467, #25323, #3968, #36099, #3257, #43987, #21724, #47363, #29439, #14536, #43751, #40142, #369, #15022, #29675, #41074, #4910, #11659, #37755, #19532, #4420, #40841, #826, #22418, #1071, #29896, #41543, #22898, #37041, #27234, #30590, #37988, #15490, #26513, #34182, #8745, #4192, #8271, #12127, #23385, #44440, #19051, #18820, #26281, #11892, #5148, #33476, #594, #45153, #33719, #15251, #8509, #37511, #45399, #8034, #4667, #19294, #41307, #15732, #1311, #22663, #15966, #12370, #30133, #26994, #44915, #19770, #37266, #1545, #34401, #16194, #30830, #30369, #12610, #7802, #44674, #26748, #23139, #27711, #42274, #31985, #12841, #5628, #38917, #24319, #45624, #28160, #42721, #17116, #9475, #31060, #23609, #20237, #41788, #39146, #2029, #6079, #46339, #1792, #45865, #8987, #31523, #24090, #20704, #31756, #13080, #34640, #38699, #5871, #27472, #20476, #24544, #20938, #42023, #35113, #9706, #27934, #9938, #9229, #6316, #35578, #35345, #34886, #13524, #2258, #16881, #31287, #46105, #13304, #42500, #2720, #16659, #17351, #23844, #2490, #46574, #13757, #38221, #5381, #16431, #20001, #38457, #36522, #25517, #47052, #28889, #10894, #22121, #3677, #13998, #21412, #42964, #21664, #2950, #14708, #43449, #10174, #306, #18301, #11127, #36041, #14247, #40084, #29383, #24780, #10652, #32706, #43927, #17587, #25018, #39378, #46811, #32473, #25748, #6563, #21172, #32943, #6793, #35806, #29133, #25260, #18529, #28647, #39849, #7038, #14476, #36295, #7282, #32230, #21899, #64, #39616, #40317, #18060, #7502, #43204, #36749, #3907, #33183, #28397, #3448, #10418, #3200, #17828, #47299, #43688, #762, #15424, #5083, #33418, #26214, #12063, #44853, #18757, #1247, #15901, #37689, #30072, #4135, #44156, #40781, #14953, #12302, #22597, #26687, #19466, #22353, #18990, #29614, #4597, #44610, #41238, #4841, #33649, #7738, #11826, #26449, #532, #41014, #45085, #41475, #15188, #8205, #30303, #1009, #30525, #29836, #26925, #8681, #8443, #7974, #34119, #22831, #37446, #4354, #19232, #33888, #15665, #23316, #37210, #37930, #44379, #23075, #19705, #34346, #11356, #25964, #36979, #40546, #11589, #9642, #46040, #20171, #31222, #31456, #42661, #24260, #35289, #2429, #6022, #45798, #5318, #30766, #9162, #1477, #13470, #23777, #13247, #20644, #8926, #5561, #45330, #38628, #13005, #27876, #28101, #27648, #41722, #42204, #9406, #19934, #24024, #9877, #24487, #34570, #5802, #16816, #2196, #39081, #1723, #6253, #20878, #42437, #38391, #12547, #20412, #16368, #30992, #45555, #12775, #25197, #40025, #46749, #36466, #24718, #14420, #21349, #39782, #10599, #46514, #10109, #13692, #42899, #43627, #29070, #35978, #3136, #25451, #44498, #7220, #21112, #28581, #2661, #28827, #6495, #21842, #32412, #17292, #8095, #3622, #18875, #10354, #46990, #33533, #647, #28327, #14183, #6976, #15301, #24961, #43387, #21600, #36236, #3386, #11718, #26339, #40900, #35521, #1135, #4473, #23440, #4971, #12902, #41130, #41367, #19597, #8805, #8567, #19828, #26575, #5204, #34456, #19351, #1605, #12433, #16255, #44737, #16488, #30890 ) ),
 .UNSPECIFIED., .F., .F., .T. ) 
 B_SPLINE_SURFACE_WITH_KNOTS ( ( 2, 1, 2 ),
 ( 3, 2, 2, 2, 2, 2, 2, 2, 2, 2, 2, 2, 2, 2, 2, 2, 2, 2, 2, 2, 2, 2, 2, 2, 2, 2, 2, 2, 2, 2, 2, 2, 2, 2, 2, 2, 2, 2, 2, 2, 2, 2, 2, 2, 2, 2, 2, 2, 2, 2, 2, 2, 2, 2, 2, 2, 2, 2, 2, 2, 2, 2, 2, 2, 2, 2, 2, 2, 2, 2, 2, 2, 2, 2, 2, 2, 2, 2, 2, 2, 2, 2, 2, 2, 2, 2, 2, 2, 2, 2, 2, 2, 2, 2, 2, 2, 2, 2, 2, 2, 2, 2, 2, 2, 2, 2, 2, 2, 2, 2, 2, 2, 2, 2, 2, 2, 2, 2, 2, 2, 2, 2, 2, 2, 2, 2, 2, 2, 2, 2, 2, 2, 2, 2, 2, 2, 2, 2, 2, 2, 2, 2, 2, 2, 2, 2, 2, 2, 2, 2, 2, 2, 2, 2, 2, 2, 2, 2, 2, 2, 2, 2, 2, 2, 2, 2, 2, 2, 2, 2, 2, 2, 2, 2, 2, 2, 2, 2, 2, 2, 2, 2, 2, 2, 2, 2, 2, 2, 2, 2, 2, 2, 2, 2, 2, 2, 2, 2, 2, 2, 2, 2, 2, 2, 2, 2, 2, 2, 2, 2, 2, 2, 2, 2, 2, 2, 2, 2, 2, 2, 2, 2, 2, 2, 2, 2, 2, 2, 2, 2, 2, 2, 2, 2, 2, 2, 2, 2, 2, 2, 2, 2, 2, 2, 2, 2, 2, 2, 2, 2, 2, 2, 2, 2, 2, 2, 2, 2, 2, 2, 2, 2, 2, 2, 2, 2, 2, 2, 2, 2, 2, 2, 2, 2, 2, 2, 2, 2, 2, 2, 2, 2, 2, 2, 2, 2, 2, 2, 2, 2, 2, 2, 2, 2, 2, 2, 2, 2, 2, 2, 2, 2, 2, 2, 2, 2, 2, 2, 2, 2, 2, 2, 2, 2, 2, 2, 2, 2, 2, 2, 2, 2, 2, 2, 2, 2, 2, 2, 2, 2, 2, 2, 2, 2, 2, 2, 2, 2, 2, 2, 2, 2, 2, 2, 2, 2, 2, 2, 2, 2, 2, 2, 2, 2, 2, 2, 2, 2, 2, 2, 2, 2, 2, 2, 2, 2, 2, 2, 2, 2, 2, 2, 2, 2, 2, 2, 2, 2, 2, 2, 2, 2, 2, 2, 2, 2, 2, 2, 2, 2, 2, 2, 2, 2, 2, 2, 2, 2, 2, 2, 3 ),
 ( 0.000000000000000000, 1.000000000000000000, 3.225190355106064999 ),
 ( 0.000000000000000000, 0.002500000000000000052, 0.005000000000000000104, 0.007499999999999999722, 0.01000000000000000021, 0.01250000000000000069, 0.01499999999999999944, 0.01750000000000000167, 0.02000000000000000042, 0.02249999999999999917, 0.02500000000000000139, 0.02750000000000000014, 0.02999999999999999889, 0.03250000000000000111, 0.03500000000000000333, 0.03749999999999999861, 0.04000000000000000083, 0.04250000000000000305, 0.04499999999999999833, 0.04750000000000000056, 0.05000000000000000278, 0.05249999999999999806, 0.05500000000000000028, 0.05750000000000000250, 0.05999999999999999778, 0.06250000000000000000, 0.06500000000000000222, 0.06750000000000000444, 0.07000000000000000666, 0.07249999999999999500, 0.07499999999999999722, 0.07749999999999999944, 0.08000000000000000167, 0.08250000000000000389, 0.08500000000000000611, 0.08749999999999999445, 0.08999999999999999667, 0.09249999999999999889, 0.09500000000000000111, 0.09750000000000000333, 0.1000000000000000056, 0.1024999999999999939, 0.1049999999999999961, 0.1074999999999999983, 0.1100000000000000006, 0.1125000000000000028, 0.1150000000000000050, 0.1174999999999999933, 0.1199999999999999956, 0.1224999999999999978, 0.1250000000000000000, 0.1275000000000000022, 0.1300000000000000044, 0.1325000000000000067, 0.1350000000000000089, 0.1375000000000000111, 0.1400000000000000133, 0.1424999999999999878, 0.1449999999999999900, 0.1474999999999999922, 0.1499999999999999944, 0.1524999999999999967, 0.1549999999999999989, 0.1575000000000000011, 0.1600000000000000033, 0.1625000000000000056, 0.1650000000000000078, 0.1675000000000000100, 0.1700000000000000122, 0.1724999999999999867, 0.1749999999999999889, 0.1774999999999999911, 0.1799999999999999933, 0.1824999999999999956, 0.1849999999999999978, 0.1875000000000000000, 0.1900000000000000022, 0.1925000000000000044, 0.1950000000000000067, 0.1975000000000000089, 0.2000000000000000111, 0.2025000000000000133, 0.2049999999999999878, 0.2074999999999999900, 0.2099999999999999922, 0.2124999999999999944, 0.2149999999999999967, 0.2174999999999999989, 0.2200000000000000011, 0.2225000000000000033, 0.2250000000000000056, 0.2275000000000000078, 0.2300000000000000100, 0.2325000000000000122, 0.2349999999999999867, 0.2374999999999999889, 0.2399999999999999911, 0.2424999999999999933, 0.2449999999999999956, 0.2474999999999999978, 0.2500000000000000000, 0.2525000000000000022, 0.2550000000000000044, 0.2575000000000000067, 0.2600000000000000089, 0.2625000000000000111, 0.2650000000000000133, 0.2675000000000000155, 0.2700000000000000178, 0.2725000000000000200, 0.2750000000000000222, 0.2775000000000000244, 0.2800000000000000266, 0.2824999999999999734, 0.2849999999999999756, 0.2874999999999999778, 0.2899999999999999800, 0.2924999999999999822, 0.2949999999999999845, 0.2974999999999999867, 0.2999999999999999889, 0.3024999999999999911, 0.3049999999999999933, 0.3074999999999999956, 0.3099999999999999978, 0.3125000000000000000, 0.3150000000000000022, 0.3175000000000000044, 0.3200000000000000067, 0.3225000000000000089, 0.3250000000000000111, 0.3275000000000000133, 0.3300000000000000155, 0.3325000000000000178, 0.3350000000000000200, 0.3375000000000000222, 0.3400000000000000244, 0.3425000000000000266, 0.3449999999999999734, 0.3474999999999999756, 0.3499999999999999778, 0.3524999999999999800, 0.3549999999999999822, 0.3574999999999999845, 0.3599999999999999867, 0.3624999999999999889, 0.3649999999999999911, 0.3674999999999999933, 0.3699999999999999956, 0.3724999999999999978, 0.3750000000000000000, 0.3775000000000000022, 0.3800000000000000044, 0.3825000000000000067, 0.3850000000000000089, 0.3875000000000000111, 0.3900000000000000133, 0.3925000000000000155, 0.3950000000000000178, 0.3975000000000000200, 0.4000000000000000222, 0.4025000000000000244, 0.4050000000000000266, 0.4074999999999999734, 0.4099999999999999756, 0.4124999999999999778, 0.4149999999999999800, 0.4174999999999999822, 0.4199999999999999845, 0.4224999999999999867, 0.4249999999999999889, 0.4274999999999999911, 0.4299999999999999933, 0.4324999999999999956, 0.4349999999999999978, 0.4375000000000000000, 0.4400000000000000022, 0.4425000000000000044, 0.4450000000000000067, 0.4475000000000000089, 0.4500000000000000111, 0.4525000000000000133, 0.4550000000000000155, 0.4575000000000000178, 0.4600000000000000200, 0.4625000000000000222, 0.4650000000000000244, 0.4675000000000000266, 0.4699999999999999734, 0.4724999999999999756, 0.4749999999999999778, 0.4774999999999999800, 0.4799999999999999822, 0.4824999999999999845, 0.4849999999999999867, 0.4874999999999999889, 0.4899999999999999911, 0.4924999999999999933, 0.4949999999999999956, 0.4974999999999999978, 0.5000000000000000000, 0.5024999999999999467, 0.5050000000000000044, 0.5074999999999999512, 0.5100000000000000089, 0.5124999999999999556, 0.5150000000000000133, 0.5174999999999999600, 0.5200000000000000178, 0.5224999999999999645, 0.5250000000000000222, 0.5274999999999999689, 0.5300000000000000266, 0.5324999999999999734, 0.5350000000000000311, 0.5374999999999999778, 0.5400000000000000355, 0.5424999999999999822, 0.5450000000000000400, 0.5474999999999999867, 0.5500000000000000444, 0.5524999999999999911, 0.5550000000000000488, 0.5574999999999999956, 0.5600000000000000533, 0.5625000000000000000, 0.5649999999999999467, 0.5675000000000000044, 0.5699999999999999512, 0.5725000000000000089, 0.5749999999999999556, 0.5775000000000000133, 0.5799999999999999600, 0.5825000000000000178, 0.5849999999999999645, 0.5875000000000000222, 0.5899999999999999689, 0.5925000000000000266, 0.5949999999999999734, 0.5975000000000000311, 0.5999999999999999778, 0.6025000000000000355, 0.6049999999999999822, 0.6075000000000000400, 0.6099999999999999867, 0.6125000000000000444, 0.6149999999999999911, 0.6175000000000000488, 0.6199999999999999956, 0.6225000000000000533, 0.6250000000000000000, 0.6274999999999999467, 0.6300000000000000044, 0.6324999999999999512, 0.6350000000000000089, 0.6374999999999999556, 0.6400000000000000133, 0.6424999999999999600, 0.6450000000000000178, 0.6474999999999999645, 0.6500000000000000222, 0.6524999999999999689, 0.6550000000000000266, 0.6574999999999999734, 0.6600000000000000311, 0.6624999999999999778, 0.6650000000000000355, 0.6674999999999999822, 0.6700000000000000400, 0.6724999999999999867, 0.6750000000000000444, 0.6774999999999999911, 0.6800000000000000488, 0.6824999999999999956, 0.6850000000000000533, 0.6875000000000000000, 0.6899999999999999467, 0.6925000000000000044, 0.6949999999999999512, 0.6975000000000000089, 0.6999999999999999556, 0.7025000000000000133, 0.7049999999999999600, 0.7075000000000000178, 0.7099999999999999645, 0.7125000000000000222, 0.7149999999999999689, 0.7175000000000000266, 0.7199999999999999734, 0.7225000000000000311, 0.7249999999999999778, 0.7275000000000000355, 0.7299999999999999822, 0.7325000000000000400, 0.7349999999999999867, 0.7375000000000000444, 0.7399999999999999911, 0.7425000000000000488, 0.7449999999999999956, 0.7475000000000000533, 0.7500000000000000000, 0.7524999999999999467, 0.7550000000000000044, 0.7574999999999999512, 0.7600000000000000089, 0.7624999999999999556, 0.7650000000000000133, 0.7674999999999999600, 0.7700000000000000178, 0.7724999999999999645, 0.7750000000000000222, 0.7774999999999999689, 0.7800000000000000266, 0.7824999999999999734, 0.7850000000000000311, 0.7874999999999999778, 0.7900000000000000355, 0.7924999999999999822, 0.7950000000000000400, 0.7974999999999999867, 0.8000000000000000444, 0.8024999999999999911, 0.8050000000000000488, 0.8074999999999999956, 0.8100000000000000533, 0.8125000000000000000, 0.8149999999999999467, 0.8175000000000000044, 0.8199999999999999512, 0.8225000000000000089, 0.8249999999999999556, 0.8275000000000000133, 0.8299999999999999600, 0.8325000000000000178, 0.8349999999999999645, 0.8375000000000000222, 0.8399999999999999689, 0.8425000000000000266, 0.8449999999999999734, 0.8475000000000000311, 0.8499999999999999778, 0.8525000000000000355, 0.8549999999999999822, 0.8575000000000000400, 0.8599999999999999867, 0.8625000000000000444, 0.8649999999999999911, 0.8675000000000000488, 0.8699999999999999956, 0.8725000000000000533, 0.8750000000000000000, 0.8774999999999999467, 0.8800000000000000044, 0.8824999999999999512, 0.8850000000000000089, 0.8874999999999999556, 0.8900000000000000133, 0.8924999999999999600, 0.8950000000000000178, 0.8974999999999999645, 0.9000000000000000222, 0.9024999999999999689, 0.9050000000000000266, 0.9074999999999999734, 0.9100000000000000311, 0.9124999999999999778, 0.9150000000000000355, 0.9174999999999999822, 0.9200000000000000400, 0.9224999999999999867, 0.9250000000000000444, 0.9274999999999999911, 0.9300000000000000488, 0.9324999999999999956, 0.9350000000000000533, 0.9375000000000000000, 0.9399999999999999467, 0.9425000000000000044, 0.9449999999999999512, 0.9475000000000000089, 0.9499999999999999556, 0.9525000000000000133, 0.9549999999999999600, 0.9575000000000000178, 0.9599999999999999645, 0.9625000000000000222, 0.9649999999999999689, 0.9675000000000000266, 0.9699999999999999734, 0.9725000000000000311, 0.9749999999999999778, 0.9775000000000000355, 0.9799999999999999822, 0.9825000000000000400, 0.9849999999999999867, 0.9875000000000000444, 0.9899999999999999911, 0.9925000000000000488, 0.9949999999999999956, 0.9975000000000000533, 1.000000000000000000 ),
 .UNSPECIFIED. ) 
 GEOMETRIC_REPRESENTATION_ITEM ( )  RATIONAL_B_SPLINE_SURFACE ( (
 ( 1.000000000000000000, 0.9238795325112869605, 1.000000000000000000, 0.9238795325112869605, 1.000000000000000000, 0.9238795325112869605, 1.000000000000000000, 0.9238795325112869605, 1.000000000000000000, 0.9238795325112869605, 1.000000000000000000, 0.9238795325112869605, 1.000000000000000000, 0.9238795325112869605, 1.000000000000000000, 0.9238795325112869605, 1.000000000000000000, 0.9238795325112869605, 1.000000000000000000, 0.9238795325112869605, 1.000000000000000000, 0.9238795325112869605, 1.000000000000000000, 0.9238795325112869605, 1.000000000000000000, 0.9238795325112869605, 1.000000000000000000, 0.9238795325112869605, 1.000000000000000000, 0.9238795325112869605, 1.000000000000000000, 0.9238795325112869605, 1.000000000000000000, 0.9238795325112869605, 1.000000000000000000, 0.9238795325112869605, 1.000000000000000000, 0.9238795325112869605, 1.000000000000000000, 0.9238795325112869605, 1.000000000000000000, 0.9238795325112869605, 1.000000000000000000, 0.9238795325112869605, 1.000000000000000000, 0.9238795325112869605, 1.000000000000000000, 0.9238795325112869605, 1.000000000000000000, 0.9238795325112869605, 1.000000000000000000, 0.9238795325112869605, 1.000000000000000000, 0.9238795325112869605, 1.000000000000000000, 0.9238795325112869605, 1.000000000000000000, 0.9238795325112869605, 1.000000000000000000, 0.9238795325112869605, 1.000000000000000000, 0.9238795325112869605, 1.000000000000000000, 0.9238795325112869605, 1.000000000000000000, 0.9238795325112869605, 1.000000000000000000, 0.9238795325112869605, 1.000000000000000000, 0.9238795325112869605, 1.000000000000000000, 0.9238795325112869605, 1.000000000000000000, 0.9238795325112869605, 1.000000000000000000, 0.9238795325112869605, 1.000000000000000000, 0.9238795325112869605, 1.000000000000000000, 0.9238795325112869605, 1.000000000000000000, 0.9238795325112869605, 1.000000000000000000, 0.9238795325112869605, 1.000000000000000000, 0.9238795325112869605, 1.000000000000000000, 0.9238795325112869605, 1.000000000000000000, 0.9238795325112869605, 1.000000000000000000, 0.9238795325112869605, 1.000000000000000000, 0.9238795325112869605, 1.000000000000000000, 0.9238795325112869605, 1.000000000000000000, 0.9238795325112869605, 1.000000000000000000, 0.9238795325112869605, 1.000000000000000000, 0.9238795325112869605, 1.000000000000000000, 0.9238795325112869605, 1.000000000000000000, 0.9238795325112869605, 1.000000000000000000, 0.9238795325112869605, 1.000000000000000000, 0.9238795325112869605, 1.000000000000000000, 0.9238795325112869605, 1.000000000000000000, 0.9238795325112869605, 1.000000000000000000, 0.9238795325112869605, 1.000000000000000000, 0.9238795325112869605, 1.000000000000000000, 0.9238795325112869605, 1.000000000000000000, 0.9238795325112869605, 1.000000000000000000, 0.9238795325112869605, 1.000000000000000000, 0.9238795325112869605, 1.000000000000000000, 0.9238795325112869605, 1.000000000000000000, 0.9238795325112869605, 1.000000000000000000, 0.9238795325112869605, 1.000000000000000000, 0.9238795325112869605, 1.000000000000000000, 0.9238795325112869605, 1.000000000000000000, 0.9238795325112869605, 1.000000000000000000, 0.9238795325112869605, 1.000000000000000000, 0.9238795325112869605, 1.000000000000000000, 0.9238795325112869605, 1.000000000000000000, 0.9238795325112869605, 1.000000000000000000, 0.9238795325112869605, 1.000000000000000000, 0.9238795325112869605, 1.000000000000000000, 0.9238795325112869605, 1.000000000000000000, 0.9238795325112869605, 1.000000000000000000, 0.9238795325112869605, 1.000000000000000000, 0.9238795325112869605, 1.000000000000000000, 0.9238795325112869605, 1.000000000000000000, 0.9238795325112869605, 1.000000000000000000, 0.9238795325112869605, 1.000000000000000000, 0.9238795325112869605, 1.000000000000000000, 0.9238795325112869605, 1.000000000000000000, 0.9238795325112869605, 1.000000000000000000, 0.9238795325112869605, 1.000000000000000000, 0.9238795325112869605, 1.000000000000000000, 0.9238795325112869605, 1.000000000000000000, 0.9238795325112869605, 1.000000000000000000, 0.9238795325112869605, 1.000000000000000000, 0.9238795325112869605, 1.000000000000000000, 0.9238795325112869605, 1.000000000000000000, 0.9238795325112869605, 1.000000000000000000, 0.9238795325112869605, 1.000000000000000000, 0.9238795325112869605, 1.000000000000000000, 0.9238795325112869605, 1.000000000000000000, 0.9238795325112869605, 1.000000000000000000, 0.9238795325112869605, 1.000000000000000000, 0.9238795325112869605, 1.000000000000000000, 0.9238795325112869605, 1.000000000000000000, 0.9238795325112869605, 1.000000000000000000, 0.9238795325112869605, 1.000000000000000000, 0.9238795325112869605, 1.000000000000000000, 0.9238795325112869605, 1.000000000000000000, 0.9238795325112869605, 1.000000000000000000, 0.9238795325112869605, 1.000000000000000000, 0.9238795325112869605, 1.000000000000000000, 0.9238795325112869605, 1.000000000000000000, 0.9238795325112869605, 1.000000000000000000, 0.9238795325112869605, 1.000000000000000000, 0.9238795325112869605, 1.000000000000000000, 0.9238795325112869605, 1.000000000000000000, 0.9238795325112869605, 1.000000000000000000, 0.9238795325112869605, 1.000000000000000000, 0.9238795325112869605, 1.000000000000000000, 0.9238795325112869605, 1.000000000000000000, 0.9238795325112869605, 1.000000000000000000, 0.9238795325112869605, 1.000000000000000000, 0.9238795325112869605, 1.000000000000000000, 0.9238795325112869605, 1.000000000000000000, 0.9238795325112869605, 1.000000000000000000, 0.9238795325112869605, 1.000000000000000000, 0.9238795325112869605, 1.000000000000000000, 0.9238795325112869605, 1.000000000000000000, 0.9238795325112869605, 1.000000000000000000, 0.9238795325112869605, 1.000000000000000000, 0.9238795325112869605, 1.000000000000000000, 0.9238795325112869605, 1.000000000000000000, 0.9238795325112869605, 1.000000000000000000, 0.9238795325112869605, 1.000000000000000000, 0.9238795325112869605, 1.000000000000000000, 0.9238795325112869605, 1.000000000000000000, 0.9238795325112869605, 1.000000000000000000, 0.9238795325112869605, 1.000000000000000000, 0.9238795325112869605, 1.000000000000000000, 0.9238795325112869605, 1.000000000000000000, 0.9238795325112869605, 1.000000000000000000, 0.9238795325112869605, 1.000000000000000000, 0.9238795325112869605, 1.000000000000000000, 0.9238795325112869605, 1.000000000000000000, 0.9238795325112869605, 1.000000000000000000, 0.9238795325112869605, 1.000000000000000000, 0.9238795325112869605, 1.000000000000000000, 0.9238795325112869605, 1.000000000000000000, 0.9238795325112869605, 1.000000000000000000, 0.9238795325112869605, 1.000000000000000000, 0.9238795325112869605, 1.000000000000000000, 0.9238795325112869605, 1.000000000000000000, 0.9238795325112869605, 1.000000000000000000, 0.9238795325112869605, 1.000000000000000000, 0.9238795325112869605, 1.000000000000000000, 0.9238795325112869605, 1.000000000000000000, 0.9238795325112869605, 1.000000000000000000, 0.9238795325112869605, 1.000000000000000000, 0.9238795325112869605, 1.000000000000000000, 0.9238795325112869605, 1.000000000000000000, 0.9238795325112869605, 1.000000000000000000, 0.9238795325112869605, 1.000000000000000000, 0.9238795325112869605, 1.000000000000000000, 0.9238795325112869605, 1.000000000000000000, 0.9238795325112869605, 1.000000000000000000, 0.9238795325112869605, 1.000000000000000000, 0.9238795325112869605, 1.000000000000000000, 0.9238795325112869605, 1.000000000000000000, 0.9238795325112869605, 1.000000000000000000, 0.9238795325112869605, 1.000000000000000000, 0.9238795325112869605, 1.000000000000000000, 0.9238795325112869605, 1.000000000000000000, 0.9238795325112869605, 1.000000000000000000, 0.9238795325112869605, 1.000000000000000000, 0.9238795325112869605, 1.000000000000000000, 0.9238795325112869605, 1.000000000000000000, 0.9238795325112869605, 1.000000000000000000, 0.9238795325112869605, 1.000000000000000000, 0.9238795325112869605, 1.000000000000000000, 0.9238795325112869605, 1.000000000000000000, 0.9238795325112869605, 1.000000000000000000, 0.9238795325112869605, 1.000000000000000000, 0.9238795325112869605, 1.000000000000000000, 0.9238795325112869605, 1.000000000000000000, 0.9238795325112869605, 1.000000000000000000, 0.9238795325112869605, 1.000000000000000000, 0.9238795325112869605, 1.000000000000000000, 0.9238795325112869605, 1.000000000000000000, 0.9238795325112869605, 1.000000000000000000, 0.9238795325112869605, 1.000000000000000000, 0.9238795325112869605, 1.000000000000000000, 0.9238795325112869605, 1.000000000000000000, 0.9238795325112869605, 1.000000000000000000, 0.9238795325112869605, 1.000000000000000000, 0.9238795325112869605, 1.000000000000000000, 0.9238795325112869605, 1.000000000000000000, 0.9238795325112869605, 1.000000000000000000, 0.9238795325112869605, 1.000000000000000000, 0.9238795325112869605, 1.000000000000000000, 0.9238795325112869605, 1.000000000000000000, 0.9238795325112869605, 1.000000000000000000, 0.9238795325112869605, 1.000000000000000000, 0.9238795325112869605, 1.000000000000000000, 0.9238795325112869605, 1.000000000000000000, 0.9238795325112869605, 1.000000000000000000, 0.9238795325112869605, 1.000000000000000000, 0.9238795325112869605, 1.000000000000000000, 0.9238795325112869605, 1.000000000000000000, 0.9238795325112869605, 1.000000000000000000, 0.9238795325112869605, 1.000000000000000000, 0.9238795325112869605, 1.000000000000000000, 0.9238795325112869605, 1.000000000000000000, 0.9238795325112869605, 1.000000000000000000, 0.9238795325112869605, 1.000000000000000000, 0.9238795325112869605, 1.000000000000000000, 0.9238795325112869605, 1.000000000000000000, 0.9238795325112869605, 1.000000000000000000, 0.9238795325112869605, 1.000000000000000000, 0.9238795325112869605, 1.000000000000000000, 0.9238795325112869605, 1.000000000000000000, 0.9238795325112869605, 1.000000000000000000, 0.9238795325112869605, 1.000000000000000000, 0.9238795325112869605, 1.000000000000000000, 0.9238795325112869605, 1.000000000000000000, 0.9238795325112869605, 1.000000000000000000, 0.9238795325112869605, 1.000000000000000000, 0.9238795325112869605, 1.000000000000000000, 0.9238795325112869605, 1.000000000000000000, 0.9238795325112869605, 1.000000000000000000, 0.9238795325112869605, 1.000000000000000000, 0.9238795325112869605, 1.000000000000000000, 0.9238795325112869605, 1.000000000000000000, 0.9238795325112869605, 1.000000000000000000, 0.9238795325112869605, 1.000000000000000000, 0.9238795325112869605, 1.000000000000000000, 0.9238795325112869605, 1.000000000000000000, 0.9238795325112869605, 1.000000000000000000, 0.9238795325112869605, 1.000000000000000000, 0.9238795325112869605, 1.000000000000000000, 0.9238795325112869605, 1.000000000000000000, 0.9238795325112869605, 1.000000000000000000, 0.9238795325112869605, 1.000000000000000000, 0.9238795325112869605, 1.000000000000000000, 0.9238795325112869605, 1.000000000000000000, 0.9238795325112869605, 1.000000000000000000, 0.9238795325112869605, 1.000000000000000000, 0.9238795325112869605, 1.000000000000000000, 0.9238795325112869605, 1.000000000000000000, 0.9238795325112869605, 1.000000000000000000, 0.9238795325112869605, 1.000000000000000000, 0.9238795325112869605, 1.000000000000000000, 0.9238795325112869605, 1.000000000000000000, 0.9238795325112869605, 1.000000000000000000, 0.9238795325112869605, 1.000000000000000000, 0.9238795325112869605, 1.000000000000000000, 0.9238795325112869605, 1.000000000000000000, 0.9238795325112869605, 1.000000000000000000, 0.9238795325112869605, 1.000000000000000000, 0.9238795325112869605, 1.000000000000000000, 0.9238795325112869605, 1.000000000000000000, 0.9238795325112869605, 1.000000000000000000, 0.9238795325112869605, 1.000000000000000000, 0.9238795325112869605, 1.000000000000000000, 0.9238795325112869605, 1.000000000000000000, 0.9238795325112869605, 1.000000000000000000, 0.9238795325112869605, 1.000000000000000000, 0.9238795325112869605, 1.000000000000000000, 0.9238795325112869605, 1.000000000000000000, 0.9238795325112869605, 1.000000000000000000, 0.9238795325112869605, 1.000000000000000000, 0.9238795325112869605, 1.000000000000000000, 0.9238795325112869605, 1.000000000000000000, 0.9238795325112869605, 1.000000000000000000, 0.9238795325112869605, 1.000000000000000000, 0.9238795325112869605, 1.000000000000000000, 0.9238795325112869605, 1.000000000000000000, 0.9238795325112869605, 1.000000000000000000, 0.9238795325112869605, 1.000000000000000000, 0.9238795325112869605, 1.000000000000000000, 0.9238795325112869605, 1.000000000000000000, 0.9238795325112869605, 1.000000000000000000, 0.9238795325112869605, 1.000000000000000000, 0.9238795325112869605, 1.000000000000000000, 0.9238795325112869605, 1.000000000000000000, 0.9238795325112869605, 1.000000000000000000, 0.9238795325112869605, 1.000000000000000000, 0.9238795325112869605, 1.000000000000000000, 0.9238795325112869605, 1.000000000000000000, 0.9238795325112869605, 1.000000000000000000, 0.9238795325112869605, 1.000000000000000000, 0.9238795325112869605, 1.000000000000000000, 0.9238795325112869605, 1.000000000000000000, 0.9238795325112869605, 1.000000000000000000, 0.9238795325112869605, 1.000000000000000000, 0.9238795325112869605, 1.000000000000000000, 0.9238795325112869605, 1.000000000000000000, 0.9238795325112869605, 1.000000000000000000, 0.9238795325112869605, 1.000000000000000000, 0.9238795325112869605, 1.000000000000000000, 0.9238795325112869605, 1.000000000000000000, 0.9238795325112869605, 1.000000000000000000, 0.9238795325112869605, 1.000000000000000000, 0.9238795325112869605, 1.000000000000000000, 0.9238795325112869605, 1.000000000000000000, 0.9238795325112869605, 1.000000000000000000, 0.9238795325112869605, 1.000000000000000000, 0.9238795325112869605, 1.000000000000000000, 0.9238795325112869605, 1.000000000000000000, 0.9238795325112869605, 1.000000000000000000, 0.9238795325112869605, 1.000000000000000000, 0.9238795325112869605, 1.000000000000000000, 0.9238795325112869605, 1.000000000000000000, 0.9238795325112869605, 1.000000000000000000, 0.9238795325112869605, 1.000000000000000000, 0.9238795325112869605, 1.000000000000000000, 0.9238795325112869605, 1.000000000000000000, 0.9238795325112869605, 1.000000000000000000, 0.9238795325112869605, 1.000000000000000000, 0.9238795325112869605, 1.000000000000000000, 0.9238795325112869605, 1.000000000000000000, 0.9238795325112869605, 1.000000000000000000, 0.9238795325112869605, 1.000000000000000000, 0.9238795325112869605, 1.000000000000000000, 0.9238795325112869605, 1.000000000000000000, 0.9238795325112869605, 1.000000000000000000, 0.9238795325112869605, 1.000000000000000000, 0.9238795325112869605, 1.000000000000000000, 0.9238795325112869605, 1.000000000000000000, 0.9238795325112869605, 1.000000000000000000, 0.9238795325112869605, 1.000000000000000000, 0.9238795325112869605, 1.000000000000000000, 0.9238795325112869605, 1.000000000000000000, 0.9238795325112869605, 1.000000000000000000, 0.9238795325112869605, 1.000000000000000000, 0.9238795325112869605, 1.000000000000000000, 0.9238795325112869605, 1.000000000000000000, 0.9238795325112869605, 1.000000000000000000, 0.9238795325112869605, 1.000000000000000000, 0.9238795325112869605, 1.000000000000000000, 0.9238795325112869605, 1.000000000000000000, 0.9238795325112869605, 1.000000000000000000, 0.9238795325112869605, 1.000000000000000000, 0.9238795325112869605, 1.000000000000000000, 0.9238795325112869605, 1.000000000000000000, 0.9238795325112869605, 1.000000000000000000, 0.9238795325112869605, 1.000000000000000000, 0.9238795325112869605, 1.000000000000000000, 0.9238795325112869605, 1.000000000000000000, 0.9238795325112869605, 1.000000000000000000, 0.9238795325112869605, 1.000000000000000000, 0.9238795325112869605, 1.000000000000000000, 0.9238795325112869605, 1.000000000000000000, 0.9238795325112869605, 1.000000000000000000, 0.9238795325112869605, 1.000000000000000000, 0.9238795325112869605, 1.000000000000000000, 0.9238795325112869605, 1.000000000000000000, 0.9238795325112869605, 1.000000000000000000, 0.9238795325112869605, 1.000000000000000000, 0.9238795325112869605, 1.000000000000000000, 0.9238795325112869605, 1.000000000000000000, 0.9238795325112869605, 1.000000000000000000, 0.9238795325112869605, 1.000000000000000000, 0.9238795325112869605, 1.000000000000000000, 0.9238795325112869605, 1.000000000000000000, 0.9238795325112869605, 1.000000000000000000, 0.9238795325112869605, 1.000000000000000000, 0.9238795325112869605, 1.000000000000000000, 0.9238795325112869605, 1.000000000000000000, 0.9238795325112869605, 1.000000000000000000, 0.9238795325112869605, 1.000000000000000000, 0.9238795325112869605, 1.000000000000000000, 0.9238795325112869605, 1.000000000000000000, 0.9238795325112869605, 1.000000000000000000, 0.9238795325112869605, 1.000000000000000000, 0.9238795325112869605, 1.000000000000000000, 0.9238795325112869605, 1.000000000000000000, 0.9238795325112869605, 1.000000000000000000, 0.9238795325112869605, 1.000000000000000000, 0.9238795325112869605, 1.000000000000000000, 0.9238795325112869605, 1.000000000000000000, 0.9238795325112869605, 1.000000000000000000, 0.9238795325112869605, 1.000000000000000000, 0.9238795325112869605, 1.000000000000000000, 0.9238795325112869605, 1.000000000000000000, 0.9238795325112869605, 1.000000000000000000, 0.9238795325112869605, 1.000000000000000000, 0.9238795325112869605, 1.000000000000000000, 0.9238795325112869605, 1.000000000000000000, 0.9238795325112869605, 1.000000000000000000, 0.9238795325112869605, 1.000000000000000000, 0.9238795325112869605, 1.000000000000000000, 0.9238795325112869605, 1.000000000000000000, 0.9238795325112869605, 1.000000000000000000, 0.9238795325112869605, 1.000000000000000000, 0.9238795325112869605, 1.000000000000000000, 0.9238795325112869605, 1.000000000000000000, 0.9238795325112869605, 1.000000000000000000, 0.9238795325112869605, 1.000000000000000000, 0.9238795325112869605, 1.000000000000000000, 0.9238795325112869605, 1.000000000000000000, 0.9238795325112869605, 1.000000000000000000, 0.9238795325112869605, 1.000000000000000000, 0.9238795325112869605, 1.000000000000000000, 0.9238795325112869605, 1.000000000000000000),
 ( 1.000000000000000000, 0.9238795325112869605, 1.000000000000000000, 0.9238795325112869605, 1.000000000000000000, 0.9238795325112869605, 1.000000000000000000, 0.9238795325112869605, 1.000000000000000000, 0.9238795325112869605, 1.000000000000000000, 0.9238795325112869605, 1.000000000000000000, 0.9238795325112869605, 1.000000000000000000, 0.9238795325112869605, 1.000000000000000000, 0.9238795325112869605, 1.000000000000000000, 0.9238795325112869605, 1.000000000000000000, 0.9238795325112869605, 1.000000000000000000, 0.9238795325112869605, 1.000000000000000000, 0.9238795325112869605, 1.000000000000000000, 0.9238795325112869605, 1.000000000000000000, 0.9238795325112869605, 1.000000000000000000, 0.9238795325112869605, 1.000000000000000000, 0.9238795325112869605, 1.000000000000000000, 0.9238795325112869605, 1.000000000000000000, 0.9238795325112869605, 1.000000000000000000, 0.9238795325112869605, 1.000000000000000000, 0.9238795325112869605, 1.000000000000000000, 0.9238795325112869605, 1.000000000000000000, 0.9238795325112869605, 1.000000000000000000, 0.9238795325112869605, 1.000000000000000000, 0.9238795325112869605, 1.000000000000000000, 0.9238795325112869605, 1.000000000000000000, 0.9238795325112869605, 1.000000000000000000, 0.9238795325112869605, 1.000000000000000000, 0.9238795325112869605, 1.000000000000000000, 0.9238795325112869605, 1.000000000000000000, 0.9238795325112869605, 1.000000000000000000, 0.9238795325112869605, 1.000000000000000000, 0.9238795325112869605, 1.000000000000000000, 0.9238795325112869605, 1.000000000000000000, 0.9238795325112869605, 1.000000000000000000, 0.9238795325112869605, 1.000000000000000000, 0.9238795325112869605, 1.000000000000000000, 0.9238795325112869605, 1.000000000000000000, 0.9238795325112869605, 1.000000000000000000, 0.9238795325112869605, 1.000000000000000000, 0.9238795325112869605, 1.000000000000000000, 0.9238795325112869605, 1.000000000000000000, 0.9238795325112869605, 1.000000000000000000, 0.9238795325112869605, 1.000000000000000000, 0.9238795325112869605, 1.000000000000000000, 0.9238795325112869605, 1.000000000000000000, 0.9238795325112869605, 1.000000000000000000, 0.9238795325112869605, 1.000000000000000000, 0.9238795325112869605, 1.000000000000000000, 0.9238795325112869605, 1.000000000000000000, 0.9238795325112869605, 1.000000000000000000, 0.9238795325112869605, 1.000000000000000000, 0.9238795325112869605, 1.000000000000000000, 0.9238795325112869605, 1.000000000000000000, 0.9238795325112869605, 1.000000000000000000, 0.9238795325112869605, 1.000000000000000000, 0.9238795325112869605, 1.000000000000000000, 0.9238795325112869605, 1.000000000000000000, 0.9238795325112869605, 1.000000000000000000, 0.9238795325112869605, 1.000000000000000000, 0.9238795325112869605, 1.000000000000000000, 0.9238795325112869605, 1.000000000000000000, 0.9238795325112869605, 1.000000000000000000, 0.9238795325112869605, 1.000000000000000000, 0.9238795325112869605, 1.000000000000000000, 0.9238795325112869605, 1.000000000000000000, 0.9238795325112869605, 1.000000000000000000, 0.9238795325112869605, 1.000000000000000000, 0.9238795325112869605, 1.000000000000000000, 0.9238795325112869605, 1.000000000000000000, 0.9238795325112869605, 1.000000000000000000, 0.9238795325112869605, 1.000000000000000000, 0.9238795325112869605, 1.000000000000000000, 0.9238795325112869605, 1.000000000000000000, 0.9238795325112869605, 1.000000000000000000, 0.9238795325112869605, 1.000000000000000000, 0.9238795325112869605, 1.000000000000000000, 0.9238795325112869605, 1.000000000000000000, 0.9238795325112869605, 1.000000000000000000, 0.9238795325112869605, 1.000000000000000000, 0.9238795325112869605, 1.000000000000000000, 0.9238795325112869605, 1.000000000000000000, 0.9238795325112869605, 1.000000000000000000, 0.9238795325112869605, 1.000000000000000000, 0.9238795325112869605, 1.000000000000000000, 0.9238795325112869605, 1.000000000000000000, 0.9238795325112869605, 1.000000000000000000, 0.9238795325112869605, 1.000000000000000000, 0.9238795325112869605, 1.000000000000000000, 0.9238795325112869605, 1.000000000000000000, 0.9238795325112869605, 1.000000000000000000, 0.9238795325112869605, 1.000000000000000000, 0.9238795325112869605, 1.000000000000000000, 0.9238795325112869605, 1.000000000000000000, 0.9238795325112869605, 1.000000000000000000, 0.9238795325112869605, 1.000000000000000000, 0.9238795325112869605, 1.000000000000000000, 0.9238795325112869605, 1.000000000000000000, 0.9238795325112869605, 1.000000000000000000, 0.9238795325112869605, 1.000000000000000000, 0.9238795325112869605, 1.000000000000000000, 0.9238795325112869605, 1.000000000000000000, 0.9238795325112869605, 1.000000000000000000, 0.9238795325112869605, 1.000000000000000000, 0.9238795325112869605, 1.000000000000000000, 0.9238795325112869605, 1.000000000000000000, 0.9238795325112869605, 1.000000000000000000, 0.9238795325112869605, 1.000000000000000000, 0.9238795325112869605, 1.000000000000000000, 0.9238795325112869605, 1.000000000000000000, 0.9238795325112869605, 1.000000000000000000, 0.9238795325112869605, 1.000000000000000000, 0.9238795325112869605, 1.000000000000000000, 0.9238795325112869605, 1.000000000000000000, 0.9238795325112869605, 1.000000000000000000, 0.9238795325112869605, 1.000000000000000000, 0.9238795325112869605, 1.000000000000000000, 0.9238795325112869605, 1.000000000000000000, 0.9238795325112869605, 1.000000000000000000, 0.9238795325112869605, 1.000000000000000000, 0.9238795325112869605, 1.000000000000000000, 0.9238795325112869605, 1.000000000000000000, 0.9238795325112869605, 1.000000000000000000, 0.9238795325112869605, 1.000000000000000000, 0.9238795325112869605, 1.000000000000000000, 0.9238795325112869605, 1.000000000000000000, 0.9238795325112869605, 1.000000000000000000, 0.9238795325112869605, 1.000000000000000000, 0.9238795325112869605, 1.000000000000000000, 0.9238795325112869605, 1.000000000000000000, 0.9238795325112869605, 1.000000000000000000, 0.9238795325112869605, 1.000000000000000000, 0.9238795325112869605, 1.000000000000000000, 0.9238795325112869605, 1.000000000000000000, 0.9238795325112869605, 1.000000000000000000, 0.9238795325112869605, 1.000000000000000000, 0.9238795325112869605, 1.000000000000000000, 0.9238795325112869605, 1.000000000000000000, 0.9238795325112869605, 1.000000000000000000, 0.9238795325112869605, 1.000000000000000000, 0.9238795325112869605, 1.000000000000000000, 0.9238795325112869605, 1.000000000000000000, 0.9238795325112869605, 1.000000000000000000, 0.9238795325112869605, 1.000000000000000000, 0.9238795325112869605, 1.000000000000000000, 0.9238795325112869605, 1.000000000000000000, 0.9238795325112869605, 1.000000000000000000, 0.9238795325112869605, 1.000000000000000000, 0.9238795325112869605, 1.000000000000000000, 0.9238795325112869605, 1.000000000000000000, 0.9238795325112869605, 1.000000000000000000, 0.9238795325112869605, 1.000000000000000000, 0.9238795325112869605, 1.000000000000000000, 0.9238795325112869605, 1.000000000000000000, 0.9238795325112869605, 1.000000000000000000, 0.9238795325112869605, 1.000000000000000000, 0.9238795325112869605, 1.000000000000000000, 0.9238795325112869605, 1.000000000000000000, 0.9238795325112869605, 1.000000000000000000, 0.9238795325112869605, 1.000000000000000000, 0.9238795325112869605, 1.000000000000000000, 0.9238795325112869605, 1.000000000000000000, 0.9238795325112869605, 1.000000000000000000, 0.9238795325112869605, 1.000000000000000000, 0.9238795325112869605, 1.000000000000000000, 0.9238795325112869605, 1.000000000000000000, 0.9238795325112869605, 1.000000000000000000, 0.9238795325112869605, 1.000000000000000000, 0.9238795325112869605, 1.000000000000000000, 0.9238795325112869605, 1.000000000000000000, 0.9238795325112869605, 1.000000000000000000, 0.9238795325112869605, 1.000000000000000000, 0.9238795325112869605, 1.000000000000000000, 0.9238795325112869605, 1.000000000000000000, 0.9238795325112869605, 1.000000000000000000, 0.9238795325112869605, 1.000000000000000000, 0.9238795325112869605, 1.000000000000000000, 0.9238795325112869605, 1.000000000000000000, 0.9238795325112869605, 1.000000000000000000, 0.9238795325112869605, 1.000000000000000000, 0.9238795325112869605, 1.000000000000000000, 0.9238795325112869605, 1.000000000000000000, 0.9238795325112869605, 1.000000000000000000, 0.9238795325112869605, 1.000000000000000000, 0.9238795325112869605, 1.000000000000000000, 0.9238795325112869605, 1.000000000000000000, 0.9238795325112869605, 1.000000000000000000, 0.9238795325112869605, 1.000000000000000000, 0.9238795325112869605, 1.000000000000000000, 0.9238795325112869605, 1.000000000000000000, 0.9238795325112869605, 1.000000000000000000, 0.9238795325112869605, 1.000000000000000000, 0.9238795325112869605, 1.000000000000000000, 0.9238795325112869605, 1.000000000000000000, 0.9238795325112869605, 1.000000000000000000, 0.9238795325112869605, 1.000000000000000000, 0.9238795325112869605, 1.000000000000000000, 0.9238795325112869605, 1.000000000000000000, 0.9238795325112869605, 1.000000000000000000, 0.9238795325112869605, 1.000000000000000000, 0.9238795325112869605, 1.000000000000000000, 0.9238795325112869605, 1.000000000000000000, 0.9238795325112869605, 1.000000000000000000, 0.9238795325112869605, 1.000000000000000000, 0.9238795325112869605, 1.000000000000000000, 0.9238795325112869605, 1.000000000000000000, 0.9238795325112869605, 1.000000000000000000, 0.9238795325112869605, 1.000000000000000000, 0.9238795325112869605, 1.000000000000000000, 0.9238795325112869605, 1.000000000000000000, 0.9238795325112869605, 1.000000000000000000, 0.9238795325112869605, 1.000000000000000000, 0.9238795325112869605, 1.000000000000000000, 0.9238795325112869605, 1.000000000000000000, 0.9238795325112869605, 1.000000000000000000, 0.9238795325112869605, 1.000000000000000000, 0.9238795325112869605, 1.000000000000000000, 0.9238795325112869605, 1.000000000000000000, 0.9238795325112869605, 1.000000000000000000, 0.9238795325112869605, 1.000000000000000000, 0.9238795325112869605, 1.000000000000000000, 0.9238795325112869605, 1.000000000000000000, 0.9238795325112869605, 1.000000000000000000, 0.9238795325112869605, 1.000000000000000000, 0.9238795325112869605, 1.000000000000000000, 0.9238795325112869605, 1.000000000000000000, 0.9238795325112869605, 1.000000000000000000, 0.9238795325112869605, 1.000000000000000000, 0.9238795325112869605, 1.000000000000000000, 0.9238795325112869605, 1.000000000000000000, 0.9238795325112869605, 1.000000000000000000, 0.9238795325112869605, 1.000000000000000000, 0.9238795325112869605, 1.000000000000000000, 0.9238795325112869605, 1.000000000000000000, 0.9238795325112869605, 1.000000000000000000, 0.9238795325112869605, 1.000000000000000000, 0.9238795325112869605, 1.000000000000000000, 0.9238795325112869605, 1.000000000000000000, 0.9238795325112869605, 1.000000000000000000, 0.9238795325112869605, 1.000000000000000000, 0.9238795325112869605, 1.000000000000000000, 0.9238795325112869605, 1.000000000000000000, 0.9238795325112869605, 1.000000000000000000, 0.9238795325112869605, 1.000000000000000000, 0.9238795325112869605, 1.000000000000000000, 0.9238795325112869605, 1.000000000000000000, 0.9238795325112869605, 1.000000000000000000, 0.9238795325112869605, 1.000000000000000000, 0.9238795325112869605, 1.000000000000000000, 0.9238795325112869605, 1.000000000000000000, 0.9238795325112869605, 1.000000000000000000, 0.9238795325112869605, 1.000000000000000000, 0.9238795325112869605, 1.000000000000000000, 0.9238795325112869605, 1.000000000000000000, 0.9238795325112869605, 1.000000000000000000, 0.9238795325112869605, 1.000000000000000000, 0.9238795325112869605, 1.000000000000000000, 0.9238795325112869605, 1.000000000000000000, 0.9238795325112869605, 1.000000000000000000, 0.9238795325112869605, 1.000000000000000000, 0.9238795325112869605, 1.000000000000000000, 0.9238795325112869605, 1.000000000000000000, 0.9238795325112869605, 1.000000000000000000, 0.9238795325112869605, 1.000000000000000000, 0.9238795325112869605, 1.000000000000000000, 0.9238795325112869605, 1.000000000000000000, 0.9238795325112869605, 1.000000000000000000, 0.9238795325112869605, 1.000000000000000000, 0.9238795325112869605, 1.000000000000000000, 0.9238795325112869605, 1.000000000000000000, 0.9238795325112869605, 1.000000000000000000, 0.9238795325112869605, 1.000000000000000000, 0.9238795325112869605, 1.000000000000000000, 0.9238795325112869605, 1.000000000000000000, 0.9238795325112869605, 1.000000000000000000, 0.9238795325112869605, 1.000000000000000000, 0.9238795325112869605, 1.000000000000000000, 0.9238795325112869605, 1.000000000000000000, 0.9238795325112869605, 1.000000000000000000, 0.9238795325112869605, 1.000000000000000000, 0.9238795325112869605, 1.000000000000000000, 0.9238795325112869605, 1.000000000000000000, 0.9238795325112869605, 1.000000000000000000, 0.9238795325112869605, 1.000000000000000000, 0.9238795325112869605, 1.000000000000000000, 0.9238795325112869605, 1.000000000000000000, 0.9238795325112869605, 1.000000000000000000, 0.9238795325112869605, 1.000000000000000000, 0.9238795325112869605, 1.000000000000000000, 0.9238795325112869605, 1.000000000000000000, 0.9238795325112869605, 1.000000000000000000, 0.9238795325112869605, 1.000000000000000000, 0.9238795325112869605, 1.000000000000000000, 0.9238795325112869605, 1.000000000000000000, 0.9238795325112869605, 1.000000000000000000, 0.9238795325112869605, 1.000000000000000000, 0.9238795325112869605, 1.000000000000000000, 0.9238795325112869605, 1.000000000000000000, 0.9238795325112869605, 1.000000000000000000, 0.9238795325112869605, 1.000000000000000000, 0.9238795325112869605, 1.000000000000000000, 0.9238795325112869605, 1.000000000000000000, 0.9238795325112869605, 1.000000000000000000, 0.9238795325112869605, 1.000000000000000000, 0.9238795325112869605, 1.000000000000000000, 0.9238795325112869605, 1.000000000000000000, 0.9238795325112869605, 1.000000000000000000, 0.9238795325112869605, 1.000000000000000000, 0.9238795325112869605, 1.000000000000000000, 0.9238795325112869605, 1.000000000000000000, 0.9238795325112869605, 1.000000000000000000, 0.9238795325112869605, 1.000000000000000000, 0.9238795325112869605, 1.000000000000000000, 0.9238795325112869605, 1.000000000000000000, 0.9238795325112869605, 1.000000000000000000, 0.9238795325112869605, 1.000000000000000000, 0.9238795325112869605, 1.000000000000000000, 0.9238795325112869605, 1.000000000000000000, 0.9238795325112869605, 1.000000000000000000, 0.9238795325112869605, 1.000000000000000000, 0.9238795325112869605, 1.000000000000000000, 0.9238795325112869605, 1.000000000000000000, 0.9238795325112869605, 1.000000000000000000, 0.9238795325112869605, 1.000000000000000000, 0.9238795325112869605, 1.000000000000000000, 0.9238795325112869605, 1.000000000000000000, 0.9238795325112869605, 1.000000000000000000, 0.9238795325112869605, 1.000000000000000000, 0.9238795325112869605, 1.000000000000000000, 0.9238795325112869605, 1.000000000000000000, 0.9238795325112869605, 1.000000000000000000, 0.9238795325112869605, 1.000000000000000000, 0.9238795325112869605, 1.000000000000000000, 0.9238795325112869605, 1.000000000000000000, 0.9238795325112869605, 1.000000000000000000, 0.9238795325112869605, 1.000000000000000000, 0.9238795325112869605, 1.000000000000000000, 0.9238795325112869605, 1.000000000000000000, 0.9238795325112869605, 1.000000000000000000, 0.9238795325112869605, 1.000000000000000000, 0.9238795325112869605, 1.000000000000000000, 0.9238795325112869605, 1.000000000000000000, 0.9238795325112869605, 1.000000000000000000, 0.9238795325112869605, 1.000000000000000000, 0.9238795325112869605, 1.000000000000000000, 0.9238795325112869605, 1.000000000000000000, 0.9238795325112869605, 1.000000000000000000, 0.9238795325112869605, 1.000000000000000000, 0.9238795325112869605, 1.000000000000000000, 0.9238795325112869605, 1.000000000000000000, 0.9238795325112869605, 1.000000000000000000, 0.9238795325112869605, 1.000000000000000000, 0.9238795325112869605, 1.000000000000000000, 0.9238795325112869605, 1.000000000000000000, 0.9238795325112869605, 1.000000000000000000, 0.9238795325112869605, 1.000000000000000000, 0.9238795325112869605, 1.000000000000000000, 0.9238795325112869605, 1.000000000000000000, 0.9238795325112869605, 1.000000000000000000, 0.9238795325112869605, 1.000000000000000000, 0.9238795325112869605, 1.000000000000000000, 0.9238795325112869605, 1.000000000000000000, 0.9238795325112869605, 1.000000000000000000, 0.9238795325112869605, 1.000000000000000000, 0.9238795325112869605, 1.000000000000000000, 0.9238795325112869605, 1.000000000000000000, 0.9238795325112869605, 1.000000000000000000, 0.9238795325112869605, 1.000000000000000000, 0.9238795325112869605, 1.000000000000000000, 0.9238795325112869605, 1.000000000000000000, 0.9238795325112869605, 1.000000000000000000, 0.9238795325112869605, 1.000000000000000000, 0.9238795325112869605, 1.000000000000000000, 0.9238795325112869605, 1.000000000000000000, 0.9238795325112869605, 1.000000000000000000, 0.9238795325112869605, 1.000000000000000000, 0.9238795325112869605, 1.000000000000000000, 0.9238795325112869605, 1.000000000000000000, 0.9238795325112869605, 1.000000000000000000, 0.9238795325112869605, 1.000000000000000000, 0.9238795325112869605, 1.000000000000000000, 0.9238795325112869605, 1.000000000000000000, 0.9238795325112869605, 1.000000000000000000, 0.9238795325112869605, 1.000000000000000000, 0.9238795325112869605, 1.000000000000000000, 0.9238795325112869605, 1.000000000000000000, 0.9238795325112869605, 1.000000000000000000, 0.9238795325112869605, 1.000000000000000000, 0.9238795325112869605, 1.000000000000000000, 0.9238795325112869605, 1.000000000000000000, 0.9238795325112869605, 1.000000000000000000, 0.9238795325112869605, 1.000000000000000000, 0.9238795325112869605, 1.000000000000000000, 0.9238795325112869605, 1.000000000000000000, 0.9238795325112869605, 1.000000000000000000, 0.9238795325112869605, 1.000000000000000000, 0.9238795325112869605, 1.000000000000000000, 0.9238795325112869605, 1.000000000000000000, 0.9238795325112869605, 1.000000000000000000, 0.9238795325112869605, 1.000000000000000000),
 ( 1.000000000000000000, 0.9238795325112869605, 1.000000000000000000, 0.9238795325112869605, 1.000000000000000000, 0.9238795325112869605, 1.000000000000000000, 0.9238795325112869605, 1.000000000000000000, 0.9238795325112869605, 1.000000000000000000, 0.9238795325112869605, 1.000000000000000000, 0.9238795325112869605, 1.000000000000000000, 0.9238795325112869605, 1.000000000000000000, 0.9238795325112869605, 1.000000000000000000, 0.9238795325112869605, 1.000000000000000000, 0.9238795325112869605, 1.000000000000000000, 0.9238795325112869605, 1.000000000000000000, 0.9238795325112869605, 1.000000000000000000, 0.9238795325112869605, 1.000000000000000000, 0.9238795325112869605, 1.000000000000000000, 0.9238795325112869605, 1.000000000000000000, 0.9238795325112869605, 1.000000000000000000, 0.9238795325112869605, 1.000000000000000000, 0.9238795325112869605, 1.000000000000000000, 0.9238795325112869605, 1.000000000000000000, 0.9238795325112869605, 1.000000000000000000, 0.9238795325112869605, 1.000000000000000000, 0.9238795325112869605, 1.000000000000000000, 0.9238795325112869605, 1.000000000000000000, 0.9238795325112869605, 1.000000000000000000, 0.9238795325112869605, 1.000000000000000000, 0.9238795325112869605, 1.000000000000000000, 0.9238795325112869605, 1.000000000000000000, 0.9238795325112869605, 1.000000000000000000, 0.9238795325112869605, 1.000000000000000000, 0.9238795325112869605, 1.000000000000000000, 0.9238795325112869605, 1.000000000000000000, 0.9238795325112869605, 1.000000000000000000, 0.9238795325112869605, 1.000000000000000000, 0.9238795325112869605, 1.000000000000000000, 0.9238795325112869605, 1.000000000000000000, 0.9238795325112869605, 1.000000000000000000, 0.9238795325112869605, 1.000000000000000000, 0.9238795325112869605, 1.000000000000000000, 0.9238795325112869605, 1.000000000000000000, 0.9238795325112869605, 1.000000000000000000, 0.9238795325112869605, 1.000000000000000000, 0.9238795325112869605, 1.000000000000000000, 0.9238795325112869605, 1.000000000000000000, 0.9238795325112869605, 1.000000000000000000, 0.9238795325112869605, 1.000000000000000000, 0.9238795325112869605, 1.000000000000000000, 0.9238795325112869605, 1.000000000000000000, 0.9238795325112869605, 1.000000000000000000, 0.9238795325112869605, 1.000000000000000000, 0.9238795325112869605, 1.000000000000000000, 0.9238795325112869605, 1.000000000000000000, 0.9238795325112869605, 1.000000000000000000, 0.9238795325112869605, 1.000000000000000000, 0.9238795325112869605, 1.000000000000000000, 0.9238795325112869605, 1.000000000000000000, 0.9238795325112869605, 1.000000000000000000, 0.9238795325112869605, 1.000000000000000000, 0.9238795325112869605, 1.000000000000000000, 0.9238795325112869605, 1.000000000000000000, 0.9238795325112869605, 1.000000000000000000, 0.9238795325112869605, 1.000000000000000000, 0.9238795325112869605, 1.000000000000000000, 0.9238795325112869605, 1.000000000000000000, 0.9238795325112869605, 1.000000000000000000, 0.9238795325112869605, 1.000000000000000000, 0.9238795325112869605, 1.000000000000000000, 0.9238795325112869605, 1.000000000000000000, 0.9238795325112869605, 1.000000000000000000, 0.9238795325112869605, 1.000000000000000000, 0.9238795325112869605, 1.000000000000000000, 0.9238795325112869605, 1.000000000000000000, 0.9238795325112869605, 1.000000000000000000, 0.9238795325112869605, 1.000000000000000000, 0.9238795325112869605, 1.000000000000000000, 0.9238795325112869605, 1.000000000000000000, 0.9238795325112869605, 1.000000000000000000, 0.9238795325112869605, 1.000000000000000000, 0.9238795325112869605, 1.000000000000000000, 0.9238795325112869605, 1.000000000000000000, 0.9238795325112869605, 1.000000000000000000, 0.9238795325112869605, 1.000000000000000000, 0.9238795325112869605, 1.000000000000000000, 0.9238795325112869605, 1.000000000000000000, 0.9238795325112869605, 1.000000000000000000, 0.9238795325112869605, 1.000000000000000000, 0.9238795325112869605, 1.000000000000000000, 0.9238795325112869605, 1.000000000000000000, 0.9238795325112869605, 1.000000000000000000, 0.9238795325112869605, 1.000000000000000000, 0.9238795325112869605, 1.000000000000000000, 0.9238795325112869605, 1.000000000000000000, 0.9238795325112869605, 1.000000000000000000, 0.9238795325112869605, 1.000000000000000000, 0.9238795325112869605, 1.000000000000000000, 0.9238795325112869605, 1.000000000000000000, 0.9238795325112869605, 1.000000000000000000, 0.9238795325112869605, 1.000000000000000000, 0.9238795325112869605, 1.000000000000000000, 0.9238795325112869605, 1.000000000000000000, 0.9238795325112869605, 1.000000000000000000, 0.9238795325112869605, 1.000000000000000000, 0.9238795325112869605, 1.000000000000000000, 0.9238795325112869605, 1.000000000000000000, 0.9238795325112869605, 1.000000000000000000, 0.9238795325112869605, 1.000000000000000000, 0.9238795325112869605, 1.000000000000000000, 0.9238795325112869605, 1.000000000000000000, 0.9238795325112869605, 1.000000000000000000, 0.9238795325112869605, 1.000000000000000000, 0.9238795325112869605, 1.000000000000000000, 0.9238795325112869605, 1.000000000000000000, 0.9238795325112869605, 1.000000000000000000, 0.9238795325112869605, 1.000000000000000000, 0.9238795325112869605, 1.000000000000000000, 0.9238795325112869605, 1.000000000000000000, 0.9238795325112869605, 1.000000000000000000, 0.9238795325112869605, 1.000000000000000000, 0.9238795325112869605, 1.000000000000000000, 0.9238795325112869605, 1.000000000000000000, 0.9238795325112869605, 1.000000000000000000, 0.9238795325112869605, 1.000000000000000000, 0.9238795325112869605, 1.000000000000000000, 0.9238795325112869605, 1.000000000000000000, 0.9238795325112869605, 1.000000000000000000, 0.9238795325112869605, 1.000000000000000000, 0.9238795325112869605, 1.000000000000000000, 0.9238795325112869605, 1.000000000000000000, 0.9238795325112869605, 1.000000000000000000, 0.9238795325112869605, 1.000000000000000000, 0.9238795325112869605, 1.000000000000000000, 0.9238795325112869605, 1.000000000000000000, 0.9238795325112869605, 1.000000000000000000, 0.9238795325112869605, 1.000000000000000000, 0.9238795325112869605, 1.000000000000000000, 0.9238795325112869605, 1.000000000000000000, 0.9238795325112869605, 1.000000000000000000, 0.9238795325112869605, 1.000000000000000000, 0.9238795325112869605, 1.000000000000000000, 0.9238795325112869605, 1.000000000000000000, 0.9238795325112869605, 1.000000000000000000, 0.9238795325112869605, 1.000000000000000000, 0.9238795325112869605, 1.000000000000000000, 0.9238795325112869605, 1.000000000000000000, 0.9238795325112869605, 1.000000000000000000, 0.9238795325112869605, 1.000000000000000000, 0.9238795325112869605, 1.000000000000000000, 0.9238795325112869605, 1.000000000000000000, 0.9238795325112869605, 1.000000000000000000, 0.9238795325112869605, 1.000000000000000000, 0.9238795325112869605, 1.000000000000000000, 0.9238795325112869605, 1.000000000000000000, 0.9238795325112869605, 1.000000000000000000, 0.9238795325112869605, 1.000000000000000000, 0.9238795325112869605, 1.000000000000000000, 0.9238795325112869605, 1.000000000000000000, 0.9238795325112869605, 1.000000000000000000, 0.9238795325112869605, 1.000000000000000000, 0.9238795325112869605, 1.000000000000000000, 0.9238795325112869605, 1.000000000000000000, 0.9238795325112869605, 1.000000000000000000, 0.9238795325112869605, 1.000000000000000000, 0.9238795325112869605, 1.000000000000000000, 0.9238795325112869605, 1.000000000000000000, 0.9238795325112869605, 1.000000000000000000, 0.9238795325112869605, 1.000000000000000000, 0.9238795325112869605, 1.000000000000000000, 0.9238795325112869605, 1.000000000000000000, 0.9238795325112869605, 1.000000000000000000, 0.9238795325112869605, 1.000000000000000000, 0.9238795325112869605, 1.000000000000000000, 0.9238795325112869605, 1.000000000000000000, 0.9238795325112869605, 1.000000000000000000, 0.9238795325112869605, 1.000000000000000000, 0.9238795325112869605, 1.000000000000000000, 0.9238795325112869605, 1.000000000000000000, 0.9238795325112869605, 1.000000000000000000, 0.9238795325112869605, 1.000000000000000000, 0.9238795325112869605, 1.000000000000000000, 0.9238795325112869605, 1.000000000000000000, 0.9238795325112869605, 1.000000000000000000, 0.9238795325112869605, 1.000000000000000000, 0.9238795325112869605, 1.000000000000000000, 0.9238795325112869605, 1.000000000000000000, 0.9238795325112869605, 1.000000000000000000, 0.9238795325112869605, 1.000000000000000000, 0.9238795325112869605, 1.000000000000000000, 0.9238795325112869605, 1.000000000000000000, 0.9238795325112869605, 1.000000000000000000, 0.9238795325112869605, 1.000000000000000000, 0.9238795325112869605, 1.000000000000000000, 0.9238795325112869605, 1.000000000000000000, 0.9238795325112869605, 1.000000000000000000, 0.9238795325112869605, 1.000000000000000000, 0.9238795325112869605, 1.000000000000000000, 0.9238795325112869605, 1.000000000000000000, 0.9238795325112869605, 1.000000000000000000, 0.9238795325112869605, 1.000000000000000000, 0.9238795325112869605, 1.000000000000000000, 0.9238795325112869605, 1.000000000000000000, 0.9238795325112869605, 1.000000000000000000, 0.9238795325112869605, 1.000000000000000000, 0.9238795325112869605, 1.000000000000000000, 0.9238795325112869605, 1.000000000000000000, 0.9238795325112869605, 1.000000000000000000, 0.9238795325112869605, 1.000000000000000000, 0.9238795325112869605, 1.000000000000000000, 0.9238795325112869605, 1.000000000000000000, 0.9238795325112869605, 1.000000000000000000, 0.9238795325112869605, 1.000000000000000000, 0.9238795325112869605, 1.000000000000000000, 0.9238795325112869605, 1.000000000000000000, 0.9238795325112869605, 1.000000000000000000, 0.9238795325112869605, 1.000000000000000000, 0.9238795325112869605, 1.000000000000000000, 0.9238795325112869605, 1.000000000000000000, 0.9238795325112869605, 1.000000000000000000, 0.9238795325112869605, 1.000000000000000000, 0.9238795325112869605, 1.000000000000000000, 0.9238795325112869605, 1.000000000000000000, 0.9238795325112869605, 1.000000000000000000, 0.9238795325112869605, 1.000000000000000000, 0.9238795325112869605, 1.000000000000000000, 0.9238795325112869605, 1.000000000000000000, 0.9238795325112869605, 1.000000000000000000, 0.9238795325112869605, 1.000000000000000000, 0.9238795325112869605, 1.000000000000000000, 0.9238795325112869605, 1.000000000000000000, 0.9238795325112869605, 1.000000000000000000, 0.9238795325112869605, 1.000000000000000000, 0.9238795325112869605, 1.000000000000000000, 0.9238795325112869605, 1.000000000000000000, 0.9238795325112869605, 1.000000000000000000, 0.9238795325112869605, 1.000000000000000000, 0.9238795325112869605, 1.000000000000000000, 0.9238795325112869605, 1.000000000000000000, 0.9238795325112869605, 1.000000000000000000, 0.9238795325112869605, 1.000000000000000000, 0.9238795325112869605, 1.000000000000000000, 0.9238795325112869605, 1.000000000000000000, 0.9238795325112869605, 1.000000000000000000, 0.9238795325112869605, 1.000000000000000000, 0.9238795325112869605, 1.000000000000000000, 0.9238795325112869605, 1.000000000000000000, 0.9238795325112869605, 1.000000000000000000, 0.9238795325112869605, 1.000000000000000000, 0.9238795325112869605, 1.000000000000000000, 0.9238795325112869605, 1.000000000000000000, 0.9238795325112869605, 1.000000000000000000, 0.9238795325112869605, 1.000000000000000000, 0.9238795325112869605, 1.000000000000000000, 0.9238795325112869605, 1.000000000000000000, 0.9238795325112869605, 1.000000000000000000, 0.9238795325112869605, 1.000000000000000000, 0.9238795325112869605, 1.000000000000000000, 0.9238795325112869605, 1.000000000000000000, 0.9238795325112869605, 1.000000000000000000, 0.9238795325112869605, 1.000000000000000000, 0.9238795325112869605, 1.000000000000000000, 0.9238795325112869605, 1.000000000000000000, 0.9238795325112869605, 1.000000000000000000, 0.9238795325112869605, 1.000000000000000000, 0.9238795325112869605, 1.000000000000000000, 0.9238795325112869605, 1.000000000000000000, 0.9238795325112869605, 1.000000000000000000, 0.9238795325112869605, 1.000000000000000000, 0.9238795325112869605, 1.000000000000000000, 0.9238795325112869605, 1.000000000000000000, 0.9238795325112869605, 1.000000000000000000, 0.9238795325112869605, 1.000000000000000000, 0.9238795325112869605, 1.000000000000000000, 0.9238795325112869605, 1.000000000000000000, 0.9238795325112869605, 1.000000000000000000, 0.9238795325112869605, 1.000000000000000000, 0.9238795325112869605, 1.000000000000000000, 0.9238795325112869605, 1.000000000000000000, 0.9238795325112869605, 1.000000000000000000, 0.9238795325112869605, 1.000000000000000000, 0.9238795325112869605, 1.000000000000000000, 0.9238795325112869605, 1.000000000000000000, 0.9238795325112869605, 1.000000000000000000, 0.9238795325112869605, 1.000000000000000000, 0.9238795325112869605, 1.000000000000000000, 0.9238795325112869605, 1.000000000000000000, 0.9238795325112869605, 1.000000000000000000, 0.9238795325112869605, 1.000000000000000000, 0.9238795325112869605, 1.000000000000000000, 0.9238795325112869605, 1.000000000000000000, 0.9238795325112869605, 1.000000000000000000, 0.9238795325112869605, 1.000000000000000000, 0.9238795325112869605, 1.000000000000000000, 0.9238795325112869605, 1.000000000000000000, 0.9238795325112869605, 1.000000000000000000, 0.9238795325112869605, 1.000000000000000000, 0.9238795325112869605, 1.000000000000000000, 0.9238795325112869605, 1.000000000000000000, 0.9238795325112869605, 1.000000000000000000, 0.9238795325112869605, 1.000000000000000000, 0.9238795325112869605, 1.000000000000000000, 0.9238795325112869605, 1.000000000000000000, 0.9238795325112869605, 1.000000000000000000, 0.9238795325112869605, 1.000000000000000000, 0.9238795325112869605, 1.000000000000000000, 0.9238795325112869605, 1.000000000000000000, 0.9238795325112869605, 1.000000000000000000, 0.9238795325112869605, 1.000000000000000000, 0.9238795325112869605, 1.000000000000000000, 0.9238795325112869605, 1.000000000000000000, 0.9238795325112869605, 1.000000000000000000, 0.9238795325112869605, 1.000000000000000000, 0.9238795325112869605, 1.000000000000000000, 0.9238795325112869605, 1.000000000000000000, 0.9238795325112869605, 1.000000000000000000, 0.9238795325112869605, 1.000000000000000000, 0.9238795325112869605, 1.000000000000000000, 0.9238795325112869605, 1.000000000000000000, 0.9238795325112869605, 1.000000000000000000, 0.9238795325112869605, 1.000000000000000000, 0.9238795325112869605, 1.000000000000000000, 0.9238795325112869605, 1.000000000000000000, 0.9238795325112869605, 1.000000000000000000, 0.9238795325112869605, 1.000000000000000000, 0.9238795325112869605, 1.000000000000000000, 0.9238795325112869605, 1.000000000000000000, 0.9238795325112869605, 1.000000000000000000, 0.9238795325112869605, 1.000000000000000000, 0.9238795325112869605, 1.000000000000000000, 0.9238795325112869605, 1.000000000000000000, 0.9238795325112869605, 1.000000000000000000, 0.9238795325112869605, 1.000000000000000000, 0.9238795325112869605, 1.000000000000000000, 0.9238795325112869605, 1.000000000000000000, 0.9238795325112869605, 1.000000000000000000, 0.9238795325112869605, 1.000000000000000000, 0.9238795325112869605, 1.000000000000000000, 0.9238795325112869605, 1.000000000000000000, 0.9238795325112869605, 1.000000000000000000, 0.9238795325112869605, 1.000000000000000000, 0.9238795325112869605, 1.000000000000000000, 0.9238795325112869605, 1.000000000000000000, 0.9238795325112869605, 1.000000000000000000, 0.9238795325112869605, 1.000000000000000000, 0.9238795325112869605, 1.000000000000000000, 0.9238795325112869605, 1.000000000000000000, 0.9238795325112869605, 1.000000000000000000, 0.9238795325112869605, 1.000000000000000000, 0.9238795325112869605, 1.000000000000000000, 0.9238795325112869605, 1.000000000000000000, 0.9238795325112869605, 1.000000000000000000, 0.9238795325112869605, 1.000000000000000000, 0.9238795325112869605, 1.000000000000000000, 0.9238795325112869605, 1.000000000000000000, 0.9238795325112869605, 1.000000000000000000, 0.9238795325112869605, 1.000000000000000000, 0.9238795325112869605, 1.000000000000000000, 0.9238795325112869605, 1.000000000000000000, 0.9238795325112869605, 1.000000000000000000, 0.9238795325112869605, 1.000000000000000000, 0.9238795325112869605, 1.000000000000000000, 0.9238795325112869605, 1.000000000000000000, 0.9238795325112869605, 1.000000000000000000, 0.9238795325112869605, 1.000000000000000000, 0.9238795325112869605, 1.000000000000000000, 0.9238795325112869605, 1.000000000000000000, 0.9238795325112869605, 1.000000000000000000, 0.9238795325112869605, 1.000000000000000000, 0.9238795325112869605, 1.000000000000000000, 0.9238795325112869605, 1.000000000000000000, 0.9238795325112869605, 1.000000000000000000, 0.9238795325112869605, 1.000000000000000000, 0.9238795325112869605, 1.000000000000000000, 0.9238795325112869605, 1.000000000000000000, 0.9238795325112869605, 1.000000000000000000, 0.9238795325112869605, 1.000000000000000000, 0.9238795325112869605, 1.000000000000000000, 0.9238795325112869605, 1.000000000000000000, 0.9238795325112869605, 1.000000000000000000, 0.9238795325112869605, 1.000000000000000000, 0.9238795325112869605, 1.000000000000000000, 0.9238795325112869605, 1.000000000000000000, 0.9238795325112869605, 1.000000000000000000, 0.9238795325112869605, 1.000000000000000000, 0.9238795325112869605, 1.000000000000000000, 0.9238795325112869605, 1.000000000000000000, 0.9238795325112869605, 1.000000000000000000, 0.9238795325112869605, 1.000000000000000000, 0.9238795325112869605, 1.000000000000000000, 0.9238795325112869605, 1.000000000000000000, 0.9238795325112869605, 1.000000000000000000, 0.9238795325112869605, 1.000000000000000000, 0.9238795325112869605, 1.000000000000000000, 0.9238795325112869605, 1.000000000000000000, 0.9238795325112869605, 1.000000000000000000, 0.9238795325112869605, 1.000000000000000000, 0.9238795325112869605, 1.000000000000000000, 0.9238795325112869605, 1.000000000000000000, 0.9238795325112869605, 1.000000000000000000, 0.9238795325112869605, 1.000000000000000000, 0.9238795325112869605, 1.000000000000000000, 0.9238795325112869605, 1.000000000000000000) ) ) 
 REPRESENTATION_ITEM ( '' )  SURFACE ( )  ) ;
#32308=CARTESIAN_POINT ( 'NONE',  ( 0.1797182628040039365, -0.8474847544649350972, -2.200913952912460540E-17 ) ) ;
#32309=CARTESIAN_POINT ( 'NONE',  ( 0.2471922904502826257, 0.07845432542752818483, 0.07637674237069280725 ) ) ;
#32311=CARTESIAN_POINT ( 'NONE',  ( -0.06523048226347956391, -0.6254921259842515235, -0.1574803149606300301 ) ) ;
#32312=CARTESIAN_POINT ( 'NONE',  ( -0.1596844025337534889, 0.1273093748619712751, 0.04123610460087424184 ) ) ;
#32318=CARTESIAN_POINT ( 'NONE',  ( -0.1574803149606297803, -0.6451771652468047957, 0.06523048226347956391 ) ) ;
#32322=CARTESIAN_POINT ( 'NONE',  ( -1.094772975963752103E-17, -0.6402559054580471143, -0.1787899950787401882 ) ) ;
#32330=CARTESIAN_POINT ( 'NONE',  ( 0.1797182628040039087, 0.09985776522010414435, -0.07444174185955065859 ) ) ;
#32331=CARTESIAN_POINT ( 'NONE',  ( -0.1264236179284866091, -1.073326771599779628, -0.1264236179284866091 ) ) ;
#32332=CARTESIAN_POINT ( 'NONE',  ( -0.06523048226347956391, -1.452263779527559251, -0.1574803149606300301 ) ) ;
#32350=CARTESIAN_POINT ( 'NONE',  ( -0.1787899950787401604, -0.2944153068119157446, -0.07405724077823318263 ) ) ;
#32351=CARTESIAN_POINT ( 'NONE',  ( -0.1344623199169003858, -0.09842519685039370636, -0.1216788222333031466 ) ) ;
#32362=CARTESIAN_POINT ( 'NONE',  ( -1.094772975963752103E-17, -1.196358267662771757, -0.1787899950787401882 ) ) ;
#32364=CARTESIAN_POINT ( 'NONE',  ( -0.07405724077823318263, -1.346456692859623550, -0.1787899950787401604 ) ) ;
#32369=CARTESIAN_POINT ( 'NONE',  ( 2.892866454678787531E-17, -0.2145669291338582751, 0.1574803149606299191 ) ) ;
#32380=CARTESIAN_POINT ( 'NONE',  ( -0.1264236179284866091, -0.07431102356828367395, 0.1264236179284866091 ) ) ;
#32382=CARTESIAN_POINT ( 'NONE',  ( -0.1574803149606297803, -1.471948818790110636, 0.06523048226347956391 ) ) ;
#32383=CARTESIAN_POINT ( 'NONE',  ( 0.07405724077823318263, -0.5836614172690718361, 0.1787899950787401604 ) ) ;
#32384=CARTESIAN_POINT ( 'NONE',  ( -0.1113553986120547346, -1.095472440944881942, -0.1113553986120547346 ) ) ;
#32403=CARTESIAN_POINT ( 'NONE',  ( -0.06523048226347956391, -0.2465551180027093781, 0.1574803149606297803 ) ) ;
#32412=CARTESIAN_POINT ( 'NONE',  ( 0.1264236179284866091, -1.724041291063883818, -0.1264236179284866091 ) ) ;
#32417=CARTESIAN_POINT ( 'NONE',  ( -0.1264236179284866091, -0.4040354330171023745, -0.1264236179284866091 ) ) ;
#32418=CARTESIAN_POINT ( 'NONE',  ( 0.1264236179284866091, -0.8912401574265511606, 0.1264236179284866091 ) ) ;
#32420=CARTESIAN_POINT ( 'NONE',  ( -0.2471918495545273875, -0.09442133267706703803, -0.03395794428076703841 ) ) ;
#32424=CARTESIAN_POINT ( 'NONE',  ( 0.07405724077823318263, -0.06803735405601045449, -0.1787899950787401604 ) ) ;
#32425=CARTESIAN_POINT ( 'NONE',  ( -0.1264236179284866091, 0.02903543312462964626, -0.1264236179284866091 ) ) ;
#32426=CARTESIAN_POINT ( 'NONE',  ( 0.2471922279627869479, -0.07692167320570084121, -0.07932652958025969425 ) ) ;
#32432=CARTESIAN_POINT ( 'NONE',  ( -0.1797182628040039087, -1.730850896197219768, 0.07444174185955065859 ) ) ;
#32433=CARTESIAN_POINT ( 'NONE',  ( 0.1264236179284866091, -0.4483267715997795166, -0.1264236179284866091 ) ) ;
#32442=CARTESIAN_POINT ( 'NONE',  ( 3.284318927891251994E-17, -0.1136811023084411398, 0.1787899950787401882 ) ) ;
#32445=CARTESIAN_POINT ( 'NONE',  ( -0.07405724077823318263, -1.031496062938363822, -0.1787899950787401604 ) ) ;
#32467=CARTESIAN_POINT ( 'NONE',  ( 3.284318927891251994E-17, -0.07431102356828367395, 0.1787899950787401882 ) ) ;
#32473=CARTESIAN_POINT ( 'NONE',  ( 0.1787899950787401882, -1.295891684764671314, -2.189545951927503898E-17 ) ) ;
#32475=CARTESIAN_POINT ( 'NONE',  ( -0.1264236179284866091, -0.2810039369541106336, -0.1264236179284866091 ) ) ;
#32479=CARTESIAN_POINT ( 'NONE',  ( -0.2471922763370260623, -0.09254788073167596885, 0.04110581524695881839 ) ) ;
#32482=CARTESIAN_POINT ( 'NONE',  ( 0.1264236179284866091, -1.634350393647023614, -0.1264236179284866091 ) ) ;
#32483=CARTESIAN_POINT ( 'NONE',  ( -0.1264236179284866091, -0.7091535432533228045, 0.1264236179284866091 ) ) ;
#32486=CARTESIAN_POINT ( 'NONE',  ( 0.1270800023317771588, -1.246106801709029321, 0.1270800023317771588 ) ) ;
#32491=CARTESIAN_POINT ( 'NONE',  ( 0.01628405332009578987, 0.1299212598425197041, 0.1749064654736346147 ) ) ;
#32509=CARTESIAN_POINT ( 'NONE',  ( 0.1264236179284866091, -0.09399606293836260118, -0.1264236179284866091 ) ) ;
#32514=CARTESIAN_POINT ( 'NONE',  ( 0.1478661631962259748, -0.09575019180978999733, -0.2000608872901662172 ) ) ;
#32518=CARTESIAN_POINT ( 'NONE',  ( 3.284318927891251994E-17, -1.806594488135212728, 0.1787899950787401882 ) ) ;
#32526=DIRECTION ( 'NONE',  ( 0.000000000000000000, -1.000000000000000000, 0.000000000000000000 ) ) ;
#32527=CARTESIAN_POINT ( 'NONE',  ( 0.1787899950787401882, -0.7840806611426240913, -2.189545951927503898E-17 ) ) ;
#32529=CARTESIAN_POINT ( 'NONE',  ( -0.04541781944810669575, -0.08956206178171143006, 0.1491237657763354596 ) ) ;
#32530=CONICAL_SURFACE ( 'NONE', #2621, 0.2471922904502826812, 0.5235987755982992597 ) ;
#32546=CARTESIAN_POINT ( 'NONE',  ( -0.1797182628040039087, -0.9040792426539112636, 0.07444174185955065859 ) ) ;
#32550=EDGE_CURVE ( 'NONE', #38566, #36909, #20756, .T. ) ;
#32551=CARTESIAN_POINT ( 'NONE',  ( 0.1113553986120547346, -0.6033464566929134243, 0.1113553986120547346 ) ) ;
#32552=CARTESIAN_POINT ( 'NONE',  ( -0.1017260139368336425, 0.1228220809759916765, -0.1240740172185132717 ) ) ;
#32562=CARTESIAN_POINT ( 'NONE',  ( 0.1264236179284866091, -0.6550196849856062542, 0.1264236179284866091 ) ) ;
#32572=CARTESIAN_POINT ( 'NONE',  ( -1.094772975963752103E-17, -1.235728346402928945, -0.1787899950787401882 ) ) ;
#32573=CARTESIAN_POINT ( 'NONE',  ( -0.1113553986120547346, -1.567913385826771755, -0.1113553986120547346 ) ) ;
#32584=CARTESIAN_POINT ( 'NONE',  ( -0.2471922904502826812, 0.09842519685039370636, 5.914624404477007554E-17 ) ) ;
#32587=CARTESIAN_POINT ( 'NONE',  ( -0.1673939672668370293, -0.09842519685039370636, -0.05722842092486787879 ) ) ;
#32599=CARTESIAN_POINT ( 'NONE',  ( 0.1264236179284866091, -1.211122047190330786, 0.1264236179284866091 ) ) ;
#32600=CARTESIAN_POINT ( 'NONE',  ( 0.07405724077823318263, -1.351377952702143004, -0.1787899950787401604 ) ) ;
#32608=CARTESIAN_POINT ( 'NONE',  ( 0.06523048226347956391, -0.07923228346456692717, -0.1574803149606300301 ) ) ;
#32621=CARTESIAN_POINT ( 'NONE',  ( -9.642888182262618425E-18, -1.484251968396409493, -0.1574803149606299191 ) ) ;
#32622=CARTESIAN_POINT ( 'NONE',  ( -0.07405724077823318263, -0.7066929133320629663, 0.1787899950787401604 ) ) ;
#32624=CARTESIAN_POINT ( 'NONE',  ( 0.06523048226347956391, -1.063484251968504379, -0.1574803149606300301 ) ) ;
#32641=CARTESIAN_POINT ( 'NONE',  ( -0.1574803149606300301, -0.1776574802074335768, -0.06523048226347956391 ) ) ;
#32647=CARTESIAN_POINT ( 'NONE',  ( -0.1730591442732248297, -0.09851383842017420733, 0.004658872311817456938 ) ) ;
#32651=CARTESIAN_POINT ( 'NONE',  ( 0.1787899950787401604, -0.6870078739619840391, -0.07405724077823318263 ) ) ;
#32652=DIRECTION ( 'NONE',  ( 0.000000000000000000, 0.000000000000000000, 1.000000000000000000 ) ) ;
#32655=CARTESIAN_POINT ( 'NONE',  ( 0.2471922904502826812, 0.09842519685039370636, -5.914624404477007554E-17 ) ) ;
#32656=CARTESIAN_POINT ( 'NONE',  ( 3.284318927891251994E-17, -0.9749015747493857686, 0.1787899950787401882 ) ) ;
#32658=CARTESIAN_POINT ( 'NONE',  ( -0.2471911544650258752, -0.08539615244838703878, -0.06152421978380465811 ) ) ;
#32661=CARTESIAN_POINT ( 'NONE',  ( -0.07444174185955065859, -0.1511264867483998187, 0.1797182628040039087 ) ) ;
#32662=CARTESIAN_POINT ( 'NONE',  ( 0.07405724077823318263, -0.1467775115363254557, -0.1787899950787401604 ) ) ;
#32663=CARTESIAN_POINT ( 'NONE',  ( 0.1264236179284866091, -0.2514763778989925203, -0.1264236179284866091 ) ) ;
#32668=CARTESIAN_POINT ( 'NONE',  ( -0.1797182628040039365, -1.654571368638163342, 0.000000000000000000 ) ) ;
#32676=CARTESIAN_POINT ( 'NONE',  ( 0.1113553986120547346, -0.8986220471365670148, -0.1113553986120547346 ) ) ;
#32677=CARTESIAN_POINT ( 'NONE',  ( 0.1787899950787401882, -0.3006889763241893943, -2.189545951927503898E-17 ) ) ;
#32680=CARTESIAN_POINT ( 'NONE',  ( 0.07405724077823318263, -1.036417322780882833, -0.1787899950787401604 ) ) ;
#32699=CARTESIAN_POINT ( 'NONE',  ( -0.1787899950787401604, -0.04724409443442544737, -0.07405724077823318263 ) ) ;
#32706=CARTESIAN_POINT ( 'NONE',  ( -0.1264236179284866091, -1.281127905237112286, -0.1264236179284866091 ) ) ;
#32708=CARTESIAN_POINT ( 'NONE',  ( -0.1787899950787401604, -0.2342519684501733479, 0.07405724077823318263 ) ) ;
#32718=CARTESIAN_POINT ( 'NONE',  ( -0.1264236179284866091, -1.663877952702141672, -0.1264236179284866091 ) ) ;
#32719=CARTESIAN_POINT ( 'NONE',  ( -0.1264236179284866091, -0.7583661416785196785, -0.1264236179284866091 ) ) ;
#32723=CARTESIAN_POINT ( 'NONE',  ( -0.07444174185955065859, -1.268252471000367976, -0.1797182628040039087 ) ) ;
#32747=CARTESIAN_POINT ( 'NONE',  ( -0.07405724077823318263, 0.006889763833291078637, 0.1787899950787401604 ) ) ;
#32750=CARTESIAN_POINT ( 'NONE',  ( -0.1235961452251415349, -0.09842519685039370636, -0.2140748031496062798 ) ) ;
#32756=ORIENTED_EDGE ( 'NONE', *, *, #19047, .T. ) ;
#32757=CARTESIAN_POINT ( 'NONE',  ( 2.892866454678787531E-17, 0.07086614183981043702, 0.1574803149606299191 ) ) ;
#32766=CARTESIAN_POINT ( 'NONE',  ( 0.07405724077823318263, -0.8554389288591597307, -0.1787899950787401604 ) ) ;
#32768=CARTESIAN_POINT ( 'NONE',  ( -9.642888182262618425E-18, -0.02755905501058318954, -0.1574803149606299191 ) ) ;
#32770=EDGE_CURVE ( 'NONE', #34774, #2394, #11463, .T. ) ;
#32781=CARTESIAN_POINT ( 'NONE',  ( 0.1797182628040039087, -0.8843942032838323364, -0.07444174185955065859 ) ) ;
#32785=CARTESIAN_POINT ( 'NONE',  ( -0.1113553986120547346, -0.6131889763779527769, 0.1113553986120547346 ) ) ;
#32794=CARTESIAN_POINT ( 'NONE',  ( 0.1787899950787401604, -0.6870078739619840391, -0.07405724077823318263 ) ) ;
#32801=CARTESIAN_POINT ( 'NONE',  ( 0.1264236179284866091, -1.171751968450173154, 0.1264236179284866091 ) ) ;
#32802=CARTESIAN_POINT ( 'NONE',  ( -0.1574803149606297803, -1.521161417322834497, 0.06523048226347956391 ) ) ;
#32807=CARTESIAN_POINT ( 'NONE',  ( -0.1574803149606297803, -0.3302165353255438474, 0.06523048226347956391 ) ) ;
#32808=CARTESIAN_POINT ( 'NONE',  ( -0.07405724077823318263, -1.430118110182456714, -0.1787899950787401604 ) ) ;
#32814=EDGE_CURVE ( 'NONE', #39269, #46651, #28235, .T. ) ;
#32815=CARTESIAN_POINT ( 'NONE',  ( -0.2471922904502826812, 0.07746962187842153236, 0.07828042841527922679 ) ) ;
#32819=CARTESIAN_POINT ( 'NONE',  ( 0.1787899950787401604, -0.3879192438197899273, -0.07405724077823318263 ) ) ;
#32820=CARTESIAN_POINT ( 'NONE',  ( -0.1407286617981055310, -0.09842519685039370636, -0.1134193063733844598 ) ) ;
#32826=EDGE_LOOP ( 'NONE', ( #34277, #23018, #30059, #21204 ) ) ;
#32830=CARTESIAN_POINT ( 'NONE',  ( 0.1787899950787401604, -1.208661417269070393, 0.07405724077823318263 ) ) ;
#32831=CARTESIAN_POINT ( 'NONE',  ( -1.094772975963752103E-17, -1.427657480261196987, -0.1787899950787401882 ) ) ;
#32836=CARTESIAN_POINT ( 'NONE',  ( 0.1797182628040039087, -0.6137249119452504731, 0.07444174185955046430 ) ) ;
#32840=CARTESIAN_POINT ( 'NONE',  ( 0.1113553986120547346, -0.09153543307086613179, 0.1113553986120547346 ) ) ;
#32853=CARTESIAN_POINT ( 'NONE',  ( -0.1574803149606299191, 0.1003937008949285503, 0.000000000000000000 ) ) ;
#32854=CARTESIAN_POINT ( 'NONE',  ( 0.1787899950787401882, -1.634350393647023614, -2.189545951927503898E-17 ) ) ;
#32855=CARTESIAN_POINT ( 'NONE',  ( -0.1574803149606300301, -1.476870078632629868, -0.06523048226347956391 ) ) ;
#32856=CARTESIAN_POINT ( 'NONE',  ( 0.1264236179284866091, -0.7288385826234015097, -0.1264236179284866091 ) ) ;
#32858=CARTESIAN_POINT ( 'NONE',  ( 0.1113553986120547346, -1.026574803149606474, -0.1113553986120547346 ) ) ;
#32866=CARTESIAN_POINT ( 'NONE',  ( -0.1113553986120547346, -1.321850393593259732, -0.1113553986120547346 ) ) ;
#32880=CARTESIAN_POINT ( 'NONE',  ( 0.1188652514094255819, -0.09851384370095650489, -0.1576607626576320975 ) ) ;
#32889=CARTESIAN_POINT ( 'NONE',  ( -0.07405724077823318263, -0.9133858267178897039, -0.1787899950787401604 ) ) ;
#32894=CARTESIAN_POINT ( 'NONE',  ( -0.1270800023317771588, -0.2323272741499747829, 0.1270800023317771588 ) ) ;
#32895=CARTESIAN_POINT ( 'NONE',  ( -0.1264236179284866091, -0.1689231808276639435, 0.1264236179284866091 ) ) ;
#32896=CARTESIAN_POINT ( 'NONE',  ( 0.07405724077823318263, -0.3031496062454492879, 0.1787899950787401604 ) ) ;
#32897=CARTESIAN_POINT ( 'NONE',  ( -0.1787899950787401604, -0.08661417317458304510, -0.07405724077823318263 ) ) ;
#32898=CARTESIAN_POINT ( 'NONE',  ( 0.2471883443658805524, -0.06218794471796348922, -0.1039611462658963509 ) ) ;
#32905=CARTESIAN_POINT ( 'NONE',  ( -0.07405724077823318263, -0.4655511810485986057, 0.1787899950787401604 ) ) ;
#32908=CARTESIAN_POINT ( 'NONE',  ( -0.1528784791658471254, -0.09445537554013620773, 0.1971681403758093198 ) ) ;
#32911=CARTESIAN_POINT ( 'NONE',  ( 0.1787899950787401882, -0.3400590550643468601, -2.189545951927503898E-17 ) ) ;
#32915=CARTESIAN_POINT ( 'NONE',  ( 0.1264236179284866091, -1.127460629867496067, 0.1264236179284866091 ) ) ;
#32924=CARTESIAN_POINT ( 'NONE',  ( 0.06523048226347956391, -1.132381889656252527, -0.1574803149606300301 ) ) ;
#32934=CARTESIAN_POINT ( 'NONE',  ( 3.284318927891251994E-17, 0.04379921265218874454, 0.1787899950787401882 ) ) ;
#32939=EDGE_CURVE ( 'NONE', #36616, #36603, #12566, .T. ) ;
#32943=CARTESIAN_POINT ( 'NONE',  ( 3.284318927891251994E-17, -1.305734204449710889, 0.1787899950787401882 ) ) ;
#32944=EDGE_LOOP ( 'NONE', ( #20384, #35526, #31694 ) ) ;
#32945=CARTESIAN_POINT ( 'NONE',  ( -0.1787899950787401882, -0.3154527558517483676, 0.000000000000000000 ) ) ;
#32953=CARTESIAN_POINT ( 'NONE',  ( 0.1787899950787401604, -1.636811023568283341, -0.07405724077823318263 ) ) ;
#32956=CARTESIAN_POINT ( 'NONE',  ( -0.07444174185955065859, -1.425732785961000282, -0.1797182628040039087 ) ) ;
#32964=CARTESIAN_POINT ( 'NONE',  ( -0.1113553986120547346, -0.7608267715460158565, 0.1113553986120547346 ) ) ;
#32965=CARTESIAN_POINT ( 'NONE',  ( 0.07405724077823318263, 0.1250000000537635492, 0.1787899950787401604 ) ) ;
#32970=AXIS2_PLACEMENT_3D ( 'NONE', #30440, #43891, #3875 ) ;
#32979=AXIS2_PLACEMENT_3D ( 'NONE', #30793, #1754, #16397 ) ;
#32985=CARTESIAN_POINT ( 'NONE',  ( 0.1264236179284866091, -0.2121062991588350544, -0.1264236179284866091 ) ) ;
#32994=CARTESIAN_POINT ( 'NONE',  ( 0.1113553986120547346, 0.07578740168233012720, 0.1113553986120547346 ) ) ;
#33003=CARTESIAN_POINT ( 'NONE',  ( -0.07405724077823318263, -0.7570137320087666488, 0.1787899950787401604 ) ) ;
#33016=CARTESIAN_POINT ( 'NONE',  ( 0.1797182628040039087, -0.8499453843861957125, 0.07444174185955046430 ) ) ;
#33029=CARTESIAN_POINT ( 'NONE',  ( 0.1264236179284866091, -0.8026574802611967652, -0.1264236179284866091 ) ) ;
#33031=( BOUNDED_CURVE ( )  B_SPLINE_CURVE ( 2, ( #31313, #13104, #27735, #41566, #19790, #31083, #30389, #42300, #45648, #19557, #24117, #37780, #30612, #15755, #38010, #34423, #44936, #45177, #5404, #33971, #26772, #1097, #41331, #1570, #12149, #8532, #8772, #30853, #12866, #4934, #42049, #20026, #12397, #23407, #14023, #17140, #21435, #31551, #25286, #20957, #10440, #35603, #13328, #10197, #2742, #17370, #13547, #32007, #35831, #46599, #28423, #24344, #6584, #3219, #39875, #38941, #2977, #6105, #20731, #17610, #43237, #46367, #28184, #32256, #29034, #36436, #42241, #14149, #10563, #43834, #35082, #36199, #24933, #36659, #38667, #5836, #16849, #31490, #17963, #13276, #25165, #17730, #9677, #39751, #32380, #6941, #14386, #20036, #23175, #35147, #12409, #9264, #46142, #27967, #20271 ),
 .UNSPECIFIED., .F., .T. ) 
 B_SPLINE_CURVE_WITH_KNOTS ( ( 3, 2, 2, 2, 2, 2, 2, 2, 2, 2, 2, 2, 2, 2, 2, 2, 2, 2, 2, 2, 2, 2, 2, 2, 2, 2, 2, 2, 2, 2, 2, 2, 2, 2, 2, 2, 2, 2, 2, 2, 2, 2, 2, 2, 2, 2, 2, 3 ),
 ( 0.01375000002627235936, 0.01499999999999999944, 0.01750000000000000167, 0.02000000000000000042, 0.02249999999999999917, 0.02500000000000000139, 0.02750000000000000014, 0.02999999999999999889, 0.03250000000000000111, 0.03500000000000000333, 0.03749999999999999861, 0.04000000000000000083, 0.04250000000000000305, 0.04499999999999999833, 0.04750000000000000056, 0.05000000000000000278, 0.05249999999999999806, 0.05500000000000000028, 0.05750000000000000250, 0.05999999999999999778, 0.06250000000000000000, 0.06500000000000000222, 0.06750000000000000444, 0.07000000000000000666, 0.07249999999999999500, 0.07499999999999999722, 0.07749999999999999944, 0.08000000000000000167, 0.08250000000000000389, 0.08500000000000000611, 0.08749999999999999445, 0.08999999999999999667, 0.09250000000000001277, 0.09500000000000000111, 0.09750000000000000333, 0.1000000000000000056, 0.1024999999999999939, 0.1050000000000000100, 0.1074999999999999983, 0.1100000000000000006, 0.1125000000000000028, 0.1150000000000000050, 0.1174999999999999933, 0.1199999999999999956, 0.1224999999999999978, 0.1250000000000000000, 0.1275000000000000022, 0.1297356019617244005 ),
 .UNSPECIFIED. ) 
 CURVE ( )  GEOMETRIC_REPRESENTATION_ITEM ( )  RATIONAL_B_SPLINE_CURVE ( ( 0.9619397662556429252, 0.9619397670555889235, 1.000000000000000000, 0.9238795325112869605, 1.000000000000000000, 0.9238795325112869605, 1.000000000000000000, 0.9238795325112869605, 1.000000000000000000, 0.9238795325112869605, 1.000000000000000000, 0.9238795325112869605, 1.000000000000000000, 0.9238795325112869605, 1.000000000000000000, 0.9238795325112869605, 1.000000000000000000, 0.9238795325112869605, 1.000000000000000000, 0.9238795325112869605, 1.000000000000000000, 0.9238795325112869605, 1.000000000000000000, 0.9238795325112869605, 1.000000000000000000, 0.9238795325112869605, 1.000000000000000000, 0.9238795325112869605, 1.000000000000000000, 0.9238795325112869605, 1.000000000000000000, 0.9238795325112869605, 1.000000000000000000, 0.9238795325112869605, 1.000000000000000000, 0.9238795325112869605, 1.000000000000000000, 0.9238795325112869605, 1.000000000000000000, 0.9238795325112869605, 1.000000000000000000, 0.9238795325112869605, 1.000000000000000000, 0.9238795325112869605, 1.000000000000000000, 0.9238795325112869605, 1.000000000000000000, 0.9238795325112869605, 1.000000000000000000, 0.9238795325112869605, 1.000000000000000000, 0.9238795325112869605, 1.000000000000000000, 0.9238795325112869605, 1.000000000000000000, 0.9238795325112869605, 1.000000000000000000, 0.9238795325112869605, 1.000000000000000000, 0.9238795325112869605, 1.000000000000000000, 0.9238795325112869605, 1.000000000000000000, 0.9238795325112869605, 1.000000000000000000, 0.9238795325112869605, 1.000000000000000000, 0.9238795325112869605, 1.000000000000000000, 0.9238795325112869605, 1.000000000000000000, 0.9238795325112869605, 1.000000000000000000, 0.9238795325112869605, 1.000000000000000000, 0.9238795325112869605, 1.000000000000000000, 0.9238795325112869605, 1.000000000000000000, 0.9238795325112869605, 1.000000000000000000, 0.9238795325112869605, 1.000000000000000000, 0.9238795325112869605, 1.000000000000000000, 0.9238795325112869605, 1.000000000000000000, 0.9238795325112869605, 1.000000000000000000, 0.9238795325112869605, 1.000000000000000000, 0.9238795325112869605, 1.000000000000000000, 0.9319299734219380626, 0.9856019348059209539 ) ) 
 REPRESENTATION_ITEM ( '' )  ) ;
#33037=CARTESIAN_POINT ( 'NONE',  ( -0.1574803149606300301, -1.604822834645670104, -0.06523048226347956391 ) ) ;
#33044=CARTESIAN_POINT ( 'NONE',  ( -0.06523048226347956391, -0.3006889762704259006, -0.1574803149606300301 ) ) ;
#33045=CARTESIAN_POINT ( 'NONE',  ( -1.094772975963752103E-17, -1.432578740103716664, -0.1787899950787401882 ) ) ;
#33055=CARTESIAN_POINT ( 'NONE',  ( 0.08438807215046524590, -0.09131796649090889728, -0.2367113086200097749 ) ) ;
#33058=CARTESIAN_POINT ( 'NONE',  ( -0.1787899950787401882, -0.3706948343709712823, 0.000000000000000000 ) ) ;
#33059=CARTESIAN_POINT ( 'NONE',  ( -0.1623394077312214634, -0.09842519685039370636, 0.05010053824418583129 ) ) ;
#33063=ORIENTED_EDGE ( 'NONE', *, *, #16090, .F. ) ;
#33066=CARTESIAN_POINT ( 'NONE',  ( 0.07405724077823318263, -1.395669291284819868, -0.1787899950787401604 ) ) ;
#33067=CARTESIAN_POINT ( 'NONE',  ( -1.094772975963752103E-17, -1.388287401521039355, -0.1787899950787401882 ) ) ;
#33069=CARTESIAN_POINT ( 'NONE',  ( -0.07444174185955065859, -0.5841973528901317492, 0.1797182628040039087 ) ) ;
#33073=CARTESIAN_POINT ( 'NONE',  ( -9.642888182262618425E-18, -0.3129921259842520231, -0.1574803149606299191 ) ) ;
#33092=CARTESIAN_POINT ( 'NONE',  ( -0.1787899950787401604, -1.577755905458046115, -0.07405724077823318263 ) ) ;
#33093=CARTESIAN_POINT ( 'NONE',  ( 0.06523048226347956391, -1.486712598317670553, -0.1574803149606300301 ) ) ;
#33094=CARTESIAN_POINT ( 'NONE',  ( -0.1787899950787401604, -0.7509842519147402751, 0.07405724077823318263 ) ) ;
#33095=CARTESIAN_POINT ( 'NONE',  ( 0.06523048226347956391, -1.078248031496062076, 0.1574803149606297803 ) ) ;
#33104=VERTEX_POINT ( 'NONE', #16838 ) ;
#33117=FACE_OUTER_BOUND ( 'NONE', #32826, .T. ) ;
#33121=CARTESIAN_POINT ( 'NONE',  ( 0.08208618821883129080, -0.09851384146206398906, -0.1770150493296937244 ) ) ;
#33129=CARTESIAN_POINT ( 'NONE',  ( -0.07405724077823318263, -0.4311023621509605386, 0.1787899950787401604 ) ) ;
#33130=CARTESIAN_POINT ( 'NONE',  ( -1.094772975963752103E-17, -0.9158464566391496531, -0.1787899950787401882 ) ) ;
#33132=CARTESIAN_POINT ( 'NONE',  ( 3.301370929368692659E-17, -0.2667760930476126280, 0.1797182628040039365 ) ) ;
#33133=CARTESIAN_POINT ( 'NONE',  ( 0.07405724077823318263, -0.08280113358356940012, 0.1787899950787401604 ) ) ;
#33134=CARTESIAN_POINT ( 'NONE',  ( 3.284318927891251994E-17, -0.1136811023084411398, 0.1787899950787401882 ) ) ;
#33135=CARTESIAN_POINT ( 'NONE',  ( 0.2471922904502826812, -0.03219022224904102836, -0.1427165354330708902 ) ) ;
#33142=LENGTH_MEASURE_WITH_UNIT ( LENGTH_MEASURE( 0.02539999999999999897 ), #26172 ) ;
#33146=CARTESIAN_POINT ( 'NONE',  ( -0.2471922904502826812, -0.03219022224904102836, 0.1427165354330708902 ) ) ;
#33155=CARTESIAN_POINT ( 'NONE',  ( -0.1264236179284866091, -0.2465551180564728440, -0.1264236179284866091 ) ) ;
#33158=CARTESIAN_POINT ( 'NONE',  ( 0.1787899950787401604, -1.006889763725763220, 0.07405724077823318263 ) ) ;
#33176=CARTESIAN_POINT ( 'NONE',  ( 0.1264236179284866091, -0.03001968498560653523, 0.1264236179284866091 ) ) ;
#33183=CARTESIAN_POINT ( 'NONE',  ( -0.1264236179284866091, -1.359868062717427328, -0.1264236179284866091 ) ) ;
#33185=CARTESIAN_POINT ( 'NONE',  ( -0.1787899950787401604, -0.2391732282926934683, -0.07405724077823318263 ) ) ;
#33191=CYLINDRICAL_SURFACE ( 'NONE', #17209, 0.1574803149606299191 ) ;
#33196=CARTESIAN_POINT ( 'NONE',  ( 0.07405724077823318263, -1.631889763725764553, -0.1787899950787401604 ) ) ;
#33197=CARTESIAN_POINT ( 'NONE',  ( 0.1264236179284866091, -1.668799212544661348, -0.1264236179284866091 ) ) ;
#33202=CARTESIAN_POINT ( 'NONE',  ( 0.07444174185955065859, -1.366677667850763056, 0.1797182628040039087 ) ) ;
#33223=CARTESIAN_POINT ( 'NONE',  ( 0.07405724077823318263, -1.799212598371432659, 0.1787899950787401604 ) ) ;
#33229=CARTESIAN_POINT ( 'NONE',  ( -1.094772975963752103E-17, -0.2071850393163153503, -0.1787899950787401882 ) ) ;
#33232=CARTESIAN_POINT ( 'NONE',  ( -0.07968303789191254205, -0.08956740676301865045, 0.2394271090160087212 ) ) ;
#33237=CARTESIAN_POINT ( 'NONE',  ( 0.1113553986120547346, 0.1151574804224878013, 0.1113553986120547346 ) ) ;
#33244=CARTESIAN_POINT ( 'NONE',  ( 0.1264236179284866091, -0.8283719997253012890, 0.1264236179284866091 ) ) ;
#33246=CARTESIAN_POINT ( 'NONE',  ( -0.1787899950787401604, 0.1151574803687242243, -0.07405724077823318263 ) ) ;
#33255=EDGE_CURVE ( 'NONE', #30178, #30877, #13164, .T. ) ;
#33259=CARTESIAN_POINT ( 'NONE',  ( 0.07444174185955065859, -1.051717037929502885, 0.1797182628040039087 ) ) ;
#33269=CARTESIAN_POINT ( 'NONE',  ( 0.1574803149606300301, -0.7042322833570394680, -0.06523048226347956391 ) ) ;
#33272=CARTESIAN_POINT ( 'NONE',  ( 0.1264236179284866091, -0.8420275590013542866, -0.1264236179284866091 ) ) ;
#33279=CARTESIAN_POINT ( 'NONE',  ( 0.1113553986120547346, -1.705708661417322913, 0.1113553986120547346 ) ) ;
#33290=CARTESIAN_POINT ( 'NONE',  ( 0.1113553986120547346, -0.03248031485310291788, -0.1113553986120547346 ) ) ;
#33295=CARTESIAN_POINT ( 'NONE',  ( -0.1264236179284866091, -0.4445137320087661492, 0.1264236179284866091 ) ) ;
#33296=CARTESIAN_POINT ( 'NONE',  ( -0.1723610762456844747, -0.08955972947387973171, 0.1519892194067951063 ) ) ;
#33303=CARTESIAN_POINT ( 'NONE',  ( 0.07405724077823318263, -1.316929133804503937, -0.1787899950787401604 ) ) ;
#33304=CARTESIAN_POINT ( 'NONE',  ( 0.1264236179284866091, -1.550688976324188895, -0.1264236179284866091 ) ) ;
#33306=CARTESIAN_POINT ( 'NONE',  ( 2.892866454678787531E-17, 0.1102362205799679168, 0.1574803149606299191 ) ) ;
#33315=CARTESIAN_POINT ( 'NONE',  ( 2.892866454678787531E-17, -0.2539370078740157410, 0.1574803149606299191 ) ) ;
#33322=CARTESIAN_POINT ( 'NONE',  ( -0.1574803149606299191, -0.5295275589475905154, 0.000000000000000000 ) ) ;
#33326=CARTESIAN_POINT ( 'NONE',  ( -0.1677809954247694024, -0.08956119031328269031, 0.01526780091050135638 ) ) ;
#33330=CARTESIAN_POINT ( 'NONE',  ( 0.1264236179284866091, -1.560531496009228247, 0.1264236179284866091 ) ) ;
#33331=CARTESIAN_POINT ( 'NONE',  ( -0.1264236179284866091, -0.6796259841982046357, -0.1264236179284866091 ) ) ;
#33332=CARTESIAN_POINT ( 'NONE',  ( 0.06523048226347956391, -1.235728346456692384, 0.1574803149606297803 ) ) ;
#33335=EDGE_LOOP ( 'NONE', ( #27935, #13368, #44669, #34497 ) ) ;
#33357=CARTESIAN_POINT ( 'NONE',  ( 0.0003609363526977173468, -0.09851383234819251211, 0.1560916676376958856 ) ) ;
#33365=CARTESIAN_POINT ( 'NONE',  ( 0.1787899950787401882, -0.9699803149068660924, -2.189545951927503898E-17 ) ) ;
#33366=CARTESIAN_POINT ( 'NONE',  ( 0.1787899950787401604, -0.4557086613635593086, -0.07405724077823318263 ) ) ;
#33367=CARTESIAN_POINT ( 'NONE',  ( -0.1787899950787401882, -0.8666338582139527791, 0.000000000000000000 ) ) ;
#33369=CARTESIAN_POINT ( 'NONE',  ( 3.301370929368692659E-17, -0.2274060143074551343, 0.1797182628040039365 ) ) ;
#33370=CARTESIAN_POINT ( 'NONE',  ( 0.1574803149606300301, 0.1126968503937008509, -0.06523048226347956391 ) ) ;
#33372=CARTESIAN_POINT ( 'NONE',  ( 0.1787899950787401604, -0.02263779522182706935, -0.07405724077823318263 ) ) ;
#33376=FILL_AREA_STYLE_COLOUR ( '', #34636 ) ;
#33386=CARTESIAN_POINT ( 'NONE',  ( -0.1264236179284866091, -0.2071850393163153503, -0.1264236179284866091 ) ) ;
#33389=CARTESIAN_POINT ( 'NONE',  ( 0.1787899950787401604, -1.277559055064345861, -0.07405724077823318263 ) ) ;
#33418=CARTESIAN_POINT ( 'NONE',  ( -0.07405724077823318263, -1.386934991851286769, 0.1787899950787401604 ) ) ;
#33420=CARTESIAN_POINT ( 'NONE',  ( -1.094772975963752103E-17, -0.4040354330171023745, -0.1787899950787401882 ) ) ;
#33429=CARTESIAN_POINT ( 'NONE',  ( -0.1787899950787401882, -1.698326771599779628, 0.000000000000000000 ) ) ;
#33430=CARTESIAN_POINT ( 'NONE',  ( 0.07405724077823318263, -1.666338582623402953, -0.1787899950787401604 ) ) ;
#33433=CARTESIAN_POINT ( 'NONE',  ( -0.1797182628040039087, -1.381441447378320531, -0.07444174185955065859 ) ) ;
#33440=CARTESIAN_POINT ( 'NONE',  ( -0.07405724077823318263, 0.1446850394238423654, -0.1787899950787401604 ) ) ;
#33454=CARTESIAN_POINT ( 'NONE',  ( -0.1797182628040039087, -0.003488691472809330677, -0.07444174185955065859 ) ) ;
#33459=CARTESIAN_POINT ( 'NONE',  ( -0.06523048226347956391, 0.05856299212598428672, 0.1574803149606297803 ) ) ;
#33462=CARTESIAN_POINT ( 'NONE',  ( 0.1264236179284866091, -0.1825787401037169411, 0.1264236179284866091 ) ) ;
#33465=CARTESIAN_POINT ( 'NONE',  ( -0.08640460078248797526, -0.09201407021823122812, 0.2355472506763592044 ) ) ;
#33468=CARTESIAN_POINT ( 'NONE',  ( -0.1574803149606300301, 0.1373031497138262058, -0.06523048226347956391 ) ) ;
#33474=FACE_OUTER_BOUND ( 'NONE', #33335, .T. ) ;
#33476=CARTESIAN_POINT ( 'NONE',  ( 0.1264236179284866091, -0.9858523146859311526, 0.1264236179284866091 ) ) ;
#33485=CARTESIAN_POINT ( 'NONE',  ( 0.1264236179284866091, -0.5319881889226142357, -0.1264236179284866091 ) ) ;
#33489=CARTESIAN_POINT ( 'NONE',  ( -0.1797182628040039087, -1.061559557614541349, 0.07444174185955065859 ) ) ;
#33499=CARTESIAN_POINT ( 'NONE',  ( -0.06523048226347956391, -0.6796259841444414196, 0.1574803149606297803 ) ) ;
#33502=CARTESIAN_POINT ( 'NONE',  ( -0.1787899950787401604, -0.7066929133320629663, 0.07405724077823318263 ) ) ;
#33509=CARTESIAN_POINT ( 'NONE',  ( 0.06523048226347956391, -1.614665354330708347, -0.1574803149606300301 ) ) ;
#33515=CARTESIAN_POINT ( 'NONE',  ( 0.1574803149606299191, -0.3129921258767248138, -1.928577636452523993E-17 ) ) ;
#33526=CARTESIAN_POINT ( 'NONE',  ( -0.07405724077823318263, -0.4420531020875061445, 0.1787899950787401604 ) ) ;
#33527=CARTESIAN_POINT ( 'NONE',  ( -0.1377300245925881794, -0.08955984809379961831, 0.1824063869217125988 ) ) ;
#33528=DIRECTION ( 'NONE',  ( 0.000000000000000000, 0.000000000000000000, 1.000000000000000000 ) ) ;
#33533=CARTESIAN_POINT ( 'NONE',  ( -0.07405724077823318263, -1.741265700512703019, 0.1787899950787401604 ) ) ;
#33539=CARTESIAN_POINT ( 'NONE',  ( -1.094772975963752103E-17, -1.275098425143086578, -0.1787899950787401882 ) ) ;
#33540=CARTESIAN_POINT ( 'NONE',  ( -0.1787899950787401604, -1.533464566875370805, 0.07405724077823318263 ) ) ;
#33547=CARTESIAN_POINT ( 'NONE',  ( -0.1574803149606297803, -0.2613188976377954220, 0.06523048226347956391 ) ) ;
#33554=CARTESIAN_POINT ( 'NONE',  ( -0.1691510595345104007, -0.08955828895034714798, -0.02489612667484852188 ) ) ;
#33563=CARTESIAN_POINT ( 'NONE',  ( -0.07405724077823318263, -1.582677165300567346, -0.1787899950787401604 ) ) ;
#33564=CARTESIAN_POINT ( 'NONE',  ( -0.1787899950787401882, -0.7928149605761574126, 0.000000000000000000 ) ) ;
#33565=CARTESIAN_POINT ( 'NONE',  ( 0.1113553986120547346, -1.262795275590551158, -0.1113553986120547346 ) ) ;
#33575=CARTESIAN_POINT ( 'NONE',  ( 0.06523048226347956391, -1.329232283357040467, -0.1574803149606300301 ) ) ;
#33584=CARTESIAN_POINT ( 'NONE',  ( 0.05940473271390560306, 0.07959431159476453022, 0.2511357324426306548 ) ) ;
#33591=CARTESIAN_POINT ( 'NONE',  ( -0.1854798818493685053, -0.09842519685039370636, 0.1431202509172336546 ) ) ;
#33600=CARTESIAN_POINT ( 'NONE',  ( 0.07405724077823318263, -0.9232283464029299447, -0.1787899950787401604 ) ) ;
#33602=CARTESIAN_POINT ( 'NONE',  ( -1.094772975963752103E-17, -1.033956692859621995, -0.1787899950787401882 ) ) ;
#33605=CARTESIAN_POINT ( 'NONE',  ( 0.1270800023317771588, -0.3799650694255653494, 0.1270800023317771588 ) ) ;
#33606=CARTESIAN_POINT ( 'NONE',  ( -0.1113553986120547346, 0.09547244094488190058, 0.1113553986120547346 ) ) ;
#33607=CARTESIAN_POINT ( 'NONE',  ( -0.1787899950787401604, -0.04232283459190575720, 0.07405724077823318263 ) ) ;
#33609=( NAMED_UNIT ( * ) SI_UNIT ( $, .STERADIAN. ) SOLID_ANGLE_UNIT ( ) ) ;
#33618=CARTESIAN_POINT ( 'NONE',  ( 0.1787899950787401882, -0.2613188975840319284, -2.189545951927503898E-17 ) ) ;
#33620=CARTESIAN_POINT ( 'NONE',  ( -0.1787899950787401882, -1.260334645615527549, 0.000000000000000000 ) ) ;
#33632=CARTESIAN_POINT ( 'NONE',  ( 0.001029233576901327765, -0.09840078316628074473, -0.1790406922995744221 ) ) ;
#33649=CARTESIAN_POINT ( 'NONE',  ( 0.07405724077823318263, -1.445990109961521553, -0.1787899950787401604 ) ) ;
#33651=CARTESIAN_POINT ( 'NONE',  ( 0.1787899950787401882, -0.4532480314422991929, -2.189545951927503898E-17 ) ) ;
#33652=VERTEX_POINT ( 'NONE', #19858 ) ;
#33654=DIRECTION ( 'NONE',  ( 0.000000000000000000, 1.000000000000000000, 0.000000000000000000 ) ) ;
#33660=CARTESIAN_POINT ( 'NONE',  ( 0.1787899950787401604, -1.754921259788755128, -0.07405724077823318263 ) ) ;
#33661=CARTESIAN_POINT ( 'NONE',  ( 0.07405724077823318263, -1.705708661363559253, -0.1787899950787401604 ) ) ;
#33666=CARTESIAN_POINT ( 'NONE',  ( -0.1113553986120547346, -0.8100393700787401619, 0.1113553986120547346 ) ) ;
#33668=CARTESIAN_POINT ( 'NONE',  ( 0.1270800023317771588, -1.364217037929501997, 0.1270800023317771588 ) ) ;
#33678=CARTESIAN_POINT ( 'NONE',  ( 0.06523048226347956391, -0.8321850392625521620, 0.1574803149606297803 ) ) ;
#33679=CARTESIAN_POINT ( 'NONE',  ( -0.1787899950787401882, 0.1520669291876218521, 0.000000000000000000 ) ) ;
#33693=CARTESIAN_POINT ( 'NONE',  ( 0.07444174185955065859, -0.06746506942556518283, 0.1797182628040039087 ) ) ;
#33695=CARTESIAN_POINT ( 'NONE',  ( 0.06523048226347956391, -1.053641732175938595, -0.1574803149606300301 ) ) ;
#33696=CARTESIAN_POINT ( 'NONE',  ( 0.1787899950787401604, -1.282480314906867314, -0.07405724077823318263 ) ) ;
#33704=CARTESIAN_POINT ( 'NONE',  ( -0.1264236179284866091, -0.1628937007336379861, -0.1264236179284866091 ) ) ;
#33711=CARTESIAN_POINT ( 'NONE',  ( -0.1113553986120547346, -0.01279527548302413463, 0.1113553986120547346 ) ) ;
#33719=CARTESIAN_POINT ( 'NONE',  ( -0.07405724077823318263, -0.9932342044497125544, 0.1787899950787401604 ) ) ;
#33721=CARTESIAN_POINT ( 'NONE',  ( -0.1787899950787401604, 0.08070866147108628208, 0.07405724077823318263 ) ) ;
#33725=DIRECTION ( 'NONE',  ( 0.000000000000000000, 0.000000000000000000, 1.000000000000000000 ) ) ;
#33727=CARTESIAN_POINT ( 'NONE',  ( 0.1787899950787401604, -0.5393700786863945273, 0.07405724077823318263 ) ) ;
#33733=CARTESIAN_POINT ( 'NONE',  ( -0.07444174185955065859, -1.032031998559423736, -0.1797182628040039087 ) ) ;
#33738=DIRECTION ( 'NONE',  ( 0.000000000000000000, 1.000000000000000000, 0.000000000000000000 ) ) ;
#33744=CARTESIAN_POINT ( 'NONE',  ( -9.642888182262618425E-18, -0.6968503935932598425, -0.1574803149606299191 ) ) ;
#33749=CARTESIAN_POINT ( 'NONE',  ( 3.284318927891251994E-17, -0.6993110235682834519, 0.1787899950787401882 ) ) ;
#33756=CARTESIAN_POINT ( 'NONE',  ( 0.1574803149606300301, -1.663877952755905332, 0.06523048226347956391 ) ) ;
#33764=CARTESIAN_POINT ( 'NONE',  ( 0.1264236179284866091, -1.594980314906866203, -0.1264236179284866091 ) ) ;
#33770=CARTESIAN_POINT ( 'NONE',  ( 0.05635946233522097504, 0.07780450164205243713, -0.2528939201155193106 ) ) ;
#33772=CARTESIAN_POINT ( 'NONE',  ( -0.1787899950787401604, -0.5700058579930178393, -0.07405724077823318263 ) ) ;
#33773=CARTESIAN_POINT ( 'NONE',  ( 0.007747115091317480218, -0.08955984173353109812, 0.2203066983908811283 ) ) ;
#33780=CARTESIAN_POINT ( 'NONE',  ( 3.624546087963248077E-17, -0.09842519685039370636, 0.2854330708661417804 ) ) ;
#33790=CARTESIAN_POINT ( 'NONE',  ( 0.06523048226347956391, -0.2514763779527561249, 0.1574803149606297803 ) ) ;
#33793=ORIENTED_EDGE ( 'NONE', *, *, #1789, .T. ) ;
#33794=CARTESIAN_POINT ( 'NONE',  ( -0.1305514342443539477, -0.09246813122503681759, -0.1221825334204538205 ) ) ;
#33800=CARTESIAN_POINT ( 'NONE',  ( -0.1539388023598581845, -0.08956124721700792213, 0.06042638813536082426 ) ) ;
#33806=ADVANCED_FACE ( 'NONE', ( #25105 ), #10754, .T. ) ;
#33809=CARTESIAN_POINT ( 'NONE',  ( 0.1264236179284866091, -1.590059055064346305, -0.1264236179284866091 ) ) ;
#33810=CARTESIAN_POINT ( 'NONE',  ( -0.07405724077823318263, -0.8248031495525351975, 0.1787899950787401604 ) ) ;
#33812=CARTESIAN_POINT ( 'NONE',  ( 0.1574803149606300301, -1.230807086614172929, 0.06523048226347956391 ) ) ;
#33829=CARTESIAN_POINT ( 'NONE',  ( -0.1713132547969852260, -0.09842519685039370636, 0.1581802318308832833 ) ) ;
#33840=CARTESIAN_POINT ( 'NONE',  ( 0.1787899950787401882, -0.9306102361667086820, -2.189545951927503898E-17 ) ) ;
#33841=CARTESIAN_POINT ( 'NONE',  ( 3.284318927891251994E-17, -1.014271653489543290, 0.1787899950787401882 ) ) ;
#33842=CARTESIAN_POINT ( 'NONE',  ( 0.1797182628040039087, -0.3775044395043055112, 0.07444174185955046430 ) ) ;
#33843=CARTESIAN_POINT ( 'NONE',  ( -0.1113553986120547346, 0.08562992125984252023, -0.1113553986120547346 ) ) ;
#33850=( NAMED_UNIT ( * ) PLANE_ANGLE_UNIT ( ) SI_UNIT ( $, .RADIAN. ) ) ;
#33854=( GEOMETRIC_REPRESENTATION_CONTEXT ( 3 ) GLOBAL_UNCERTAINTY_ASSIGNED_CONTEXT ( ( #26848 ) ) GLOBAL_UNIT_ASSIGNED_CONTEXT ( ( #44575, #33850, #33609 ) ) REPRESENTATION_CONTEXT ( 'NONE', 'WORKASPACE' ) ) ;
#33858=CARTESIAN_POINT ( 'NONE',  ( -0.1787899950787401604, -0.4409448818359998357, -0.07405724077823318263 ) ) ;
#33860=CARTESIAN_POINT ( 'NONE',  ( -0.1787899950787401604, -1.297244094434425010, 0.07405724077823318263 ) ) ;
#33888=CARTESIAN_POINT ( 'NONE',  ( 3.284318927891251994E-17, -1.502584598150498163, 0.1787899950787401882 ) ) ;
#33890=CARTESIAN_POINT ( 'NONE',  ( -1.094772975963752103E-17, -0.3646653542769452971, -0.1787899950787401882 ) ) ;
#33896=CARTESIAN_POINT ( 'NONE',  ( 0.2471922904502826812, 0.03219022224904106305, 0.1427165354330708902 ) ) ;
#33902=CARTESIAN_POINT ( 'NONE',  ( 3.284318927891251994E-17, -1.806594488135212728, 0.1787899950787401882 ) ) ;
#33903=PRODUCT_CONTEXT ( 'NONE', #320, 'mechanical' ) ;
#33907=CARTESIAN_POINT ( 'NONE',  ( -9.642888182262618425E-18, -0.6673228346456693272, -0.1574803149606299191 ) ) ;
#33909=CARTESIAN_POINT ( 'NONE',  ( 0.1797182628040039087, -1.474945384386196379, -0.07444174185955065859 ) ) ;
#33915=CARTESIAN_POINT ( 'NONE',  ( -0.1574803149606300301, -0.8075787400499540025, -0.06523048226347956391 ) ) ;
#33926=CARTESIAN_POINT ( 'NONE',  ( 0.1574803149606300301, -0.04970472440944883469, 0.06523048226347956391 ) ) ;
#33928=CARTESIAN_POINT ( 'NONE',  ( 0.1270800023317771588, -0.09453199855942362451, -0.1270800023317771588 ) ) ;
#33929=CARTESIAN_POINT ( 'NONE',  ( 0.1787899950787401604, -1.248031496009228913, 0.07405724077823318263 ) ) ;
#33939=CARTESIAN_POINT ( 'NONE',  ( -7.939671275311751530E-17, -0.03219022224904082713, -0.2854330708661417804 ) ) ;
#33942=CARTESIAN_POINT ( 'NONE',  ( 2.892866454678787531E-17, -0.1259842518609769757, 0.1574803149606299191 ) ) ;
#33952=CARTESIAN_POINT ( 'NONE',  ( -0.1787899950787401604, 0.04133858273092887170, 0.07405724077823318263 ) ) ;
#33959=CARTESIAN_POINT ( 'NONE',  ( 0.1264236179284866091, -0.5418307086076535883, 0.1264236179284866091 ) ) ;
#33963=CARTESIAN_POINT ( 'NONE',  ( 3.301370929368692659E-17, -1.014807589110604313, 0.1797182628040039365 ) ) ;
#33969=CARTESIAN_POINT ( 'NONE',  ( -0.02739131347899105909, -0.09752745740044843625, 0.1550798682808147422 ) ) ;
#33970=CARTESIAN_POINT ( 'NONE',  ( -0.1113553986120547346, -0.6919291337507401662, -0.1113553986120547346 ) ) ;
#33971=CARTESIAN_POINT ( 'NONE',  ( -0.07405724077823318263, 0.08562992131360593062, 0.1787899950787401604 ) ) ;
#33976=CARTESIAN_POINT ( 'NONE',  ( 0.1787899950787401882, -0.7682086613635590311, -2.189545951927503898E-17 ) ) ;
#33979=CARTESIAN_POINT ( 'NONE',  ( -0.06523048226347956391, -1.467027558947591848, 0.1574803149606297803 ) ) ;
#33983=CARTESIAN_POINT ( 'NONE',  ( -0.06523048226347956391, -1.673720472440946017, 0.1574803149606297803 ) ) ;
#33989=CARTESIAN_POINT ( 'NONE',  ( 0.1264236179284866091, 0.09793307091990532953, -0.1264236179284866091 ) ) ;
#33990=CARTESIAN_POINT ( 'NONE',  ( 0.1574803149606300301, -0.3548228345381419513, 0.06523048226347956391 ) ) ;
#33991=CARTESIAN_POINT ( 'NONE',  ( 0.1264236179284866091, -1.476870078686393750, -0.1264236179284866091 ) ) ;
#34000=CARTESIAN_POINT ( 'NONE',  ( 0.1264236179284866091, -0.5134113698040417839, 0.1264236179284866091 ) ) ;
#34004=( BOUNDED_CURVE ( )  B_SPLINE_CURVE ( 2, ( #8913, #31446, #13239, #6243, #31213, #45789, #27867, #23543, #24013 ),
 .UNSPECIFIED., .F., .T. ) 
 B_SPLINE_CURVE_WITH_KNOTS ( ( 3, 2, 2, 2, 3 ),
 ( 0.1250000000000000000, 0.1275000000000000022, 0.1300000000000000044, 0.1325000000000000067, 0.1350000000000000089 ),
 .UNSPECIFIED. ) 
 CURVE ( )  GEOMETRIC_REPRESENTATION_ITEM ( )  RATIONAL_B_SPLINE_CURVE ( ( 1.000000000000000000, 0.9238795325112869605, 1.000000000000000000, 0.9238795325112869605, 1.000000000000000000, 0.9238795325112869605, 1.000000000000000000, 0.9238795325112869605, 1.000000000000000000 ) ) 
 REPRESENTATION_ITEM ( '' )  ) ;
#34009=CARTESIAN_POINT ( 'NONE',  ( 0.2471921300642929697, -0.09379707428445169248, 0.03645430680490753528 ) ) ;
#34013=CARTESIAN_POINT ( 'NONE',  ( 0.1787899950787401604, -1.326771653489542402, 0.07405724077823318263 ) ) ;
#34014=CARTESIAN_POINT ( 'NONE',  ( 0.1787899950787401882, -1.476870078686393750, -2.189545951927503898E-17 ) ) ;
#34022=CARTESIAN_POINT ( 'NONE',  ( -0.06523048226347956391, -0.2170275590551181411, 0.1574803149606297803 ) ) ;
#34040=CARTESIAN_POINT ( 'NONE',  ( 0.1264236179284866091, -1.708169291284818980, -0.1264236179284866091 ) ) ;
#34041=CARTESIAN_POINT ( 'NONE',  ( 0.07405724077823318263, -0.9232283464029299447, -0.1787899950787401604 ) ) ;
#34042=CARTESIAN_POINT ( 'NONE',  ( 0.1574803149606299191, -1.149606299212598381, -1.928577636452523993E-17 ) ) ;
#34050=EDGE_LOOP ( 'NONE', ( #12343, #10033, #15136, #9902, #26683 ) ) ;
#34062=CARTESIAN_POINT ( 'NONE',  ( -0.1749890002391197019, -0.09842519685039370636, -0.1786399317641141626 ) ) ;
#34074=CARTESIAN_POINT ( 'NONE',  ( -1.094772975963752103E-17, -0.9207677164816693294, -0.1787899950787401882 ) ) ;
#34075=CARTESIAN_POINT ( 'NONE',  ( -0.07405724077823318263, -1.070866141678519456, -0.1787899950787401604 ) ) ;
#34077=CARTESIAN_POINT ( 'NONE',  ( -0.1270800023317771588, -0.3996501087956441101, -0.1270800023317771588 ) ) ;
#34078=CARTESIAN_POINT ( 'NONE',  ( 0.1113553986120547346, -1.813976377845228249, 0.1113553986120547346 ) ) ;
#34087=CARTESIAN_POINT ( 'NONE',  ( 0.1787899950787401882, -0.3794291338045042705, -2.189545951927503898E-17 ) ) ;
#34089=CARTESIAN_POINT ( 'NONE',  ( -0.07405724077823318263, -1.307086614119465695, -0.1787899950787401604 ) ) ;
#34103=CARTESIAN_POINT ( 'NONE',  ( 0.04296924029584964916, -0.09842683234878628340, -0.1736138147098973683 ) ) ;
#34119=CARTESIAN_POINT ( 'NONE',  ( 0.1787899950787401604, -1.490281448544198639, -0.07405724077823318263 ) ) ;
#34122=CARTESIAN_POINT ( 'NONE',  ( 0.1787899950787401604, -0.4901574802611972093, -0.07405724077823318263 ) ) ;
#34130=CARTESIAN_POINT ( 'NONE',  ( 0.07405724077823318263, -1.749999999946236340, -0.1787899950787401604 ) ) ;
#34132=CARTESIAN_POINT ( 'NONE',  ( 0.1678155187887284683, -0.09842519685039373412, 0.05062837720671468922 ) ) ;
#34134=CARTESIAN_POINT ( 'NONE',  ( 0.1574803149606299191, -0.7559055118110236116, -1.928577636452523993E-17 ) ) ;
#34136=CARTESIAN_POINT ( 'NONE',  ( 0.1797182628040039087, -1.558606801709029543, 0.07444174185955046430 ) ) ;
#34145=CARTESIAN_POINT ( 'NONE',  ( -0.1264236179284866091, -0.03986220467064590517, 0.1264236179284866091 ) ) ;
#34159=CARTESIAN_POINT ( 'NONE',  ( -0.07444174185955065859, -0.07238632926808483137, 0.1797182628040039087 ) ) ;
#34160=CARTESIAN_POINT ( 'NONE',  ( -0.1264236179284866091, -1.309547244040724312, -0.1264236179284866091 ) ) ;
#34171=CARTESIAN_POINT ( 'NONE',  ( -0.05769093565148274150, -0.07859528327913033185, -0.2521251929553486315 ) ) ;
#34173=CARTESIAN_POINT ( 'NONE',  ( -0.1574803149606297803, -0.01525590540428398145, 0.06523048226347956391 ) ) ;
#34182=CARTESIAN_POINT ( 'NONE',  ( -0.1264236179284866091, -0.9563247556308129838, 0.1264236179284866091 ) ) ;
#34184=CARTESIAN_POINT ( 'NONE',  ( 0.07405724077823318263, -0.01279527553678768380, -0.1787899950787401604 ) ) ;
#34191=CARTESIAN_POINT ( 'NONE',  ( -0.07405724077823318263, -0.5885826771115909573, 0.1787899950787401604 ) ) ;
#34195=CARTESIAN_POINT ( 'NONE',  ( 0.07444174185955046430, -1.036953258401943412, -0.1797182628040039087 ) ) ;
#34204=CARTESIAN_POINT ( 'NONE',  ( 0.1113553986120547346, -0.6624015746956219974, -0.1113553986120547346 ) ) ;
#34209=CARTESIAN_POINT ( 'NONE',  ( 0.1787899950787401604, -0.8494094487651332459, 0.07405724077823318263 ) ) ;
#34213=CARTESIAN_POINT ( 'NONE',  ( -9.642888182262618425E-18, -1.641732283357039357, -0.1574803149606299191 ) ) ;
#34220=CARTESIAN_POINT ( 'NONE',  ( 0.1574803149606300301, -1.781988188976379117, 0.06523048226347956391 ) ) ;
#34225=CARTESIAN_POINT ( 'NONE',  ( -1.094772975963752103E-17, -1.590059055064346305, -0.1787899950787401882 ) ) ;
#34233=CARTESIAN_POINT ( 'NONE',  ( 0.1787899950787401604, -0.5109507398827820568, 0.07405724077823318263 ) ) ;
#34234=CARTESIAN_POINT ( 'NONE',  ( -0.08566400215306142762, -0.08956101637306594643, -0.1598881813297279575 ) ) ;
#34242=CARTESIAN_POINT ( 'NONE',  ( -0.07405724077823318263, -1.469488188922614791, -0.1787899950787401604 ) ) ;
#34243=CARTESIAN_POINT ( 'NONE',  ( -1.094772975963752103E-17, -1.506397637741511586, -0.1787899950787401882 ) ) ;
#34248=CARTESIAN_POINT ( 'NONE',  ( -0.1574803149606299191, -0.4212598425196850127, 0.000000000000000000 ) ) ;
#34254=( BOUNDED_SURFACE ( )  B_SPLINE_SURFACE ( 1, 2, ( 
 ( #33679, #18787, #3704, #33440, #557, #40805, #15213, #44406, #30105, #11622, #791, #32965, #89, #1039, #15697, #30558, #5345, #31025, #1998, #16847, #30797, #16625, #26956, #41508, #41987, #8714, #12337, #8957, #45120, #31488, #12094, #31255, #45362, #9444, #45832, #23349, #26717, #16400, #37961, #34369, #5111, #23577, #5835, #41272, #19734, #4873, #12813, #9191, #2228, #12575, #27203, #23809, #19501, #19968, #1509, #38428, #13041, #27678, #20201, #5594, #34608, #34854, #41753, #45591, #16163, #1275, #38185, #15929, #42240, #24060, #1758, #8472, #38665, #27443, #20444, #35080, #23106, #37722, #34145, #28364, #2695, #6291, #36264, #18031, #46075, #17322, #13725, #10143, #42472, #3166, #27909, #17795, #46780, #3415, #39115, #36009, #24752, #14216, #39586, #42933, #2920, #28855, #13275, #38890, #31959, #9676, #24292, #20911, #32442, #46543, #6052, #31724, #39347, #20679, #21383, #6767, #13501, #47020, #6529, #10624, #28133, #21142, #35319, #25226, #35778, #39814, #2459, #17555, #42690, #28617, #17086, #7003, #32193, #21630, #46317, #9907, #24517, #13967, #35551, #43177, #10385, #24991, #26420, #14445, #3648, #25484, #33386, #29804, #22799, #18498, #276, #44351, #40050, #40518, #29354, #11558, #4325, #733, #40750, #26183, #7707, #7947, #33155, #18727, #11094, #21872, #14921, #36493, #33618, #22565, #44127, #47264, #44582, #18268, #4108, #30039, #11801, #22323, #18958, #29586, #36716, #40286, #37407, #4564, #32677, #3879, #11326, #25938, #29099, #37181, #43657, #15395, #501, #10864, #25717, #40988, #36951, #8173, #7250, #15160, #32911, #31, #14680, #43896, #7471, #22091, #23999, #12268, #23749, #37899, #26659, #4814, #45300, #15634, #41925, #12753, #34087, #38360, #1448, #34791, #1217, #5057, #8412, #45768, #16106, #1931, #12036, #30731, #15868, #1692, #38598, #30496, #45056, #19910, #19437, #26891, #5531, #34316, #23040, #30272, #19199, #33858, #16565, #37658, #12518, #38130, #9132, #977, #19674, #20146, #41448, #8649, #16341, #23286, #27141, #41693, #8895, #44824, #23526, #41206, #5290, #34540, #30962, #45529, #27382, #12978, #31195, #27616, #42170, #9378, #2859, #43361, #39058, #20851, #17496, #46013, #13665, #2399, #32127, #24936, #21321, #13905, #46718, #28301, #28552, #6227, #39293, #31669, #42412, #35493, #9616, #6708, #43120, #17267, #20379, #17733, #24235, #24692, #3109, #32383, #42866, #39529, #2633, #9847, #13446, #10568, #25170, #5773, #24457, #31903, #46484, #2168, #10324, #35017, #35952, #6466, #16791, #46247, #46964, #10081, #14153, #28797, #21084, #35724, #31431, #13218, #27853, #38832, #5995, #20616, #28075, #35264, #17032, #42636, #25422, #18443, #36204, #15107, #33331, #7189, #11503, #22039, #7891, #21814, #25657, #29039, #18908, #36665, #22509, #32622, #3823, #36442, #22265, #11750, #3594, #18214, #40466, #39996, #32856, #44300, #7421, #43598, #3356, #44534, #39754, #4274, #10809, #33094, #25884, #29752, #6944, #11041, #26124, #47450, #14622, #36902, #29292, #43840, #215, #40232, #21566, #17968, #40695, #14865, #33564, #682, #29524, #44075, #15337, #29989, #47209, #7649, #14389, #4056, #18671, #454, #45006, #33810, #11986, #5008, #22749, #1646, #19867, #41161, #45482, #8600, #41880, #8365, #12219, #15585, #5486, #23240, #9086, #19144, #37853, #22991, #8845, #45721, #37602, #4763, #27090, #26609, #19390, #30921, #41402, #30223, #37355, #31152, #26371, #23706, #44770, #19627, #45248, #16291, #40930, #26842, #12710, #34041, #1166, #23482, #15825, #30450, #34268, #1398, #8126, #4509, #27335, #16058, #38313, #20101, #30685, #927, #12469, #41641, #38083, #5240, #34492, #34747, #1888, #16523, #5723, #13613, #10028, #3051, #46202, #28031, #24648, #20339, #20803, #9570, #39242, #32080, #28502, #21033, #6416, #35444, #35678, #13401, #46433, #38791, #2122, #42590, #16751, #13855, #2815, #24411, #27570, #24882, #31392, #31855, #10272, #39479, #2582, #46669, #9802, #16983, #20571, #17680, #32331, #12937, #31622, #39015, #6179, #9332, #17446, #42118, #43068, #28253, #23952, #5948, #6656, #17220, #21273, #35898, #38558, #34977, #42816, #45961, #13175, #27812, #42372, #24189, #35212, #2350, #30346, #44894, #39948, #18161, #44650, #28747, #15229, #37490, #19511, #15711, #36146, #43545, #43311, #3549, #32801, #10515, #10759, #39702, #22878, #25366, #25113, #572, #26732, #14101, #21508, #21759, #22644, #23120, #29876, #11867, #3300, #30117, #26492, #7138, #41054, #37249, #8252, #12107, #44418, #8013, #32572, #4646, #4401, #19273, #41285, #33929, #37733, #11635, #36395, #26255, #4889, #17919, #40818, #1052, #8485, #47157, #46911, #19028, #6890, #33696, #14341, #28987, #804, #15469, #13053, #41764, #31267, #38679, #41521, #38198, #34160, #23821, #34619, #16636, #24071, #5359, #5122, #1769, #19979, #34382, #31036, #16858, #9686, #1521, #45603, #2239, #46083, #45846, #5847, #38901, #6062, #2010, #27214, #1289, #15944, #8967, #30569, #12822, #5607, #38439, #16174, #45375, #12591, #27455, #27690, #41998, #9203, #20215, #42253, #43554, #47164, #21767, #21516, #3555, #3309, #40187, #21996, #3780, #18169, #32808, #33045, #171, #44024, #15061, #11228, #25839, #40420, #7604, #36850, #4004, #4712, #37307, #12168, #41349, #19096, #19340, #874, #30875, #33991, #4456, #26792, #34690, #22701, #30179, #30407, #30635, #31104, #8551, #5190, #11939, #38031, #19814, #1116, #34442, #45197, #1590, #5430, #23187, #16010, #41119, #16243, #12419, #45436, #20048, #12655, #45667, #37800, #15777, #4951, #12885, #26560, #44956, #27282, #41830, #8313, #9033, #19580, #27518, #41589, #23655, #22943, #38265, #1833, #16472, #34225, #8079, #33764, #15536, #1353, #44720, #27040, #8793, #37551, #23427, #13350, #34927, #9750, #27978, #45912, #42547, #24829, #21224, #13128, #24364, #28449, #6610, #24593, #17394, #43016, #35850, #9984, #35159, #3002, #46860, #2303, #39431, #6127, #13568, #31806, #46623, #5674, #42323, #32033, #39191, #20281, #42072, #16931, #24141, #16702, #38503, #2075, #2770, #31331, #10223, #46155, #31573, #20524, #14047, #27762, #38962, #9275, #35394, #9517, #17636, #35628, #23895, #6366, #38745, #20751, #13807, #5909, #32282, #2539, #17167, #46391, #28204, #42767, #20982, #25314, #21460, #3957, #7089, #10467, #47354, #7792, #43263, #3248, #3500, #3730, #4184, #14527, #25794, #32518, #11181, #40366, #39901, #7555 ),
 ( #39656, #33468, #588, #44206, #47104, #21949, #117, #18579, #28695, #29193, #33237, #43499, #10709, #22165, #21714, #28938, #25564, #14294, #25064, #6839, #364, #43740, #26023, #15014, #36346, #36091, #32994, #18114, #32757, #10945, #40136, #22409, #17874, #7333, #36571, #29434, #36804, #18811, #18350, #14764, #29667, #43977, #11405, #40598, #37035, #34397, #30821, #23377, #41534, #23131, #37984, #1065, #1306, #41067, #4414, #44907, #19044, #16190, #5138, #26741, #29889, #27227, #33711, #34173, #12606, #41780, #4903, #1537, #12120, #19288, #22890, #5374, #34634, #15244, #15961, #12365, #19995, #15723, #30359, #26983, #8027, #37745, #11882, #8741, #45391, #8981, #19764, #23602, #19524, #38214, #41300, #30581, #8265, #820, #8501, #15482, #44434, #11649, #45145, #26272, #40835, #30126, #22656, #37261, #44666, #26507, #37503, #4661, #33942, #10098, #40014, #21832, #1784, #21103, #17513, #13926, #45618, #6965, #31053, #21587, #3126, #7210, #42887, #39774, #28570, #17987, #43380, #32148, #6723, #32641, #16425, #42016, #35741, #12836, #27468, #24708, #36227, #2877, #9222, #34880, #43137, #23840, #25187, #10590, #16655, #3379, #46739, #47227, #31282, #10343, #38452, #29061, #24952, #14411, #5623, #39550, #45859, #32403, #20231, #13072, #28320, #17757, #2025, #39309, #43617, #21339, #6483, #35970, #46979, #14172, #10825, #28817, #25441, #26072, #29938, #44719, #11227, #44481, #7387, #33044, #22457, #40643, #37078, #4229, #33515, #25374, #39953, #26326, #19095, #21766, #18168, #32807, #47404, #14576, #37799, #1352, #12167, #8792, #8312, #22942, #45196, #33990, #38502, #27281, #12418, #37550, #27039, #1589, #30874, #41829, #9032, #5429, #45666, #34689, #42071, #43015, #32032, #38744, #13127, #6126, #42546, #2302, #16930, #46390, #24828, #42766, #6609, #9983, #20981, #35627, #27761, #32281, #21223, #8463, #34597, #30548, #24051, #31246, #23092, #20435, #46063, #41263, #30786, #38173, #37710, #19490, #19957, #12328, #41498, #23340, #1747, #16391, #31011, #23799, #28353, #20666, #6278, #46302, #206, #35542, #2682, #24742, #7642, #31950, #6517, #32184, #22029, #4045, #25873, #40458, #36891, #18662, #33322, #27899, #12206, #1156, #26831, #23467, #917, #22979, #15577, #41387, #15811, #23226, #38069, #19615, #44288, #8354, #11492, #4266, #9073, #31140, #27557, #13387, #42579, #45708, #31840, #34964, #9315, #16969, #6169, #31377, #9788, #46424, #42360, #25101, #14560, #18384, #24866, #39691, #2801, #25357, #3287, #18149, #149, #47147, #28484, #28976, #21750, #32318, #3538, #29463, #11211, #7588, #17433, #13841, #34204, #19321, #23161, #37779, #4933, #41564, #37287, #33499, #19072, #22203, #11681, #26306, #33970, #15754, #33744, #1331, #854, #33269, #30610, #11915, #9009, #20500, #20729, #31550, #45647, #46128, #17138, #30852, #27498, #5170, #9495, #9251, #19789, #27258, #42048, #23869, #34909, #31312, #46597, #14021, #32964, #88, #28421, #10438, #29157, #14735, #7060, #18084, #10918, #42742, #10677, #17608, #32004, #39400, #21687, #3472, #47323, #790, #19013, #33915, #7527, #25992, #44880, #26478, #335, #14982, #11621, #37004, #4383, #33678, #44638, #23105, #11854, #46074, #12812, #41986, #34853, #15928, #5110, #31254, #26955, #27677, #34368, #2227, #9443, #45361, #35079, #38889, #6051, #38664, #20443, #27202, #46316, #46779, #7002, #17085, #32676, #28363, #6528, #28132, #2919, #24990, #42689, #6766, #36008, #21629, #28854, #43415, #36263, #30, #11093, #3878, #22322, #26182, #275, #36950, #26419, #14920, #18957, #8172, #29585, #37406, #22564, #4107, #18726, #41692, #45767, #5056, #38597, #20378, #13217, #45055, #12267, #26890, #41447, #1447, #2398, #3108, #9615, #13445, #4508, #25656, #46140, #19389, #35380, #28192, #2755, #28680, #3229, #36556, #17861, #28434, #29173, #43725, #18568, #7778, #37248, #4645, #41520, #33695, #15710, #29875, #23360, #350, #44192, #20456, #42252, #16857, #17096, #9202, #24070, #5358, #27919, #35091, #31736, #5121, #19746, #12590, #38438, #1768, #23820, #12821, #5606, #20214, #21641, #7015, #28377, #40063, #25000, #14691, #18042, #32924, #24762, #47277, #43, #29365, #21393, #43905, #17332, #13736, #3177, #6540, #14224, #47034, #2928, #987, #29816, #18510, #40761, #44361, #14934, #22576, #23049, #40298, #44139, #37191, #12045, #7481, #37419, #30282, #36729, #287, #19209, #15172, #25949, #22333, #744, #30049, #5542, #16577, #31207, #46020, #1456, #8904, #9625, #42181, #5300, #41458, #45779, #12988, #38606, #20625, #2407, #39765, #24468, #14402, #17506, #3119, #39300, #46258, #6233, #28809, #46493, #3370, #28310, #10819, #21823, #6475, #37364, #15594, #37134, #44781, #41170, #18916, #37612, #44310, #18680, #26135, #32866, #25669, #22050, #33575, #15345, #29998, #18456, #226, #11283, #40939, #8135, #42379, #12478, #5732, #16301, #20347, #45731, #34754, #1896, #45969, #1175, #12228, #31161, #30458, #41412, #27101, #27819, #37863, #5017, #19637, #16068, #8856, #43319, #6897, #20811, #36155, #2821, #3308, #2592, #6424, #28039, #14347, #43076, #28996, #31632, #10281, #46442, #38798, #35220, #42824, #10037, #39487, #6664, #42599, #18442, #29038, #17732, #24935, #19330, #33979, #29523, #32382, #7188, #32855, #3822, #13904, #32621, #33093, #28796, #43360, #43839, #10567, #14152, #10808, #46963, #28551, #43119, #214, #47208, #11271, #14864, #25169, #10323, #18213, #39753, #36203, #6943, #25421, #7648, #39528, #21565, #6707, #14621, #11040, #4699, #14388, #43597, #25655, #21320, #21813, #3355, #40231, #44074, #25883, #22038, #7420, #36441, #36664, #39995, #47449, #17967, #3107, #3593, #29291, #40465, #22929, #37540, #35951, #13113, #4942, #19569, #31094, #12873, #45185, #45655, #38253, #27507, #45898, #19799, #9019, #34213, #42058, #23640, #9261, #27746, #38492, #38729, #1578, #12406, #34431, #5898, #1343, #27028, #23880, #5661, #15997, #34917, #16229, #20510, #34675, #20269, #30621, #2061, #16693, #31321, #8780, #42311, #9503, #8540, #5179, #1106, #5415, #30863, #24124, #15765, #45425, #41340, #12642, #27268, #41577, #41817, #30397, #44946, #23417, #20034, #12157, #26781, #23173, #37790, #38019, #1822, #16458, #30716, #2156, #42402, #19896, #35008, #1683, #38345, #27371, #42157, #1206, #37887, #9365, #1922, #23271, #37643, #16329, #19665, #5045, #34078, #34307, #45757, #1434, #38587, #41913, #5521 ) ),
 .UNSPECIFIED., .F., .F., .T. ) 
 B_SPLINE_SURFACE_WITH_KNOTS ( ( 2, 2 ),
 ( 3, 2, 2, 2, 2, 2, 2, 2, 2, 2, 2, 2, 2, 2, 2, 2, 2, 2, 2, 2, 2, 2, 2, 2, 2, 2, 2, 2, 2, 2, 2, 2, 2, 2, 2, 2, 2, 2, 2, 2, 2, 2, 2, 2, 2, 2, 2, 2, 2, 2, 2, 2, 2, 2, 2, 2, 2, 2, 2, 2, 2, 2, 2, 2, 2, 2, 2, 2, 2, 2, 2, 2, 2, 2, 2, 2, 2, 2, 2, 2, 2, 2, 2, 2, 2, 2, 2, 2, 2, 2, 2, 2, 2, 2, 2, 2, 2, 2, 2, 2, 2, 2, 2, 2, 2, 2, 2, 2, 2, 2, 2, 2, 2, 2, 2, 2, 2, 2, 2, 2, 2, 2, 2, 2, 2, 2, 2, 2, 2, 2, 2, 2, 2, 2, 2, 2, 2, 2, 2, 2, 2, 2, 2, 2, 2, 2, 2, 2, 2, 2, 2, 2, 2, 2, 2, 2, 2, 2, 2, 2, 2, 2, 2, 2, 2, 2, 2, 2, 2, 2, 2, 2, 2, 2, 2, 2, 2, 2, 2, 2, 2, 2, 2, 2, 2, 2, 2, 2, 2, 2, 2, 2, 2, 2, 2, 2, 2, 2, 2, 2, 2, 2, 2, 2, 2, 2, 2, 2, 2, 2, 2, 2, 2, 2, 2, 2, 2, 2, 2, 2, 2, 2, 2, 2, 2, 2, 2, 2, 2, 2, 2, 2, 2, 2, 2, 2, 2, 2, 2, 2, 2, 2, 2, 2, 2, 2, 2, 2, 2, 2, 2, 2, 2, 2, 2, 2, 2, 2, 2, 2, 2, 2, 2, 2, 2, 2, 2, 2, 2, 2, 2, 2, 2, 2, 2, 2, 2, 2, 2, 2, 2, 2, 2, 2, 2, 2, 2, 2, 2, 2, 2, 2, 2, 2, 2, 2, 2, 2, 2, 2, 2, 2, 2, 2, 2, 2, 2, 2, 2, 2, 2, 2, 2, 2, 2, 2, 2, 2, 2, 2, 2, 2, 2, 2, 2, 2, 2, 2, 2, 2, 2, 2, 2, 2, 2, 2, 2, 2, 2, 2, 2, 2, 2, 2, 2, 2, 2, 2, 2, 2, 2, 2, 2, 2, 2, 2, 2, 2, 2, 2, 2, 2, 2, 2, 2, 2, 2, 2, 2, 2, 2, 2, 2, 2, 2, 2, 2, 2, 2, 2, 2, 2, 2, 2, 2, 2, 2, 2, 2, 2, 2, 2, 2, 2, 2, 2, 2, 2, 2, 2, 3 ),
 ( 0.000000000000000000, 1.000000000000000000 ),
 ( 0.000000000000000000, 0.002500000000000000052, 0.005000000000000000104, 0.007499999999999999722, 0.01000000000000000021, 0.01250000000000000069, 0.01499999999999999944, 0.01750000000000000167, 0.02000000000000000042, 0.02249999999999999917, 0.02500000000000000139, 0.02750000000000000014, 0.02999999999999999889, 0.03250000000000000111, 0.03500000000000000333, 0.03749999999999999861, 0.04000000000000000083, 0.04250000000000000305, 0.04499999999999999833, 0.04750000000000000056, 0.05000000000000000278, 0.05249999999999999806, 0.05500000000000000028, 0.05750000000000000250, 0.05999999999999999778, 0.06250000000000000000, 0.06500000000000000222, 0.06750000000000000444, 0.07000000000000000666, 0.07249999999999999500, 0.07499999999999999722, 0.07749999999999999944, 0.08000000000000000167, 0.08250000000000000389, 0.08500000000000000611, 0.08749999999999999445, 0.08999999999999999667, 0.09249999999999999889, 0.09500000000000000111, 0.09750000000000000333, 0.1000000000000000056, 0.1024999999999999939, 0.1049999999999999961, 0.1074999999999999983, 0.1100000000000000006, 0.1125000000000000028, 0.1150000000000000050, 0.1174999999999999933, 0.1199999999999999956, 0.1224999999999999978, 0.1250000000000000000, 0.1275000000000000022, 0.1300000000000000044, 0.1325000000000000067, 0.1350000000000000089, 0.1375000000000000111, 0.1400000000000000133, 0.1424999999999999878, 0.1449999999999999900, 0.1474999999999999922, 0.1499999999999999944, 0.1524999999999999967, 0.1549999999999999989, 0.1575000000000000011, 0.1600000000000000033, 0.1625000000000000056, 0.1650000000000000078, 0.1675000000000000100, 0.1700000000000000122, 0.1724999999999999867, 0.1749999999999999889, 0.1774999999999999911, 0.1799999999999999933, 0.1824999999999999956, 0.1849999999999999978, 0.1875000000000000000, 0.1900000000000000022, 0.1925000000000000044, 0.1950000000000000067, 0.1975000000000000089, 0.2000000000000000111, 0.2025000000000000133, 0.2049999999999999878, 0.2074999999999999900, 0.2099999999999999922, 0.2124999999999999944, 0.2149999999999999967, 0.2174999999999999989, 0.2200000000000000011, 0.2225000000000000033, 0.2250000000000000056, 0.2275000000000000078, 0.2300000000000000100, 0.2325000000000000122, 0.2349999999999999867, 0.2374999999999999889, 0.2399999999999999911, 0.2424999999999999933, 0.2449999999999999956, 0.2474999999999999978, 0.2500000000000000000, 0.2525000000000000022, 0.2550000000000000044, 0.2575000000000000067, 0.2600000000000000089, 0.2625000000000000111, 0.2650000000000000133, 0.2675000000000000155, 0.2700000000000000178, 0.2725000000000000200, 0.2750000000000000222, 0.2775000000000000244, 0.2800000000000000266, 0.2824999999999999734, 0.2849999999999999756, 0.2874999999999999778, 0.2899999999999999800, 0.2924999999999999822, 0.2949999999999999845, 0.2974999999999999867, 0.2999999999999999889, 0.3024999999999999911, 0.3049999999999999933, 0.3074999999999999956, 0.3099999999999999978, 0.3125000000000000000, 0.3150000000000000022, 0.3175000000000000044, 0.3200000000000000067, 0.3225000000000000089, 0.3250000000000000111, 0.3275000000000000133, 0.3300000000000000155, 0.3325000000000000178, 0.3350000000000000200, 0.3375000000000000222, 0.3400000000000000244, 0.3425000000000000266, 0.3449999999999999734, 0.3474999999999999756, 0.3499999999999999778, 0.3524999999999999800, 0.3549999999999999822, 0.3574999999999999845, 0.3599999999999999867, 0.3624999999999999889, 0.3649999999999999911, 0.3674999999999999933, 0.3699999999999999956, 0.3724999999999999978, 0.3750000000000000000, 0.3775000000000000022, 0.3800000000000000044, 0.3825000000000000067, 0.3850000000000000089, 0.3875000000000000111, 0.3900000000000000133, 0.3925000000000000155, 0.3950000000000000178, 0.3975000000000000200, 0.4000000000000000222, 0.4025000000000000244, 0.4050000000000000266, 0.4074999999999999734, 0.4099999999999999756, 0.4124999999999999778, 0.4149999999999999800, 0.4174999999999999822, 0.4199999999999999845, 0.4224999999999999867, 0.4249999999999999889, 0.4274999999999999911, 0.4299999999999999933, 0.4324999999999999956, 0.4349999999999999978, 0.4375000000000000000, 0.4400000000000000022, 0.4425000000000000044, 0.4450000000000000067, 0.4475000000000000089, 0.4500000000000000111, 0.4525000000000000133, 0.4550000000000000155, 0.4575000000000000178, 0.4600000000000000200, 0.4625000000000000222, 0.4650000000000000244, 0.4675000000000000266, 0.4699999999999999734, 0.4724999999999999756, 0.4749999999999999778, 0.4774999999999999800, 0.4799999999999999822, 0.4824999999999999845, 0.4849999999999999867, 0.4874999999999999889, 0.4899999999999999911, 0.4924999999999999933, 0.4949999999999999956, 0.4974999999999999978, 0.5000000000000000000, 0.5024999999999999467, 0.5050000000000000044, 0.5074999999999999512, 0.5100000000000000089, 0.5124999999999999556, 0.5150000000000000133, 0.5174999999999999600, 0.5200000000000000178, 0.5224999999999999645, 0.5250000000000000222, 0.5274999999999999689, 0.5300000000000000266, 0.5324999999999999734, 0.5350000000000000311, 0.5374999999999999778, 0.5400000000000000355, 0.5424999999999999822, 0.5450000000000000400, 0.5474999999999999867, 0.5500000000000000444, 0.5524999999999999911, 0.5550000000000000488, 0.5574999999999999956, 0.5600000000000000533, 0.5625000000000000000, 0.5649999999999999467, 0.5675000000000000044, 0.5699999999999999512, 0.5725000000000000089, 0.5749999999999999556, 0.5775000000000000133, 0.5799999999999999600, 0.5825000000000000178, 0.5849999999999999645, 0.5875000000000000222, 0.5899999999999999689, 0.5925000000000000266, 0.5949999999999999734, 0.5975000000000000311, 0.5999999999999999778, 0.6025000000000000355, 0.6049999999999999822, 0.6075000000000000400, 0.6099999999999999867, 0.6125000000000000444, 0.6149999999999999911, 0.6175000000000000488, 0.6199999999999999956, 0.6225000000000000533, 0.6250000000000000000, 0.6274999999999999467, 0.6300000000000000044, 0.6324999999999999512, 0.6350000000000000089, 0.6374999999999999556, 0.6400000000000000133, 0.6424999999999999600, 0.6450000000000000178, 0.6474999999999999645, 0.6500000000000000222, 0.6524999999999999689, 0.6550000000000000266, 0.6574999999999999734, 0.6600000000000000311, 0.6624999999999999778, 0.6650000000000000355, 0.6674999999999999822, 0.6700000000000000400, 0.6724999999999999867, 0.6750000000000000444, 0.6774999999999999911, 0.6800000000000000488, 0.6824999999999999956, 0.6850000000000000533, 0.6875000000000000000, 0.6899999999999999467, 0.6925000000000000044, 0.6949999999999999512, 0.6975000000000000089, 0.6999999999999999556, 0.7025000000000000133, 0.7049999999999999600, 0.7075000000000000178, 0.7099999999999999645, 0.7125000000000000222, 0.7149999999999999689, 0.7175000000000000266, 0.7199999999999999734, 0.7225000000000000311, 0.7249999999999999778, 0.7275000000000000355, 0.7299999999999999822, 0.7325000000000000400, 0.7349999999999999867, 0.7375000000000000444, 0.7399999999999999911, 0.7425000000000000488, 0.7449999999999999956, 0.7475000000000000533, 0.7500000000000000000, 0.7524999999999999467, 0.7550000000000000044, 0.7574999999999999512, 0.7600000000000000089, 0.7624999999999999556, 0.7650000000000000133, 0.7674999999999999600, 0.7700000000000000178, 0.7724999999999999645, 0.7750000000000000222, 0.7774999999999999689, 0.7800000000000000266, 0.7824999999999999734, 0.7850000000000000311, 0.7874999999999999778, 0.7900000000000000355, 0.7924999999999999822, 0.7950000000000000400, 0.7974999999999999867, 0.8000000000000000444, 0.8024999999999999911, 0.8050000000000000488, 0.8074999999999999956, 0.8100000000000000533, 0.8125000000000000000, 0.8149999999999999467, 0.8175000000000000044, 0.8199999999999999512, 0.8225000000000000089, 0.8249999999999999556, 0.8275000000000000133, 0.8299999999999999600, 0.8325000000000000178, 0.8349999999999999645, 0.8375000000000000222, 0.8399999999999999689, 0.8425000000000000266, 0.8449999999999999734, 0.8475000000000000311, 0.8499999999999999778, 0.8525000000000000355, 0.8549999999999999822, 0.8575000000000000400, 0.8599999999999999867, 0.8625000000000000444, 0.8649999999999999911, 0.8675000000000000488, 0.8699999999999999956, 0.8725000000000000533, 0.8750000000000000000, 0.8774999999999999467, 0.8800000000000000044, 0.8824999999999999512, 0.8850000000000000089, 0.8874999999999999556, 0.8900000000000000133, 0.8924999999999999600, 0.8950000000000000178, 0.8974999999999999645, 0.9000000000000000222, 0.9024999999999999689, 0.9050000000000000266, 0.9074999999999999734, 0.9100000000000000311, 0.9124999999999999778, 0.9150000000000000355, 0.9174999999999999822, 0.9200000000000000400, 0.9224999999999999867, 0.9250000000000000444, 0.9274999999999999911, 0.9300000000000000488, 0.9324999999999999956, 0.9350000000000000533, 0.9375000000000000000, 0.9399999999999999467, 0.9425000000000000044, 0.9449999999999999512, 0.9475000000000000089, 0.9499999999999999556, 0.9525000000000000133, 0.9549999999999999600, 0.9575000000000000178, 0.9599999999999999645, 0.9625000000000000222, 0.9649999999999999689, 0.9675000000000000266, 0.9699999999999999734, 0.9725000000000000311, 0.9749999999999999778, 0.9775000000000000355, 0.9799999999999999822, 0.9825000000000000400, 0.9849999999999999867, 0.9875000000000000444, 0.9899999999999999911, 0.9925000000000000488, 0.9949999999999999956, 0.9975000000000000533, 1.000000000000000000 ),
 .UNSPECIFIED. ) 
 GEOMETRIC_REPRESENTATION_ITEM ( )  RATIONAL_B_SPLINE_SURFACE ( (
 ( 1.000000000000000000, 0.9238795325112869605, 1.000000000000000000, 0.9238795325112869605, 1.000000000000000000, 0.9238795325112869605, 1.000000000000000000, 0.9238795325112869605, 1.000000000000000000, 0.9238795325112869605, 1.000000000000000000, 0.9238795325112869605, 1.000000000000000000, 0.9238795325112869605, 1.000000000000000000, 0.9238795325112869605, 1.000000000000000000, 0.9238795325112869605, 1.000000000000000000, 0.9238795325112869605, 1.000000000000000000, 0.9238795325112869605, 1.000000000000000000, 0.9238795325112869605, 1.000000000000000000, 0.9238795325112869605, 1.000000000000000000, 0.9238795325112869605, 1.000000000000000000, 0.9238795325112869605, 1.000000000000000000, 0.9238795325112869605, 1.000000000000000000, 0.9238795325112869605, 1.000000000000000000, 0.9238795325112869605, 1.000000000000000000, 0.9238795325112869605, 1.000000000000000000, 0.9238795325112869605, 1.000000000000000000, 0.9238795325112869605, 1.000000000000000000, 0.9238795325112869605, 1.000000000000000000, 0.9238795325112869605, 1.000000000000000000, 0.9238795325112869605, 1.000000000000000000, 0.9238795325112869605, 1.000000000000000000, 0.9238795325112869605, 1.000000000000000000, 0.9238795325112869605, 1.000000000000000000, 0.9238795325112869605, 1.000000000000000000, 0.9238795325112869605, 1.000000000000000000, 0.9238795325112869605, 1.000000000000000000, 0.9238795325112869605, 1.000000000000000000, 0.9238795325112869605, 1.000000000000000000, 0.9238795325112869605, 1.000000000000000000, 0.9238795325112869605, 1.000000000000000000, 0.9238795325112869605, 1.000000000000000000, 0.9238795325112869605, 1.000000000000000000, 0.9238795325112869605, 1.000000000000000000, 0.9238795325112869605, 1.000000000000000000, 0.9238795325112869605, 1.000000000000000000, 0.9238795325112869605, 1.000000000000000000, 0.9238795325112869605, 1.000000000000000000, 0.9238795325112869605, 1.000000000000000000, 0.9238795325112869605, 1.000000000000000000, 0.9238795325112869605, 1.000000000000000000, 0.9238795325112869605, 1.000000000000000000, 0.9238795325112869605, 1.000000000000000000, 0.9238795325112869605, 1.000000000000000000, 0.9238795325112869605, 1.000000000000000000, 0.9238795325112869605, 1.000000000000000000, 0.9238795325112869605, 1.000000000000000000, 0.9238795325112869605, 1.000000000000000000, 0.9238795325112869605, 1.000000000000000000, 0.9238795325112869605, 1.000000000000000000, 0.9238795325112869605, 1.000000000000000000, 0.9238795325112869605, 1.000000000000000000, 0.9238795325112869605, 1.000000000000000000, 0.9238795325112869605, 1.000000000000000000, 0.9238795325112869605, 1.000000000000000000, 0.9238795325112869605, 1.000000000000000000, 0.9238795325112869605, 1.000000000000000000, 0.9238795325112869605, 1.000000000000000000, 0.9238795325112869605, 1.000000000000000000, 0.9238795325112869605, 1.000000000000000000, 0.9238795325112869605, 1.000000000000000000, 0.9238795325112869605, 1.000000000000000000, 0.9238795325112869605, 1.000000000000000000, 0.9238795325112869605, 1.000000000000000000, 0.9238795325112869605, 1.000000000000000000, 0.9238795325112869605, 1.000000000000000000, 0.9238795325112869605, 1.000000000000000000, 0.9238795325112869605, 1.000000000000000000, 0.9238795325112869605, 1.000000000000000000, 0.9238795325112869605, 1.000000000000000000, 0.9238795325112869605, 1.000000000000000000, 0.9238795325112869605, 1.000000000000000000, 0.9238795325112869605, 1.000000000000000000, 0.9238795325112869605, 1.000000000000000000, 0.9238795325112869605, 1.000000000000000000, 0.9238795325112869605, 1.000000000000000000, 0.9238795325112869605, 1.000000000000000000, 0.9238795325112869605, 1.000000000000000000, 0.9238795325112869605, 1.000000000000000000, 0.9238795325112869605, 1.000000000000000000, 0.9238795325112869605, 1.000000000000000000, 0.9238795325112869605, 1.000000000000000000, 0.9238795325112869605, 1.000000000000000000, 0.9238795325112869605, 1.000000000000000000, 0.9238795325112869605, 1.000000000000000000, 0.9238795325112869605, 1.000000000000000000, 0.9238795325112869605, 1.000000000000000000, 0.9238795325112869605, 1.000000000000000000, 0.9238795325112869605, 1.000000000000000000, 0.9238795325112869605, 1.000000000000000000, 0.9238795325112869605, 1.000000000000000000, 0.9238795325112869605, 1.000000000000000000, 0.9238795325112869605, 1.000000000000000000, 0.9238795325112869605, 1.000000000000000000, 0.9238795325112869605, 1.000000000000000000, 0.9238795325112869605, 1.000000000000000000, 0.9238795325112869605, 1.000000000000000000, 0.9238795325112869605, 1.000000000000000000, 0.9238795325112869605, 1.000000000000000000, 0.9238795325112869605, 1.000000000000000000, 0.9238795325112869605, 1.000000000000000000, 0.9238795325112869605, 1.000000000000000000, 0.9238795325112869605, 1.000000000000000000, 0.9238795325112869605, 1.000000000000000000, 0.9238795325112869605, 1.000000000000000000, 0.9238795325112869605, 1.000000000000000000, 0.9238795325112869605, 1.000000000000000000, 0.9238795325112869605, 1.000000000000000000, 0.9238795325112869605, 1.000000000000000000, 0.9238795325112869605, 1.000000000000000000, 0.9238795325112869605, 1.000000000000000000, 0.9238795325112869605, 1.000000000000000000, 0.9238795325112869605, 1.000000000000000000, 0.9238795325112869605, 1.000000000000000000, 0.9238795325112869605, 1.000000000000000000, 0.9238795325112869605, 1.000000000000000000, 0.9238795325112869605, 1.000000000000000000, 0.9238795325112869605, 1.000000000000000000, 0.9238795325112869605, 1.000000000000000000, 0.9238795325112869605, 1.000000000000000000, 0.9238795325112869605, 1.000000000000000000, 0.9238795325112869605, 1.000000000000000000, 0.9238795325112869605, 1.000000000000000000, 0.9238795325112869605, 1.000000000000000000, 0.9238795325112869605, 1.000000000000000000, 0.9238795325112869605, 1.000000000000000000, 0.9238795325112869605, 1.000000000000000000, 0.9238795325112869605, 1.000000000000000000, 0.9238795325112869605, 1.000000000000000000, 0.9238795325112869605, 1.000000000000000000, 0.9238795325112869605, 1.000000000000000000, 0.9238795325112869605, 1.000000000000000000, 0.9238795325112869605, 1.000000000000000000, 0.9238795325112869605, 1.000000000000000000, 0.9238795325112869605, 1.000000000000000000, 0.9238795325112869605, 1.000000000000000000, 0.9238795325112869605, 1.000000000000000000, 0.9238795325112869605, 1.000000000000000000, 0.9238795325112869605, 1.000000000000000000, 0.9238795325112869605, 1.000000000000000000, 0.9238795325112869605, 1.000000000000000000, 0.9238795325112869605, 1.000000000000000000, 0.9238795325112869605, 1.000000000000000000, 0.9238795325112869605, 1.000000000000000000, 0.9238795325112869605, 1.000000000000000000, 0.9238795325112869605, 1.000000000000000000, 0.9238795325112869605, 1.000000000000000000, 0.9238795325112869605, 1.000000000000000000, 0.9238795325112869605, 1.000000000000000000, 0.9238795325112869605, 1.000000000000000000, 0.9238795325112869605, 1.000000000000000000, 0.9238795325112869605, 1.000000000000000000, 0.9238795325112869605, 1.000000000000000000, 0.9238795325112869605, 1.000000000000000000, 0.9238795325112869605, 1.000000000000000000, 0.9238795325112869605, 1.000000000000000000, 0.9238795325112869605, 1.000000000000000000, 0.9238795325112869605, 1.000000000000000000, 0.9238795325112869605, 1.000000000000000000, 0.9238795325112869605, 1.000000000000000000, 0.9238795325112869605, 1.000000000000000000, 0.9238795325112869605, 1.000000000000000000, 0.9238795325112869605, 1.000000000000000000, 0.9238795325112869605, 1.000000000000000000, 0.9238795325112869605, 1.000000000000000000, 0.9238795325112869605, 1.000000000000000000, 0.9238795325112869605, 1.000000000000000000, 0.9238795325112869605, 1.000000000000000000, 0.9238795325112869605, 1.000000000000000000, 0.9238795325112869605, 1.000000000000000000, 0.9238795325112869605, 1.000000000000000000, 0.9238795325112869605, 1.000000000000000000, 0.9238795325112869605, 1.000000000000000000, 0.9238795325112869605, 1.000000000000000000, 0.9238795325112869605, 1.000000000000000000, 0.9238795325112869605, 1.000000000000000000, 0.9238795325112869605, 1.000000000000000000, 0.9238795325112869605, 1.000000000000000000, 0.9238795325112869605, 1.000000000000000000, 0.9238795325112869605, 1.000000000000000000, 0.9238795325112869605, 1.000000000000000000, 0.9238795325112869605, 1.000000000000000000, 0.9238795325112869605, 1.000000000000000000, 0.9238795325112869605, 1.000000000000000000, 0.9238795325112869605, 1.000000000000000000, 0.9238795325112869605, 1.000000000000000000, 0.9238795325112869605, 1.000000000000000000, 0.9238795325112869605, 1.000000000000000000, 0.9238795325112869605, 1.000000000000000000, 0.9238795325112869605, 1.000000000000000000, 0.9238795325112869605, 1.000000000000000000, 0.9238795325112869605, 1.000000000000000000, 0.9238795325112869605, 1.000000000000000000, 0.9238795325112869605, 1.000000000000000000, 0.9238795325112869605, 1.000000000000000000, 0.9238795325112869605, 1.000000000000000000, 0.9238795325112869605, 1.000000000000000000, 0.9238795325112869605, 1.000000000000000000, 0.9238795325112869605, 1.000000000000000000, 0.9238795325112869605, 1.000000000000000000, 0.9238795325112869605, 1.000000000000000000, 0.9238795325112869605, 1.000000000000000000, 0.9238795325112869605, 1.000000000000000000, 0.9238795325112869605, 1.000000000000000000, 0.9238795325112869605, 1.000000000000000000, 0.9238795325112869605, 1.000000000000000000, 0.9238795325112869605, 1.000000000000000000, 0.9238795325112869605, 1.000000000000000000, 0.9238795325112869605, 1.000000000000000000, 0.9238795325112869605, 1.000000000000000000, 0.9238795325112869605, 1.000000000000000000, 0.9238795325112869605, 1.000000000000000000, 0.9238795325112869605, 1.000000000000000000, 0.9238795325112869605, 1.000000000000000000, 0.9238795325112869605, 1.000000000000000000, 0.9238795325112869605, 1.000000000000000000, 0.9238795325112869605, 1.000000000000000000, 0.9238795325112869605, 1.000000000000000000, 0.9238795325112869605, 1.000000000000000000, 0.9238795325112869605, 1.000000000000000000, 0.9238795325112869605, 1.000000000000000000, 0.9238795325112869605, 1.000000000000000000, 0.9238795325112869605, 1.000000000000000000, 0.9238795325112869605, 1.000000000000000000, 0.9238795325112869605, 1.000000000000000000, 0.9238795325112869605, 1.000000000000000000, 0.9238795325112869605, 1.000000000000000000, 0.9238795325112869605, 1.000000000000000000, 0.9238795325112869605, 1.000000000000000000, 0.9238795325112869605, 1.000000000000000000, 0.9238795325112869605, 1.000000000000000000, 0.9238795325112869605, 1.000000000000000000, 0.9238795325112869605, 1.000000000000000000, 0.9238795325112869605, 1.000000000000000000, 0.9238795325112869605, 1.000000000000000000, 0.9238795325112869605, 1.000000000000000000, 0.9238795325112869605, 1.000000000000000000, 0.9238795325112869605, 1.000000000000000000, 0.9238795325112869605, 1.000000000000000000, 0.9238795325112869605, 1.000000000000000000, 0.9238795325112869605, 1.000000000000000000, 0.9238795325112869605, 1.000000000000000000, 0.9238795325112869605, 1.000000000000000000, 0.9238795325112869605, 1.000000000000000000, 0.9238795325112869605, 1.000000000000000000, 0.9238795325112869605, 1.000000000000000000, 0.9238795325112869605, 1.000000000000000000, 0.9238795325112869605, 1.000000000000000000, 0.9238795325112869605, 1.000000000000000000, 0.9238795325112869605, 1.000000000000000000, 0.9238795325112869605, 1.000000000000000000, 0.9238795325112869605, 1.000000000000000000, 0.9238795325112869605, 1.000000000000000000, 0.9238795325112869605, 1.000000000000000000, 0.9238795325112869605, 1.000000000000000000, 0.9238795325112869605, 1.000000000000000000, 0.9238795325112869605, 1.000000000000000000, 0.9238795325112869605, 1.000000000000000000, 0.9238795325112869605, 1.000000000000000000, 0.9238795325112869605, 1.000000000000000000, 0.9238795325112869605, 1.000000000000000000, 0.9238795325112869605, 1.000000000000000000, 0.9238795325112869605, 1.000000000000000000, 0.9238795325112869605, 1.000000000000000000, 0.9238795325112869605, 1.000000000000000000, 0.9238795325112869605, 1.000000000000000000, 0.9238795325112869605, 1.000000000000000000, 0.9238795325112869605, 1.000000000000000000, 0.9238795325112869605, 1.000000000000000000, 0.9238795325112869605, 1.000000000000000000, 0.9238795325112869605, 1.000000000000000000, 0.9238795325112869605, 1.000000000000000000, 0.9238795325112869605, 1.000000000000000000, 0.9238795325112869605, 1.000000000000000000, 0.9238795325112869605, 1.000000000000000000, 0.9238795325112869605, 1.000000000000000000, 0.9238795325112869605, 1.000000000000000000, 0.9238795325112869605, 1.000000000000000000, 0.9238795325112869605, 1.000000000000000000, 0.9238795325112869605, 1.000000000000000000, 0.9238795325112869605, 1.000000000000000000, 0.9238795325112869605, 1.000000000000000000, 0.9238795325112869605, 1.000000000000000000, 0.9238795325112869605, 1.000000000000000000, 0.9238795325112869605, 1.000000000000000000, 0.9238795325112869605, 1.000000000000000000, 0.9238795325112869605, 1.000000000000000000, 0.9238795325112869605, 1.000000000000000000, 0.9238795325112869605, 1.000000000000000000, 0.9238795325112869605, 1.000000000000000000, 0.9238795325112869605, 1.000000000000000000, 0.9238795325112869605, 1.000000000000000000, 0.9238795325112869605, 1.000000000000000000, 0.9238795325112869605, 1.000000000000000000, 0.9238795325112869605, 1.000000000000000000, 0.9238795325112869605, 1.000000000000000000, 0.9238795325112869605, 1.000000000000000000, 0.9238795325112869605, 1.000000000000000000, 0.9238795325112869605, 1.000000000000000000, 0.9238795325112869605, 1.000000000000000000, 0.9238795325112869605, 1.000000000000000000, 0.9238795325112869605, 1.000000000000000000, 0.9238795325112869605, 1.000000000000000000, 0.9238795325112869605, 1.000000000000000000, 0.9238795325112869605, 1.000000000000000000, 0.9238795325112869605, 1.000000000000000000, 0.9238795325112869605, 1.000000000000000000, 0.9238795325112869605, 1.000000000000000000, 0.9238795325112869605, 1.000000000000000000, 0.9238795325112869605, 1.000000000000000000, 0.9238795325112869605, 1.000000000000000000, 0.9238795325112869605, 1.000000000000000000, 0.9238795325112869605, 1.000000000000000000, 0.9238795325112869605, 1.000000000000000000, 0.9238795325112869605, 1.000000000000000000, 0.9238795325112869605, 1.000000000000000000, 0.9238795325112869605, 1.000000000000000000, 0.9238795325112869605, 1.000000000000000000, 0.9238795325112869605, 1.000000000000000000, 0.9238795325112869605, 1.000000000000000000, 0.9238795325112869605, 1.000000000000000000, 0.9238795325112869605, 1.000000000000000000, 0.9238795325112869605, 1.000000000000000000, 0.9238795325112869605, 1.000000000000000000, 0.9238795325112869605, 1.000000000000000000, 0.9238795325112869605, 1.000000000000000000, 0.9238795325112869605, 1.000000000000000000, 0.9238795325112869605, 1.000000000000000000, 0.9238795325112869605, 1.000000000000000000, 0.9238795325112869605, 1.000000000000000000, 0.9238795325112869605, 1.000000000000000000, 0.9238795325112869605, 1.000000000000000000, 0.9238795325112869605, 1.000000000000000000, 0.9238795325112869605, 1.000000000000000000, 0.9238795325112869605, 1.000000000000000000, 0.9238795325112869605, 1.000000000000000000, 0.9238795325112869605, 1.000000000000000000, 0.9238795325112869605, 1.000000000000000000, 0.9238795325112869605, 1.000000000000000000, 0.9238795325112869605, 1.000000000000000000, 0.9238795325112869605, 1.000000000000000000, 0.9238795325112869605, 1.000000000000000000, 0.9238795325112869605, 1.000000000000000000, 0.9238795325112869605, 1.000000000000000000, 0.9238795325112869605, 1.000000000000000000, 0.9238795325112869605, 1.000000000000000000, 0.9238795325112869605, 1.000000000000000000, 0.9238795325112869605, 1.000000000000000000, 0.9238795325112869605, 1.000000000000000000, 0.9238795325112869605, 1.000000000000000000, 0.9238795325112869605, 1.000000000000000000, 0.9238795325112869605, 1.000000000000000000, 0.9238795325112869605, 1.000000000000000000, 0.9238795325112869605, 1.000000000000000000, 0.9238795325112869605, 1.000000000000000000, 0.9238795325112869605, 1.000000000000000000, 0.9238795325112869605, 1.000000000000000000, 0.9238795325112869605, 1.000000000000000000, 0.9238795325112869605, 1.000000000000000000, 0.9238795325112869605, 1.000000000000000000, 0.9238795325112869605, 1.000000000000000000, 0.9238795325112869605, 1.000000000000000000, 0.9238795325112869605, 1.000000000000000000, 0.9238795325112869605, 1.000000000000000000, 0.9238795325112869605, 1.000000000000000000, 0.9238795325112869605, 1.000000000000000000, 0.9238795325112869605, 1.000000000000000000, 0.9238795325112869605, 1.000000000000000000, 0.9238795325112869605, 1.000000000000000000, 0.9238795325112869605, 1.000000000000000000, 0.9238795325112869605, 1.000000000000000000, 0.9238795325112869605, 1.000000000000000000, 0.9238795325112869605, 1.000000000000000000, 0.9238795325112869605, 1.000000000000000000, 0.9238795325112869605, 1.000000000000000000, 0.9238795325112869605, 1.000000000000000000, 0.9238795325112869605, 1.000000000000000000, 0.9238795325112869605, 1.000000000000000000, 0.9238795325112869605, 1.000000000000000000, 0.9238795325112869605, 1.000000000000000000, 0.9238795325112869605, 1.000000000000000000, 0.9238795325112869605, 1.000000000000000000, 0.9238795325112869605, 1.000000000000000000, 0.9238795325112869605, 1.000000000000000000, 0.9238795325112869605, 1.000000000000000000, 0.9238795325112869605, 1.000000000000000000, 0.9238795325112869605, 1.000000000000000000, 0.9238795325112869605, 1.000000000000000000, 0.9238795325112869605, 1.000000000000000000, 0.9238795325112869605, 1.000000000000000000, 0.9238795325112869605, 1.000000000000000000, 0.9238795325112869605, 1.000000000000000000, 0.9238795325112869605, 1.000000000000000000, 0.9238795325112869605, 1.000000000000000000, 0.9238795325112869605, 1.000000000000000000, 0.9238795325112869605, 1.000000000000000000, 0.9238795325112869605, 1.000000000000000000),
 ( 1.000000000000000000, 0.9238795325112869605, 1.000000000000000000, 0.9238795325112869605, 1.000000000000000000, 0.9238795325112869605, 1.000000000000000000, 0.9238795325112869605, 1.000000000000000000, 0.9238795325112869605, 1.000000000000000000, 0.9238795325112869605, 1.000000000000000000, 0.9238795325112869605, 1.000000000000000000, 0.9238795325112869605, 1.000000000000000000, 0.9238795325112869605, 1.000000000000000000, 0.9238795325112869605, 1.000000000000000000, 0.9238795325112869605, 1.000000000000000000, 0.9238795325112869605, 1.000000000000000000, 0.9238795325112869605, 1.000000000000000000, 0.9238795325112869605, 1.000000000000000000, 0.9238795325112869605, 1.000000000000000000, 0.9238795325112869605, 1.000000000000000000, 0.9238795325112869605, 1.000000000000000000, 0.9238795325112869605, 1.000000000000000000, 0.9238795325112869605, 1.000000000000000000, 0.9238795325112869605, 1.000000000000000000, 0.9238795325112869605, 1.000000000000000000, 0.9238795325112869605, 1.000000000000000000, 0.9238795325112869605, 1.000000000000000000, 0.9238795325112869605, 1.000000000000000000, 0.9238795325112869605, 1.000000000000000000, 0.9238795325112869605, 1.000000000000000000, 0.9238795325112869605, 1.000000000000000000, 0.9238795325112869605, 1.000000000000000000, 0.9238795325112869605, 1.000000000000000000, 0.9238795325112869605, 1.000000000000000000, 0.9238795325112869605, 1.000000000000000000, 0.9238795325112869605, 1.000000000000000000, 0.9238795325112869605, 1.000000000000000000, 0.9238795325112869605, 1.000000000000000000, 0.9238795325112869605, 1.000000000000000000, 0.9238795325112869605, 1.000000000000000000, 0.9238795325112869605, 1.000000000000000000, 0.9238795325112869605, 1.000000000000000000, 0.9238795325112869605, 1.000000000000000000, 0.9238795325112869605, 1.000000000000000000, 0.9238795325112869605, 1.000000000000000000, 0.9238795325112869605, 1.000000000000000000, 0.9238795325112869605, 1.000000000000000000, 0.9238795325112869605, 1.000000000000000000, 0.9238795325112869605, 1.000000000000000000, 0.9238795325112869605, 1.000000000000000000, 0.9238795325112869605, 1.000000000000000000, 0.9238795325112869605, 1.000000000000000000, 0.9238795325112869605, 1.000000000000000000, 0.9238795325112869605, 1.000000000000000000, 0.9238795325112869605, 1.000000000000000000, 0.9238795325112869605, 1.000000000000000000, 0.9238795325112869605, 1.000000000000000000, 0.9238795325112869605, 1.000000000000000000, 0.9238795325112869605, 1.000000000000000000, 0.9238795325112869605, 1.000000000000000000, 0.9238795325112869605, 1.000000000000000000, 0.9238795325112869605, 1.000000000000000000, 0.9238795325112869605, 1.000000000000000000, 0.9238795325112869605, 1.000000000000000000, 0.9238795325112869605, 1.000000000000000000, 0.9238795325112869605, 1.000000000000000000, 0.9238795325112869605, 1.000000000000000000, 0.9238795325112869605, 1.000000000000000000, 0.9238795325112869605, 1.000000000000000000, 0.9238795325112869605, 1.000000000000000000, 0.9238795325112869605, 1.000000000000000000, 0.9238795325112869605, 1.000000000000000000, 0.9238795325112869605, 1.000000000000000000, 0.9238795325112869605, 1.000000000000000000, 0.9238795325112869605, 1.000000000000000000, 0.9238795325112869605, 1.000000000000000000, 0.9238795325112869605, 1.000000000000000000, 0.9238795325112869605, 1.000000000000000000, 0.9238795325112869605, 1.000000000000000000, 0.9238795325112869605, 1.000000000000000000, 0.9238795325112869605, 1.000000000000000000, 0.9238795325112869605, 1.000000000000000000, 0.9238795325112869605, 1.000000000000000000, 0.9238795325112869605, 1.000000000000000000, 0.9238795325112869605, 1.000000000000000000, 0.9238795325112869605, 1.000000000000000000, 0.9238795325112869605, 1.000000000000000000, 0.9238795325112869605, 1.000000000000000000, 0.9238795325112869605, 1.000000000000000000, 0.9238795325112869605, 1.000000000000000000, 0.9238795325112869605, 1.000000000000000000, 0.9238795325112869605, 1.000000000000000000, 0.9238795325112869605, 1.000000000000000000, 0.9238795325112869605, 1.000000000000000000, 0.9238795325112869605, 1.000000000000000000, 0.9238795325112869605, 1.000000000000000000, 0.9238795325112869605, 1.000000000000000000, 0.9238795325112869605, 1.000000000000000000, 0.9238795325112869605, 1.000000000000000000, 0.9238795325112869605, 1.000000000000000000, 0.9238795325112869605, 1.000000000000000000, 0.9238795325112869605, 1.000000000000000000, 0.9238795325112869605, 1.000000000000000000, 0.9238795325112869605, 1.000000000000000000, 0.9238795325112869605, 1.000000000000000000, 0.9238795325112869605, 1.000000000000000000, 0.9238795325112869605, 1.000000000000000000, 0.9238795325112869605, 1.000000000000000000, 0.9238795325112869605, 1.000000000000000000, 0.9238795325112869605, 1.000000000000000000, 0.9238795325112869605, 1.000000000000000000, 0.9238795325112869605, 1.000000000000000000, 0.9238795325112869605, 1.000000000000000000, 0.9238795325112869605, 1.000000000000000000, 0.9238795325112869605, 1.000000000000000000, 0.9238795325112869605, 1.000000000000000000, 0.9238795325112869605, 1.000000000000000000, 0.9238795325112869605, 1.000000000000000000, 0.9238795325112869605, 1.000000000000000000, 0.9238795325112869605, 1.000000000000000000, 0.9238795325112869605, 1.000000000000000000, 0.9238795325112869605, 1.000000000000000000, 0.9238795325112869605, 1.000000000000000000, 0.9238795325112869605, 1.000000000000000000, 0.9238795325112869605, 1.000000000000000000, 0.9238795325112869605, 1.000000000000000000, 0.9238795325112869605, 1.000000000000000000, 0.9238795325112869605, 1.000000000000000000, 0.9238795325112869605, 1.000000000000000000, 0.9238795325112869605, 1.000000000000000000, 0.9238795325112869605, 1.000000000000000000, 0.9238795325112869605, 1.000000000000000000, 0.9238795325112869605, 1.000000000000000000, 0.9238795325112869605, 1.000000000000000000, 0.9238795325112869605, 1.000000000000000000, 0.9238795325112869605, 1.000000000000000000, 0.9238795325112869605, 1.000000000000000000, 0.9238795325112869605, 1.000000000000000000, 0.9238795325112869605, 1.000000000000000000, 0.9238795325112869605, 1.000000000000000000, 0.9238795325112869605, 1.000000000000000000, 0.9238795325112869605, 1.000000000000000000, 0.9238795325112869605, 1.000000000000000000, 0.9238795325112869605, 1.000000000000000000, 0.9238795325112869605, 1.000000000000000000, 0.9238795325112869605, 1.000000000000000000, 0.9238795325112869605, 1.000000000000000000, 0.9238795325112869605, 1.000000000000000000, 0.9238795325112869605, 1.000000000000000000, 0.9238795325112869605, 1.000000000000000000, 0.9238795325112869605, 1.000000000000000000, 0.9238795325112869605, 1.000000000000000000, 0.9238795325112869605, 1.000000000000000000, 0.9238795325112869605, 1.000000000000000000, 0.9238795325112869605, 1.000000000000000000, 0.9238795325112869605, 1.000000000000000000, 0.9238795325112869605, 1.000000000000000000, 0.9238795325112869605, 1.000000000000000000, 0.9238795325112869605, 1.000000000000000000, 0.9238795325112869605, 1.000000000000000000, 0.9238795325112869605, 1.000000000000000000, 0.9238795325112869605, 1.000000000000000000, 0.9238795325112869605, 1.000000000000000000, 0.9238795325112869605, 1.000000000000000000, 0.9238795325112869605, 1.000000000000000000, 0.9238795325112869605, 1.000000000000000000, 0.9238795325112869605, 1.000000000000000000, 0.9238795325112869605, 1.000000000000000000, 0.9238795325112869605, 1.000000000000000000, 0.9238795325112869605, 1.000000000000000000, 0.9238795325112869605, 1.000000000000000000, 0.9238795325112869605, 1.000000000000000000, 0.9238795325112869605, 1.000000000000000000, 0.9238795325112869605, 1.000000000000000000, 0.9238795325112869605, 1.000000000000000000, 0.9238795325112869605, 1.000000000000000000, 0.9238795325112869605, 1.000000000000000000, 0.9238795325112869605, 1.000000000000000000, 0.9238795325112869605, 1.000000000000000000, 0.9238795325112869605, 1.000000000000000000, 0.9238795325112869605, 1.000000000000000000, 0.9238795325112869605, 1.000000000000000000, 0.9238795325112869605, 1.000000000000000000, 0.9238795325112869605, 1.000000000000000000, 0.9238795325112869605, 1.000000000000000000, 0.9238795325112869605, 1.000000000000000000, 0.9238795325112869605, 1.000000000000000000, 0.9238795325112869605, 1.000000000000000000, 0.9238795325112869605, 1.000000000000000000, 0.9238795325112869605, 1.000000000000000000, 0.9238795325112869605, 1.000000000000000000, 0.9238795325112869605, 1.000000000000000000, 0.9238795325112869605, 1.000000000000000000, 0.9238795325112869605, 1.000000000000000000, 0.9238795325112869605, 1.000000000000000000, 0.9238795325112869605, 1.000000000000000000, 0.9238795325112869605, 1.000000000000000000, 0.9238795325112869605, 1.000000000000000000, 0.9238795325112869605, 1.000000000000000000, 0.9238795325112869605, 1.000000000000000000, 0.9238795325112869605, 1.000000000000000000, 0.9238795325112869605, 1.000000000000000000, 0.9238795325112869605, 1.000000000000000000, 0.9238795325112869605, 1.000000000000000000, 0.9238795325112869605, 1.000000000000000000, 0.9238795325112869605, 1.000000000000000000, 0.9238795325112869605, 1.000000000000000000, 0.9238795325112869605, 1.000000000000000000, 0.9238795325112869605, 1.000000000000000000, 0.9238795325112869605, 1.000000000000000000, 0.9238795325112869605, 1.000000000000000000, 0.9238795325112869605, 1.000000000000000000, 0.9238795325112869605, 1.000000000000000000, 0.9238795325112869605, 1.000000000000000000, 0.9238795325112869605, 1.000000000000000000, 0.9238795325112869605, 1.000000000000000000, 0.9238795325112869605, 1.000000000000000000, 0.9238795325112869605, 1.000000000000000000, 0.9238795325112869605, 1.000000000000000000, 0.9238795325112869605, 1.000000000000000000, 0.9238795325112869605, 1.000000000000000000, 0.9238795325112869605, 1.000000000000000000, 0.9238795325112869605, 1.000000000000000000, 0.9238795325112869605, 1.000000000000000000, 0.9238795325112869605, 1.000000000000000000, 0.9238795325112869605, 1.000000000000000000, 0.9238795325112869605, 1.000000000000000000, 0.9238795325112869605, 1.000000000000000000, 0.9238795325112869605, 1.000000000000000000, 0.9238795325112869605, 1.000000000000000000, 0.9238795325112869605, 1.000000000000000000, 0.9238795325112869605, 1.000000000000000000, 0.9238795325112869605, 1.000000000000000000, 0.9238795325112869605, 1.000000000000000000, 0.9238795325112869605, 1.000000000000000000, 0.9238795325112869605, 1.000000000000000000, 0.9238795325112869605, 1.000000000000000000, 0.9238795325112869605, 1.000000000000000000, 0.9238795325112869605, 1.000000000000000000, 0.9238795325112869605, 1.000000000000000000, 0.9238795325112869605, 1.000000000000000000, 0.9238795325112869605, 1.000000000000000000, 0.9238795325112869605, 1.000000000000000000, 0.9238795325112869605, 1.000000000000000000, 0.9238795325112869605, 1.000000000000000000, 0.9238795325112869605, 1.000000000000000000, 0.9238795325112869605, 1.000000000000000000, 0.9238795325112869605, 1.000000000000000000, 0.9238795325112869605, 1.000000000000000000, 0.9238795325112869605, 1.000000000000000000, 0.9238795325112869605, 1.000000000000000000, 0.9238795325112869605, 1.000000000000000000, 0.9238795325112869605, 1.000000000000000000, 0.9238795325112869605, 1.000000000000000000, 0.9238795325112869605, 1.000000000000000000, 0.9238795325112869605, 1.000000000000000000, 0.9238795325112869605, 1.000000000000000000, 0.9238795325112869605, 1.000000000000000000, 0.9238795325112869605, 1.000000000000000000, 0.9238795325112869605, 1.000000000000000000, 0.9238795325112869605, 1.000000000000000000, 0.9238795325112869605, 1.000000000000000000, 0.9238795325112869605, 1.000000000000000000, 0.9238795325112869605, 1.000000000000000000, 0.9238795325112869605, 1.000000000000000000, 0.9238795325112869605, 1.000000000000000000, 0.9238795325112869605, 1.000000000000000000, 0.9238795325112869605, 1.000000000000000000, 0.9238795325112869605, 1.000000000000000000, 0.9238795325112869605, 1.000000000000000000, 0.9238795325112869605, 1.000000000000000000, 0.9238795325112869605, 1.000000000000000000, 0.9238795325112869605, 1.000000000000000000, 0.9238795325112869605, 1.000000000000000000, 0.9238795325112869605, 1.000000000000000000, 0.9238795325112869605, 1.000000000000000000, 0.9238795325112869605, 1.000000000000000000, 0.9238795325112869605, 1.000000000000000000, 0.9238795325112869605, 1.000000000000000000, 0.9238795325112869605, 1.000000000000000000, 0.9238795325112869605, 1.000000000000000000, 0.9238795325112869605, 1.000000000000000000, 0.9238795325112869605, 1.000000000000000000, 0.9238795325112869605, 1.000000000000000000, 0.9238795325112869605, 1.000000000000000000, 0.9238795325112869605, 1.000000000000000000, 0.9238795325112869605, 1.000000000000000000, 0.9238795325112869605, 1.000000000000000000, 0.9238795325112869605, 1.000000000000000000, 0.9238795325112869605, 1.000000000000000000, 0.9238795325112869605, 1.000000000000000000, 0.9238795325112869605, 1.000000000000000000, 0.9238795325112869605, 1.000000000000000000, 0.9238795325112869605, 1.000000000000000000, 0.9238795325112869605, 1.000000000000000000, 0.9238795325112869605, 1.000000000000000000, 0.9238795325112869605, 1.000000000000000000, 0.9238795325112869605, 1.000000000000000000, 0.9238795325112869605, 1.000000000000000000, 0.9238795325112869605, 1.000000000000000000, 0.9238795325112869605, 1.000000000000000000, 0.9238795325112869605, 1.000000000000000000, 0.9238795325112869605, 1.000000000000000000, 0.9238795325112869605, 1.000000000000000000, 0.9238795325112869605, 1.000000000000000000, 0.9238795325112869605, 1.000000000000000000, 0.9238795325112869605, 1.000000000000000000, 0.9238795325112869605, 1.000000000000000000, 0.9238795325112869605, 1.000000000000000000, 0.9238795325112869605, 1.000000000000000000, 0.9238795325112869605, 1.000000000000000000, 0.9238795325112869605, 1.000000000000000000, 0.9238795325112869605, 1.000000000000000000, 0.9238795325112869605, 1.000000000000000000, 0.9238795325112869605, 1.000000000000000000, 0.9238795325112869605, 1.000000000000000000, 0.9238795325112869605, 1.000000000000000000, 0.9238795325112869605, 1.000000000000000000, 0.9238795325112869605, 1.000000000000000000, 0.9238795325112869605, 1.000000000000000000, 0.9238795325112869605, 1.000000000000000000, 0.9238795325112869605, 1.000000000000000000, 0.9238795325112869605, 1.000000000000000000, 0.9238795325112869605, 1.000000000000000000, 0.9238795325112869605, 1.000000000000000000, 0.9238795325112869605, 1.000000000000000000, 0.9238795325112869605, 1.000000000000000000, 0.9238795325112869605, 1.000000000000000000, 0.9238795325112869605, 1.000000000000000000, 0.9238795325112869605, 1.000000000000000000, 0.9238795325112869605, 1.000000000000000000, 0.9238795325112869605, 1.000000000000000000, 0.9238795325112869605, 1.000000000000000000, 0.9238795325112869605, 1.000000000000000000, 0.9238795325112869605, 1.000000000000000000, 0.9238795325112869605, 1.000000000000000000, 0.9238795325112869605, 1.000000000000000000, 0.9238795325112869605, 1.000000000000000000, 0.9238795325112869605, 1.000000000000000000, 0.9238795325112869605, 1.000000000000000000, 0.9238795325112869605, 1.000000000000000000, 0.9238795325112869605, 1.000000000000000000, 0.9238795325112869605, 1.000000000000000000, 0.9238795325112869605, 1.000000000000000000, 0.9238795325112869605, 1.000000000000000000, 0.9238795325112869605, 1.000000000000000000, 0.9238795325112869605, 1.000000000000000000, 0.9238795325112869605, 1.000000000000000000, 0.9238795325112869605, 1.000000000000000000, 0.9238795325112869605, 1.000000000000000000, 0.9238795325112869605, 1.000000000000000000, 0.9238795325112869605, 1.000000000000000000, 0.9238795325112869605, 1.000000000000000000, 0.9238795325112869605, 1.000000000000000000, 0.9238795325112869605, 1.000000000000000000, 0.9238795325112869605, 1.000000000000000000, 0.9238795325112869605, 1.000000000000000000, 0.9238795325112869605, 1.000000000000000000, 0.9238795325112869605, 1.000000000000000000, 0.9238795325112869605, 1.000000000000000000, 0.9238795325112869605, 1.000000000000000000, 0.9238795325112869605, 1.000000000000000000, 0.9238795325112869605, 1.000000000000000000, 0.9238795325112869605, 1.000000000000000000, 0.9238795325112869605, 1.000000000000000000, 0.9238795325112869605, 1.000000000000000000, 0.9238795325112869605, 1.000000000000000000, 0.9238795325112869605, 1.000000000000000000, 0.9238795325112869605, 1.000000000000000000, 0.9238795325112869605, 1.000000000000000000, 0.9238795325112869605, 1.000000000000000000, 0.9238795325112869605, 1.000000000000000000, 0.9238795325112869605, 1.000000000000000000, 0.9238795325112869605, 1.000000000000000000, 0.9238795325112869605, 1.000000000000000000, 0.9238795325112869605, 1.000000000000000000, 0.9238795325112869605, 1.000000000000000000, 0.9238795325112869605, 1.000000000000000000, 0.9238795325112869605, 1.000000000000000000, 0.9238795325112869605, 1.000000000000000000, 0.9238795325112869605, 1.000000000000000000, 0.9238795325112869605, 1.000000000000000000, 0.9238795325112869605, 1.000000000000000000, 0.9238795325112869605, 1.000000000000000000, 0.9238795325112869605, 1.000000000000000000, 0.9238795325112869605, 1.000000000000000000, 0.9238795325112869605, 1.000000000000000000, 0.9238795325112869605, 1.000000000000000000, 0.9238795325112869605, 1.000000000000000000, 0.9238795325112869605, 1.000000000000000000, 0.9238795325112869605, 1.000000000000000000, 0.9238795325112869605, 1.000000000000000000, 0.9238795325112869605, 1.000000000000000000, 0.9238795325112869605, 1.000000000000000000, 0.9238795325112869605, 1.000000000000000000, 0.9238795325112869605, 1.000000000000000000, 0.9238795325112869605, 1.000000000000000000, 0.9238795325112869605, 1.000000000000000000, 0.9238795325112869605, 1.000000000000000000, 0.9238795325112869605, 1.000000000000000000, 0.9238795325112869605, 1.000000000000000000, 0.9238795325112869605, 1.000000000000000000, 0.9238795325112869605, 1.000000000000000000, 0.9238795325112869605, 1.000000000000000000) ) ) 
 REPRESENTATION_ITEM ( '' )  SURFACE ( )  ) ;
#34258=CARTESIAN_POINT ( 'NONE',  ( -0.1563239858028344920, -0.08956157449492478662, 0.05512560382421622523 ) ) ;
#34259=CARTESIAN_POINT ( 'NONE',  ( -1.094772975963752103E-17, -0.4827755904974173617, -0.1787899950787401882 ) ) ;
#34267=CARTESIAN_POINT ( 'NONE',  ( -1.094772975963752103E-17, -1.663877952702141672, -0.1787899950787401882 ) ) ;
#34268=CARTESIAN_POINT ( 'NONE',  ( 0.1264236179284866091, -0.9355314960092283583, 0.1264236179284866091 ) ) ;
#34269=CARTESIAN_POINT ( 'NONE',  ( 0.1113553986120547346, -1.272637795275590511, 0.1113553986120547346 ) ) ;
#34277=ORIENTED_EDGE ( 'NONE', *, *, #28957, .F. ) ;
#34297=CARTESIAN_POINT ( 'NONE',  ( -0.2190824202996543291, -0.09842519685039370636, 0.09088772691789900882 ) ) ;
#34301=CARTESIAN_POINT ( 'NONE',  ( -0.1787899950787401604, -0.9527559054580476694, -0.07405724077823318263 ) ) ;
#34302=CARTESIAN_POINT ( 'NONE',  ( 0.1787899950787401604, -1.006889763725763220, 0.07405724077823318263 ) ) ;
#34306=CARTESIAN_POINT ( 'NONE',  ( 0.1797182628040039087, -0.4119532584019430788, -0.07444174185955065859 ) ) ;
#34307=CARTESIAN_POINT ( 'NONE',  ( 0.06523048226347956391, -1.816437007766488421, 0.1574803149606297803 ) ) ;
#34308=CARTESIAN_POINT ( 'NONE',  ( -0.06523048226347956391, 0.09793307086614169710, 0.1574803149606297803 ) ) ;
#34316=CARTESIAN_POINT ( 'NONE',  ( -0.07405724077823318263, -0.4311023621509605386, 0.1787899950787401604 ) ) ;
#34318=CARTESIAN_POINT ( 'NONE',  ( -0.1787899950787401604, -1.218503936954111300, 0.07405724077823318263 ) ) ;
#34329=CARTESIAN_POINT ( 'NONE',  ( -0.1281275874986674834, -0.09843444007757132241, -0.1247355789481490590 ) ) ;
#34334=CARTESIAN_POINT ( 'NONE',  ( -0.1213179770789060835, -0.08931471071071625523, -0.1315292587780671485 ) ) ;
#34346=CARTESIAN_POINT ( 'NONE',  ( -1.094772975963752103E-17, -1.522269637520576868, -0.1787899950787401882 ) ) ;
#34349=CARTESIAN_POINT ( 'NONE',  ( -0.1264236179284866091, -0.3892716534895436786, 0.1264236179284866091 ) ) ;
#34355=CARTESIAN_POINT ( 'NONE',  ( -0.1787899950787401882, -1.777066929080094670, 0.000000000000000000 ) ) ;
#34359=CARTESIAN_POINT ( 'NONE',  ( 0.1574803149606300301, -0.7977362204724408601, 0.06523048226347956391 ) ) ;
#34360=CARTESIAN_POINT ( 'NONE',  ( 0.1797182628040039087, -1.637346959189346141, 0.07444174185955046430 ) ) ;
#34365=FACE_OUTER_BOUND ( 'NONE', #10021, .T. ) ;
#34368=CARTESIAN_POINT ( 'NONE',  ( 0.1574803149606299191, -0.8641732282389291697, -1.928577636452523993E-17 ) ) ;
#34369=CARTESIAN_POINT ( 'NONE',  ( 0.1787899950787401604, 0.05610236225848794223, -0.07405724077823318263 ) ) ;
#34382=CARTESIAN_POINT ( 'NONE',  ( 0.07405724077823318263, -1.331692913332063855, 0.1787899950787401604 ) ) ;
#34397=CARTESIAN_POINT ( 'NONE',  ( -0.06523048226347956391, 0.02903543317839319890, 0.1574803149606297803 ) ) ;
#34399=CARTESIAN_POINT ( 'NONE',  ( 0.000000000000000000, -0.09842519685039370636, 0.2471922904502826812 ) ) ;
#34401=CARTESIAN_POINT ( 'NONE',  ( -0.1787899950787401604, -1.042446802874906986, -0.07405724077823318263 ) ) ;
#34403=CARTESIAN_POINT ( 'NONE',  ( -0.07405724077823318263, 0.07086614178604697112, -0.1787899950787401604 ) ) ;
#34411=CARTESIAN_POINT ( 'NONE',  ( -0.1787899950787401882, -0.5565944881352126172, 0.000000000000000000 ) ) ;
#34415=CARTESIAN_POINT ( 'NONE',  ( -0.1797182628040039087, -1.145220974937376734, -0.07444174185955065859 ) ) ;
#34423=CARTESIAN_POINT ( 'NONE',  ( 0.1787899950787401604, 0.09547244099864542199, 0.07405724077823318263 ) ) ;
#34431=CARTESIAN_POINT ( 'NONE',  ( -0.06523048226347956391, -1.663877952648379788, 0.1574803149606297803 ) ) ;
#34436=CARTESIAN_POINT ( 'NONE',  ( 0.09072478486330262659, -0.09340956239926194449, 0.2330530577653585345 ) ) ;
#34437=CARTESIAN_POINT ( 'NONE',  ( -0.07405724077823318263, 0.1496062992663619862, -0.1787899950787401604 ) ) ;
#34442=CARTESIAN_POINT ( 'NONE',  ( 0.07405724077823318263, -1.513779527505292322, -0.1787899950787401604 ) ) ;
#34449=CARTESIAN_POINT ( 'NONE',  ( 0.1512627532823037080, 0.1257768396322719584, -0.06122819718290384294 ) ) ;
#34451=CARTESIAN_POINT ( 'NONE',  ( 0.07405724077823318263, -0.5552420784654592545, 0.1787899950787401604 ) ) ;
#34452=CARTESIAN_POINT ( 'NONE',  ( 0.1244665901409340580, -0.08956009715716832520, 0.1738892908116259906 ) ) ;
#34456=CARTESIAN_POINT ( 'NONE',  ( 0.1787899950787401604, -1.810163338307978265, 0.07405724077823318263 ) ) ;
#34462=CARTESIAN_POINT ( 'NONE',  ( 0.1264236179284866091, -1.447342519631275692, 0.1264236179284866091 ) ) ;
#34467=CARTESIAN_POINT ( 'NONE',  ( -0.1270800023317771588, -0.7441382977720216729, 0.1270800023317771588 ) ) ;
#34472=CARTESIAN_POINT ( 'NONE',  ( -0.1113553986120547346, -0.3769685039370078705, 0.1113553986120547346 ) ) ;
#34484=CARTESIAN_POINT ( 'NONE',  ( 0.1787899950787401882, -0.6107283464029291675, -2.189545951927503898E-17 ) ) ;
#34491=CARTESIAN_POINT ( 'NONE',  ( 0.07405724077823318263, -1.666338582623402953, -0.1787899950787401604 ) ) ;
#34492=CARTESIAN_POINT ( 'NONE',  ( 0.1787899950787401882, -0.9699803149068660924, -2.189545951927503898E-17 ) ) ;
#34493=CARTESIAN_POINT ( 'NONE',  ( -0.1113553986120547346, -1.331692913385826849, -0.1113553986120547346 ) ) ;
#34497=ORIENTED_EDGE ( 'NONE', *, *, #41444, .F. ) ;
#34515=CARTESIAN_POINT ( 'NONE',  ( 0.1947348203212858064, -0.09842519685039370636, -0.06116798660091043310 ) ) ;
#34520=CARTESIAN_POINT ( 'NONE',  ( 0.1787899950787401604, -0.9724409448281265966, 0.07405724077823318263 ) ) ;
#34522=CARTESIAN_POINT ( 'NONE',  ( -0.1787899950787401604, -1.105314960576158301, -0.07405724077823318263 ) ) ;
#34526=CARTESIAN_POINT ( 'NONE',  ( 0.1797182628040039365, -0.3750438095830456731, -2.200913952912460540E-17 ) ) ;
#34529=CARTESIAN_POINT ( 'NONE',  ( -9.642888182262618425E-18, 0.08070866141732284393, -0.1574803149606299191 ) ) ;
#34540=CARTESIAN_POINT ( 'NONE',  ( 0.07405724077823318263, -0.4901574802611972093, -0.1787899950787401604 ) ) ;
#34542=CARTESIAN_POINT ( 'NONE',  ( 0.1264236179284866091, -1.432578740103716664, -0.1264236179284866091 ) ) ;
#34545=EDGE_LOOP ( 'NONE', ( #4899, #46936, #5803, #1675, #46750, #4478, #27858 ) ) ;
#34552=CARTESIAN_POINT ( 'NONE',  ( 0.03929603434986066873, -0.09842483377092413332, -0.1744181471411035411 ) ) ;
#34558=AXIS2_PLACEMENT_3D ( 'NONE', #20081, #16504, #23685 ) ;
#34564=CARTESIAN_POINT ( 'NONE',  ( -0.09381437428497224618, -0.09851384883702854478, 0.2089447948460571025 ) ) ;
#34570=CARTESIAN_POINT ( 'NONE',  ( 3.284318927891251994E-17, -1.620694834370970616, 0.1787899950787401882 ) ) ;
#34573=CARTESIAN_POINT ( 'NONE',  ( -0.1264236179284866091, -0.5467519684501732646, 0.1264236179284866091 ) ) ;
#34579=CARTESIAN_POINT ( 'NONE',  ( 0.07405724077823318263, -0.2539370078202523584, -0.1787899950787401604 ) ) ;
#34584=CARTESIAN_POINT ( 'NONE',  ( 3.284318927891251994E-17, 0.1115886301959580773, 0.1787899950787401882 ) ) ;
#34585=CARTESIAN_POINT ( 'NONE',  ( -0.1787899950787401604, 0.1496062992663619862, -0.07405724077823318263 ) ) ;
#34590=AXIS2_PLACEMENT_3D ( 'NONE', #28846, #29575, #43889 ) ;
#34592=CARTESIAN_POINT ( 'NONE',  ( -0.1574803149606297803, -0.8125000000000006661, 0.06523048226347956391 ) ) ;
#34594=CARTESIAN_POINT ( 'NONE',  ( 0.07444174185955065859, -1.563528061551551218, 0.1797182628040039087 ) ) ;
#34596=CARTESIAN_POINT ( 'NONE',  ( -0.1574803149606300301, -0.05954724398696107507, -0.06523048226347956391 ) ) ;
#34597=CARTESIAN_POINT ( 'NONE',  ( 0.1113553986120547346, -0.4360236219397173318, 0.1113553986120547346 ) ) ;
#34598=CARTESIAN_POINT ( 'NONE',  ( 0.1787899950787401882, -0.4138779527021417826, -2.189545951927503898E-17 ) ) ;
#34608=CARTESIAN_POINT ( 'NONE',  ( 3.284318927891251994E-17, 0.004429133912031243958, 0.1787899950787401882 ) ) ;
#34619=CARTESIAN_POINT ( 'NONE',  ( -1.094772975963752103E-17, -1.314468503883243988, -0.1787899950787401882 ) ) ;
#34631=CARTESIAN_POINT ( 'NONE',  ( -0.09932472909908414416, -0.09575019180978999733, -0.2280862973330396448 ) ) ;
#34634=CARTESIAN_POINT ( 'NONE',  ( 0.1574803149606299191, -0.03740157469562260112, -1.928577636452523993E-17 ) ) ;
#34636=COLOUR_RGB ( '', 0.08235294, 0.09019608, 0.10196078) ;
#34640=CARTESIAN_POINT ( 'NONE',  ( 0.1264236179284866091, -1.133490109961521775, -0.1264236179284866091 ) ) ;
#34642=CARTESIAN_POINT ( 'NONE',  ( -0.1264236179284866091, -0.03494094482812625663, 0.1264236179284866091 ) ) ;
#34655=CARTESIAN_POINT ( 'NONE',  ( 0.1797182628040039365, -1.201815463126352457, -2.200913952912460540E-17 ) ) ;
#34675=CARTESIAN_POINT ( 'NONE',  ( 0.1574803149606300301, -1.688484251860975949, -0.06523048226347956391 ) ) ;
#34679=EDGE_LOOP ( 'NONE', ( #9091, #5410, #18299 ) ) ;
#34680=CARTESIAN_POINT ( 'NONE',  ( 0.05730322896416124856, -0.07836638817768049048, 0.2523490388730026401 ) ) ;
#34681=CARTESIAN_POINT ( 'NONE',  ( 0.1113553986120547346, -1.784448818897637734, 0.1113553986120547346 ) ) ;
#34689=CARTESIAN_POINT ( 'NONE',  ( 0.06523048226347956391, -0.3843503935932603421, -0.1574803149606300301 ) ) ;
#34690=CARTESIAN_POINT ( 'NONE',  ( 0.1787899950787401604, -1.484251968450174930, 0.07405724077823318263 ) ) ;
#34700=CARTESIAN_POINT ( 'NONE',  ( -0.1787899950787401604, -0.6438247556308137609, 0.07405724077823318263 ) ) ;
#34701=CARTESIAN_POINT ( 'NONE',  ( 0.1329235558887131852, -0.08956032744261475942, -0.1422831879104033415 ) ) ;
#34713=CONICAL_SURFACE ( 'NONE', #16339, 0.2471922904502826812, 0.5235987755982992597 ) ;
#34715=CARTESIAN_POINT ( 'NONE',  ( 0.07405724077823318263, -1.489173228292693718, 0.1787899950787401604 ) ) ;
#34720=CARTESIAN_POINT ( 'NONE',  ( -0.1797182628040039087, -0.6727800300554868107, -0.07444174185955065859 ) ) ;
#34725=CARTESIAN_POINT ( 'NONE',  ( 0.1574803149606300301, -0.4434055118110233340, 0.06523048226347956391 ) ) ;
#34739=CARTESIAN_POINT ( 'NONE',  ( 0.07405724077823318263, -0.5787401574265509385, 0.1787899950787401604 ) ) ;
#34746=CARTESIAN_POINT ( 'NONE',  ( 0.1264236179284866091, -1.668799212544661348, -0.1264236179284866091 ) ) ;
#34747=CARTESIAN_POINT ( 'NONE',  ( 0.1787899950787401604, -0.9724409448281265966, 0.07405724077823318263 ) ) ;
#34748=CARTESIAN_POINT ( 'NONE',  ( -0.1113553986120547346, -1.439960629921259949, 0.1113553986120547346 ) ) ;
#34754=CARTESIAN_POINT ( 'NONE',  ( -0.06523048226347956391, -1.363681102254677313, -0.1574803149606300301 ) ) ;
#34764=CARTESIAN_POINT ( 'NONE',  ( 0.03342428880116892626, -0.06208088008896735233, -0.2661310841544295425 ) ) ;
#34769=CARTESIAN_POINT ( 'NONE',  ( 0.1466781083505074856, -0.09842519685039370636, 0.1600438778087322766 ) ) ;
#34774=VERTEX_POINT ( 'NONE', #40355 ) ;
#34777=CARTESIAN_POINT ( 'NONE',  ( 0.1787899950787401604, -1.085629921206079374, -0.07405724077823318263 ) ) ;
#34778=CARTESIAN_POINT ( 'NONE',  ( -0.1787899950787401604, -1.218503936954111300, 0.07405724077823318263 ) ) ;
#34781=CARTESIAN_POINT ( 'NONE',  ( 0.1797182628040039087, -0.5349847544649350972, 0.07444174185955046430 ) ) ;
#34783=CARTESIAN_POINT ( 'NONE',  ( -0.06523048226347956391, 0.004429133858267709535, -0.1574803149606300301 ) ) ;
#34791=CARTESIAN_POINT ( 'NONE',  ( 0.07405724077823318263, -0.3868110235682837295, 0.1787899950787401604 ) ) ;
#34793=CARTESIAN_POINT ( 'NONE',  ( 0.1264236179284866091, -1.363681102308440973, 0.1264236179284866091 ) ) ;
#34797=VERTEX_POINT ( 'NONE', #4406 ) ;
#34806=CARTESIAN_POINT ( 'NONE',  ( 0.08940444365453828479, -0.09842526949101637612, -0.1548350272596675514 ) ) ;
#34817=CARTESIAN_POINT ( 'NONE',  ( 0.1141376464151068887, -0.09851384742766575164, 0.1860460344805917599 ) ) ;
#34825=CARTESIAN_POINT ( 'NONE',  ( -0.07405724077823318263, -0.6624015747493856576, 0.1787899950787401604 ) ) ;
#34830=CARTESIAN_POINT ( 'NONE',  ( 0.07405724077823318263, -0.7214566928596228834, -0.1787899950787401604 ) ) ;
#34833=CARTESIAN_POINT ( 'NONE',  ( -0.1787899950787401604, -0.05819483437097103251, -0.07405724077823318263 ) ) ;
#34834=CARTESIAN_POINT ( 'NONE',  ( 0.1264236179284866091, 0.1373031496600628232, -0.1264236179284866091 ) ) ;
#34840=CARTESIAN_POINT ( 'NONE',  ( 2.892866454678787531E-17, -0.8444881889763780070, 0.1574803149606299191 ) ) ;
#34842=CARTESIAN_POINT ( 'NONE',  ( -0.1797182628040039087, -1.578291841079108471, -0.07444174185955065859 ) ) ;
#34853=CARTESIAN_POINT ( 'NONE',  ( -0.1113553986120547346, -0.8494094487113701408, -0.1113553986120547346 ) ) ;
#34854=CARTESIAN_POINT ( 'NONE',  ( -0.07405724077823318263, 0.001968503990771400605, 0.1787899950787401604 ) ) ;
#34880=CARTESIAN_POINT ( 'NONE',  ( 0.06523048226347956391, -0.2022637794200320971, 0.1574803149606297803 ) ) ;
#34886=CARTESIAN_POINT ( 'NONE',  ( 0.1264236179284866091, -1.172860188701678963, -0.1264236179284866091 ) ) ;
#34888=CARTESIAN_POINT ( 'NONE',  ( -0.1264236179284866091, -0.04478346451316559534, -0.1264236179284866091 ) ) ;
#34896=CARTESIAN_POINT ( 'NONE',  ( 0.07405724077823318263, -0.6870078739619840391, -0.1787899950787401604 ) ) ;
#34899=CARTESIAN_POINT ( 'NONE',  ( -0.07444174185955065859, -1.214118612732652425, 0.1797182628040039087 ) ) ;
#34909=CARTESIAN_POINT ( 'NONE',  ( 0.1113553986120547346, -0.7509842518609763928, 0.1113553986120547346 ) ) ;
#34917=CARTESIAN_POINT ( 'NONE',  ( -9.642888182262618425E-18, -1.681102362097196767, -0.1574803149606299191 ) ) ;
#34922=CARTESIAN_POINT ( 'NONE',  ( 3.284318927891251994E-17, 0.1274606299750234428, 0.1787899950787401882 ) ) ;
#34927=CARTESIAN_POINT ( 'NONE',  ( -0.1787899950787401604, -1.617125984198204414, 0.07405724077823318263 ) ) ;
#34935=CARTESIAN_POINT ( 'NONE',  ( -1.094772975963752103E-17, -0.6561279052371122855, -0.1787899950787401882 ) ) ;
#34937=CARTESIAN_POINT ( 'NONE',  ( 0.1168315015349214586, -0.08956051179396516682, -0.1546330483755491980 ) ) ;
#34938=FACE_OUTER_BOUND ( 'NONE', #1549, .T. ) ;
#34945=CARTESIAN_POINT ( 'NONE',  ( -0.1787899950787401604, -1.543307086560409713, -0.07405724077823318263 ) ) ;
#34951=CARTESIAN_POINT ( 'NONE',  ( -0.07444174185955065859, -0.6777012898980057098, -0.1797182628040039087 ) ) ;
#34954=CARTESIAN_POINT ( 'NONE',  ( -0.1574803149606297803, -0.3794291338582678752, 0.06523048226347956391 ) ) ;
#34955=CARTESIAN_POINT ( 'NONE',  ( -0.1604642934754345052, -0.09842519685039373412, -0.07810648738970782379 ) ) ;
#34964=CARTESIAN_POINT ( 'NONE',  ( 0.1574803149606300301, -0.5910433069790869132, 0.06523048226347956391 ) ) ;
#34966=FACE_OUTER_BOUND ( 'NONE', #23310, .T. ) ;
#34968=CARTESIAN_POINT ( 'NONE',  ( 0.1264236179284866091, -0.5369094487651339120, 0.1264236179284866091 ) ) ;
#34974=CARTESIAN_POINT ( 'NONE',  ( -0.06655125492326575964, 0.08353766247255413335, -0.2470096859212868312 ) ) ;
#34976=CARTESIAN_POINT ( 'NONE',  ( 0.1264236179284866091, -1.757381889710015965, 0.1264236179284866091 ) ) ;
#34977=CARTESIAN_POINT ( 'NONE',  ( -0.07405724077823318263, -1.115157480261196987, -0.1787899950787401604 ) ) ;
#34978=CARTESIAN_POINT ( 'NONE',  ( -0.06523048226347956391, -1.358759842519685845, 0.1574803149606297803 ) ) ;
#34994=CARTESIAN_POINT ( 'NONE',  ( -0.1292751490962173455, 0.09842519685039369248, 0.2107960287359116613 ) ) ;
#34997=CARTESIAN_POINT ( 'NONE',  ( -0.07405724077823318263, -0.2058326296465617378, 0.1787899950787401604 ) ) ;
#34999=CARTESIAN_POINT ( 'NONE',  ( -0.02490719980953610274, -0.09842519685039370636, -0.1871115436693586709 ) ) ;
#35004=CARTESIAN_POINT ( 'NONE',  ( -0.07405724077823318263, -1.075787401521038689, -0.1787899950787401604 ) ) ;
#35005=CARTESIAN_POINT ( 'NONE',  ( -0.1264236179284866091, -1.255413385773007873, 0.1264236179284866091 ) ) ;
#35007=CARTESIAN_POINT ( 'NONE',  ( 0.1797182628040039087, -0.5300634946224150879, -0.07444174185955065859 ) ) ;
#35008=CARTESIAN_POINT ( 'NONE',  ( 2.892866454678787531E-17, -1.779527558947590515, 0.1574803149606299191 ) ) ;
#35011=CARTESIAN_POINT ( 'NONE',  ( -0.1574803149606299191, 0.05118110236220472370, 0.000000000000000000 ) ) ;
#35017=CARTESIAN_POINT ( 'NONE',  ( 0.1787899950787401604, -0.6181102361667089040, 0.07405724077823318263 ) ) ;
#35020=CARTESIAN_POINT ( 'NONE',  ( 0.1264236179284866091, -1.403051181048598384, 0.1264236179284866091 ) ) ;
#35021=AXIS2_PLACEMENT_3D ( 'NONE', #6654, #24409, #36079 ) ;
#35036=EDGE_CURVE ( 'NONE', #34797, #799, #42261, .T. ) ;
#35043=CARTESIAN_POINT ( 'NONE',  ( 0.05863737992348047601, -0.09851384783664468570, 0.2134933313796791299 ) ) ;
#35050=CARTESIAN_POINT ( 'NONE',  ( 3.284318927891251994E-17, -0.6205708660879685201, 0.1787899950787401882 ) ) ;
#35055=CARTESIAN_POINT ( 'NONE',  ( 0.1787899950787401604, -0.7657480314423001921, -0.07405724077823318263 ) ) ;
#35058=CARTESIAN_POINT ( 'NONE',  ( 0.07405724077823318263, 0.03530910263690301143, 0.1787899950787401604 ) ) ;
#35059=CARTESIAN_POINT ( 'NONE',  ( 3.284318927891251994E-17, 0.08316929139234625901, 0.1787899950787401882 ) ) ;
#35061=CARTESIAN_POINT ( 'NONE',  ( -0.01002589960738839783, -0.09842519685039363697, 0.1604807810695956793 ) ) ;
#35064=EDGE_CURVE ( 'NONE', #10382, #40254, #21662, .T. ) ;
#35065=CARTESIAN_POINT ( 'NONE',  ( -0.1574803149606299191, -0.9330708661417322913, 0.000000000000000000 ) ) ;
#35067=CARTESIAN_POINT ( 'NONE',  ( -0.1797182628040039365, -1.575831211157848299, 0.000000000000000000 ) ) ;
#35071=CARTESIAN_POINT ( 'NONE',  ( 0.1235961452251413406, 0.09842519685039370636, -0.2140748031496062798 ) ) ;
#35079=CARTESIAN_POINT ( 'NONE',  ( 2.892866454678787531E-17, -0.8740157479239685223, 0.1574803149606299191 ) ) ;
#35080=CARTESIAN_POINT ( 'NONE',  ( 0.07405724077823318263, -0.03248031490686641154, 0.1787899950787401604 ) ) ;
#35082=CARTESIAN_POINT ( 'NONE',  ( -0.1787899950787401882, -0.03986220467064590517, 0.000000000000000000 ) ) ;
#35084=CARTESIAN_POINT ( 'NONE',  ( 0.1264236179284866091, -0.9995078739619842612, -0.1264236179284866091 ) ) ;
#35091=CARTESIAN_POINT ( 'NONE',  ( -0.06523048226347956391, -1.088090551073574996, -0.1574803149606300301 ) ) ;
#35103=CONICAL_SURFACE ( 'NONE', #18986, 0.2471922904502826812, 0.5235987755982992597 ) ;
#35104=CARTESIAN_POINT ( 'NONE',  ( 0.1787899950787401882, 0.09301181107738563936, -2.189545951927503898E-17 ) ) ;
#35113=CARTESIAN_POINT ( 'NONE',  ( -0.1264236179284866091, -1.153175149331600480, 0.1264236179284866091 ) ) ;
#35115=CARTESIAN_POINT ( 'NONE',  ( -0.1787899950787401882, -0.1973425196312759700, 0.000000000000000000 ) ) ;
#35116=ORIENTED_EDGE ( 'NONE', *, *, #35064, .T. ) ;
#35121=CARTESIAN_POINT ( 'NONE',  ( -0.1264236179284866091, -0.6304133857730078727, 0.1264236179284866091 ) ) ;
#35128=CARTESIAN_POINT ( 'NONE',  ( -1.100456976456230270E-17, -1.231343022181470293, -0.1797182628040039365 ) ) ;
#35139=CARTESIAN_POINT ( 'NONE',  ( 0.000000000000000000, 0.09842519685039370636, 0.2471922904502826812 ) ) ;
#35147=CARTESIAN_POINT ( 'NONE',  ( -0.07405724077823318263, -0.08661417317458304510, -0.1787899950787401604 ) ) ;
#35151=CARTESIAN_POINT ( 'NONE',  ( 0.06523048226347956391, -1.772145669291338654, -0.1574803149606300301 ) ) ;
#35153=AXIS2_PLACEMENT_3D ( 'NONE', #45528, #30730, #12035 ) ;
#35159=CARTESIAN_POINT ( 'NONE',  ( -0.1787899950787401604, -1.656496062938362268, 0.07405724077823318263 ) ) ;
#35168=CARTESIAN_POINT ( 'NONE',  ( 0.1405684605170431090, -0.08956022275308050951, -0.1355147671057568837 ) ) ;
#35183=CARTESIAN_POINT ( 'NONE',  ( -0.1270800023317771588, -0.7047682190318641515, 0.1270800023317771588 ) ) ;
#35186=CARTESIAN_POINT ( 'NONE',  ( 0.1574803149606299191, -0.3622047244094488416, -1.928577636452523993E-17 ) ) ;
#35187=CARTESIAN_POINT ( 'NONE',  ( -0.1683020774058382463, -0.09842519685039370636, 0.03867328716997087829 ) ) ;
#35191=CARTESIAN_POINT ( 'NONE',  ( 0.06523048226347956391, 0.02411417322834644855, 0.1574803149606297803 ) ) ;
#35201=CARTESIAN_POINT ( 'NONE',  ( -0.1239754358329518830, -0.08954324691734161235, -0.1284353226271238435 ) ) ;
#35202=CARTESIAN_POINT ( 'NONE',  ( -0.07405724077823318263, -0.5590551180564723444, -0.1787899950787401604 ) ) ;
#35209=CARTESIAN_POINT ( 'NONE',  ( -0.07600661141688493105, 0.08819060268786639567, -0.2415506333044120379 ) ) ;
#35211=CARTESIAN_POINT ( 'NONE',  ( 0.1270800023317771588, 0.1416884738815214761, -0.1270800023317771588 ) ) ;
#35212=CARTESIAN_POINT ( 'NONE',  ( 0.1264236179284866091, -1.132381889710015743, 0.1264236179284866091 ) ) ;
#35213=CARTESIAN_POINT ( 'NONE',  ( 0.06523048226347956391, -1.299704724409448398, -0.1574803149606300301 ) ) ;
#35220=CARTESIAN_POINT ( 'NONE',  ( -0.1113553986120547346, -1.439960629813732185, -0.1113553986120547346 ) ) ;
#35222=B_SPLINE_CURVE_WITH_KNOTS ( 'NONE', 3,
 ( #44262, #40893, #8086, #15068, #15293, #22226, #11235, #29489, #4464, #33770, #18176, #7611, #36859, #18633, #14584, #29945, #29258, #44490, #26079, #19105 ),
 .UNSPECIFIED., .F., .F.,
 ( 4, 1, 1, 1, 1, 1, 2, 2, 1, 1, 1, 2, 2, 4 ),
 ( 0.000000000000000000, 0.2499999999999991118, 0.3749999999999987232, 0.4374999999999983347, 0.4687499999999982792, 0.4843749999999981681, 0.4921874999999980016, 0.4999999999999977796, 0.6249999999999977796, 0.6874999999999978906, 0.7187499999999981126, 0.7343749999999981126, 0.7499999999999982236, 1.000000000000000000 ),
 .UNSPECIFIED. ) ;
#35232=CARTESIAN_POINT ( 'NONE',  ( 0.05467468201772719694, -0.07678538764759434976, -0.2538665577330192491 ) ) ;
#35235=CARTESIAN_POINT ( 'NONE',  ( 3.284318927891251994E-17, -0.2821121572056168869, 0.1787899950787401882 ) ) ;
#35236=CARTESIAN_POINT ( 'NONE',  ( 0.1908586082815771912, -0.09842519685039370636, -0.07077711205430314845 ) ) ;
#35243=CARTESIAN_POINT ( 'NONE',  ( 0.1787899950787401604, -1.046259842465921297, -0.07405724077823318263 ) ) ;
#35244=CARTESIAN_POINT ( 'NONE',  ( 0.1787899950787401604, -1.198818897584032150, -0.07405724077823318263 ) ) ;
#35247=CARTESIAN_POINT ( 'NONE',  ( -0.1797182628040039365, -0.5522091639137544083, 0.000000000000000000 ) ) ;
#35251=CARTESIAN_POINT ( 'NONE',  ( 0.1574803149606299191, 0.07086614173228346358, -1.928577636452523993E-17 ) ) ;
#35264=CARTESIAN_POINT ( 'NONE',  ( 0.07405724077823318263, -0.6624015747493856576, 0.1787899950787401604 ) ) ;
#35266=CARTESIAN_POINT ( 'NONE',  ( 0.1264236179284866091, -1.353838582623401621, -0.1264236179284866091 ) ) ;
#35277=CARTESIAN_POINT ( 'NONE',  ( 0.1235961452251413406, -0.09842519685039370636, 0.2140748031496062798 ) ) ;
#35284=CARTESIAN_POINT ( 'NONE',  ( 0.1643129700501710921, -0.09851384408417600269, -0.1153281366345470377 ) ) ;
#35289=CARTESIAN_POINT ( 'NONE',  ( -0.1787899950787401604, -1.554257826496955097, -0.07405724077823318263 ) ) ;
#35291=CARTESIAN_POINT ( 'NONE',  ( -0.07405724077823318263, -0.6377952755367874982, -0.1787899950787401604 ) ) ;
#35295=CARTESIAN_POINT ( 'NONE',  ( -0.1264236179284866091, -0.2760826771115909573, 0.1264236179284866091 ) ) ;
#35296=CARTESIAN_POINT ( 'NONE',  ( 0.07405724077823318263, -0.7608267715997808489, -0.1787899950787401604 ) ) ;
#35300=CARTESIAN_POINT ( 'NONE',  ( 0.1787899950787401604, 0.0008602837392652073079, 0.07405724077823318263 ) ) ;
#35301=CARTESIAN_POINT ( 'NONE',  ( -0.07405724077823318263, 0.02657480320336980464, -0.1787899950787401604 ) ) ;
#35303=CARTESIAN_POINT ( 'NONE',  ( 0.1033725344634994631, -0.09842519685039372024, 0.1327416431847782963 ) ) ;
#35307=CARTESIAN_POINT ( 'NONE',  ( -9.642888182262618425E-18, -0.9429133858267716439, -0.1574803149606299191 ) ) ;
#35309=CARTESIAN_POINT ( 'NONE',  ( 0.1270800023317771588, -1.718547746590919356, 0.1270800023317771588 ) ) ;
#35316=CARTESIAN_POINT ( 'NONE',  ( -0.1588219152425539016, -0.09266989036297289262, -0.1937372027062211621 ) ) ;
#35319=CARTESIAN_POINT ( 'NONE',  ( 0.1264236179284866091, -0.1481299212060789294, 0.1264236179284866091 ) ) ;
#35321=CARTESIAN_POINT ( 'NONE',  ( 0.07405724077823318263, -0.8937007873478103326, 0.1787899950787401604 ) ) ;
#35343=CARTESIAN_POINT ( 'NONE',  ( -0.2471922904502826257, 0.08811029028640915417, -0.05516800237527129391 ) ) ;
#35345=CARTESIAN_POINT ( 'NONE',  ( 0.07405724077823318263, -1.170399558780419680, -0.1787899950787401604 ) ) ;
#35347=CARTESIAN_POINT ( 'NONE',  ( -0.1787899950787401604, -0.1604330708123782034, -0.07405724077823318263 ) ) ;
#35355=CARTESIAN_POINT ( 'NONE',  ( -0.1797182628040039365, -0.1978784552523369933, 0.000000000000000000 ) ) ;
#35358=CARTESIAN_POINT ( 'NONE',  ( -0.07405724077823318263, -0.8001968503399367050, -0.1787899950787401604 ) ) ;
#35361=CARTESIAN_POINT ( 'NONE',  ( -0.1797182628040039087, -1.140299715094857502, 0.07444174185955065859 ) ) ;
#35366=DIRECTION ( 'NONE',  ( 0.000000000000000000, 1.000000000000000000, 0.000000000000000000 ) ) ;
#35380=CARTESIAN_POINT ( 'NONE',  ( 0.1113553986120547346, -1.016732283357039357, -0.1113553986120547346 ) ) ;
#35387=CARTESIAN_POINT ( 'NONE',  ( 3.284318927891251994E-17, -0.03001968498560657339, 0.1787899950787401882 ) ) ;
#35394=CARTESIAN_POINT ( 'NONE',  ( -0.07405724077823318263, -1.730314960576156968, 0.1787899950787401604 ) ) ;
#35405=CARTESIAN_POINT ( 'NONE',  ( -0.07405724077823318263, -0.6536672753158522253, -0.1787899950787401604 ) ) ;
#35408=CARTESIAN_POINT ( 'NONE',  ( -0.1639377702882210686, -0.08956143926285886625, 0.03448135181225767815 ) ) ;
#35410=VERTEX_POINT ( 'NONE', #26904 ) ;
#35413=CARTESIAN_POINT ( 'NONE',  ( 0.1113553986120547346, -0.01279527559055118092, 0.1113553986120547346 ) ) ;
#35419=CARTESIAN_POINT ( 'NONE',  ( 0.1797182628040039087, -0.6530949906854075504, 0.07444174185955046430 ) ) ;
#35422=CARTESIAN_POINT ( 'NONE',  ( -0.1574803149606297803, -0.5369094488188979053, 0.06523048226347956391 ) ) ;
#35423=CARTESIAN_POINT ( 'NONE',  ( -0.1509072091341974453, -0.09842519685039369248, 0.07426438480369451645 ) ) ;
#35429=CARTESIAN_POINT ( 'NONE',  ( 0.06523048226347956391, 0.07332677176107038619, 0.1574803149606297803 ) ) ;
#35443=CARTESIAN_POINT ( 'NONE',  ( 3.284318927891251994E-17, -1.801673228292693052, 0.1787899950787401882 ) ) ;
#35444=CARTESIAN_POINT ( 'NONE',  ( 0.07405724077823318263, -1.016732283410803905, 0.1787899950787401604 ) ) ;
#35445=CARTESIAN_POINT ( 'NONE',  ( -0.1574803149606300301, -1.407972440944881942, -0.06523048226347956391 ) ) ;
#35457=CARTESIAN_POINT ( 'NONE',  ( -0.1594274916601879644, 0.09247100924357856688, -0.1933875656399054732 ) ) ;
#35461=CARTESIAN_POINT ( 'NONE',  ( 0.1787899950787401882, -0.2722696375205775898, -2.189545951927503898E-17 ) ) ;
#35462=CARTESIAN_POINT ( 'NONE',  ( 0.1225656093788251993, -0.09842519685039370636, 0.1799294716465091037 ) ) ;
#35463=CARTESIAN_POINT ( 'NONE',  ( -0.1113553986120547346, 0.01673228346456692717, 0.1113553986120547346 ) ) ;
#35473=CARTESIAN_POINT ( 'NONE',  ( 0.07405724077823318263, -1.016732283410803905, 0.1787899950787401604 ) ) ;
#35474=CARTESIAN_POINT ( 'NONE',  ( 0.1787899950787401604, -1.238188976324190005, -0.07405724077823318263 ) ) ;
#35476=CARTESIAN_POINT ( 'NONE',  ( -0.1270800023317771588, -0.4390201875358015760, -0.1270800023317771588 ) ) ;
#35480=CARTESIAN_POINT ( 'NONE',  ( 0.1113553986120547346, 0.06594488188976378729, 0.1113553986120547346 ) ) ;
#35493=CARTESIAN_POINT ( 'NONE',  ( -0.1787899950787401604, -0.5590551180564723444, -0.07405724077823318263 ) ) ;
#35495=CARTESIAN_POINT ( 'NONE',  ( -0.1264236179284866091, -1.373523621993480326, 0.1264236179284866091 ) ) ;
#35497=CONICAL_SURFACE ( 'NONE', #14077, 0.2471922904502826812, 0.5235987755982992597 ) ;
#35500=ORIENTED_EDGE ( 'NONE', *, *, #6553, .T. ) ;
#35501=CARTESIAN_POINT ( 'NONE',  ( 0.000000000000000000, 0.0004086818895575684884, -0.2204724409448818867 ) ) ;
#35504=CARTESIAN_POINT ( 'NONE',  ( 0.08824861846397512311, -0.09842533983058743274, -0.1554957777122596418 ) ) ;
#35516=CARTESIAN_POINT ( 'NONE',  ( 0.06845965469993897656, -0.09851384754476909256, 0.2100007770323626122 ) ) ;
#35521=CARTESIAN_POINT ( 'NONE',  ( 0.07405724077823318263, -1.775714519410341419, 0.1787899950787401604 ) ) ;
#35523=CARTESIAN_POINT ( 'NONE',  ( 0.1787899950787401604, -0.6525590550643474153, 0.07405724077823318263 ) ) ;
#35526=ORIENTED_EDGE ( 'NONE', *, *, #1789, .F. ) ;
#35530=CARTESIAN_POINT ( 'NONE',  ( 0.1264236179284866091, -0.6943897637257637756, 0.1264236179284866091 ) ) ;
#35533=CARTESIAN_POINT ( 'NONE',  ( 0.1264236179284866091, 0.04761225224320220911, -0.1264236179284866091 ) ) ;
#35534=CARTESIAN_POINT ( 'NONE',  ( -0.07405724077823318263, -0.2687007873478113318, 0.1787899950787401604 ) ) ;
#35539=CARTESIAN_POINT ( 'NONE',  ( 2.892866454678787531E-17, -0.9625984251968503491, 0.1574803149606299191 ) ) ;
#35541=CARTESIAN_POINT ( 'NONE',  ( -0.07444174185955065859, -1.804669793835014469, 0.1797182628040039087 ) ) ;
#35542=CARTESIAN_POINT ( 'NONE',  ( -0.06523048226347956391, -0.4975393699712130080, -0.1574803149606300301 ) ) ;
#35543=CARTESIAN_POINT ( 'NONE',  ( 0.1264236179284866091, -0.3695866141194649179, -0.1264236179284866091 ) ) ;
#35551=CARTESIAN_POINT ( 'NONE',  ( 0.1264236179284866091, -0.1874999999462366451, 0.1264236179284866091 ) ) ;
#35553=CARTESIAN_POINT ( 'NONE',  ( 3.284318927891251994E-17, -0.8961614172690708369, 0.1787899950787401882 ) ) ;
#35576=CARTESIAN_POINT ( 'NONE',  ( -0.2471922904502826812, 0.08342621139836772781, -0.06611980121264428301 ) ) ;
#35578=CARTESIAN_POINT ( 'NONE',  ( -1.094772975963752103E-17, -1.167938928859159509, -0.1787899950787401882 ) ) ;
#35580=CARTESIAN_POINT ( 'NONE',  ( -0.07405724077823318263, -0.08661417317458304510, -0.1787899950787401604 ) ) ;
#35589=CONICAL_SURFACE ( 'NONE', #372, 0.2471922904502826812, 0.5235987755982992597 ) ;
#35591=CARTESIAN_POINT ( 'NONE',  ( -0.07405724077823318263, -0.7854330708123791194, 0.1787899950787401604 ) ) ;
#35593=CARTESIAN_POINT ( 'NONE',  ( -0.1797182628040039365, -1.300240659976745983, 0.000000000000000000 ) ) ;
#35603=CARTESIAN_POINT ( 'NONE',  ( -0.07405724077823318263, 0.03149606304588949135, -0.1787899950787401604 ) ) ;
#35617=CARTESIAN_POINT ( 'NONE',  ( 0.07405724077823318263, -0.06692913380450424277, 0.1787899950787401604 ) ) ;
#35623=CARTESIAN_POINT ( 'NONE',  ( 0.1674339218906837068, 0.08959396230940555594, 0.1887650509910807906 ) ) ;
#35627=CARTESIAN_POINT ( 'NONE',  ( 0.06523048226347956391, -0.4237204723334175305, -0.1574803149606300301 ) ) ;
#35628=CARTESIAN_POINT ( 'NONE',  ( -0.1787899950787401882, -1.737696850339937038, 0.000000000000000000 ) ) ;
#35631=VECTOR ( 'NONE', #13078, 39.37007874015748143 ) ;
#35653=CARTESIAN_POINT ( 'NONE',  ( 0.1797182628040039365, -0.8868548332050926186, -2.200913952912460540E-17 ) ) ;
#35656=CARTESIAN_POINT ( 'NONE',  ( 0.1574803149606300301, -0.5221456692913385433, 0.06523048226347956391 ) ) ;
#35677=CARTESIAN_POINT ( 'NONE',  ( 0.1797182628040039087, 0.05556642663742687727, 0.07444174185955046430 ) ) ;
#35678=CARTESIAN_POINT ( 'NONE',  ( 3.284318927891251994E-17, -1.019192913332062966, 0.1787899950787401882 ) ) ;
#35679=CARTESIAN_POINT ( 'NONE',  ( 0.1574803149606300301, -1.501476377952755570, -0.06523048226347956391 ) ) ;
#35693=CARTESIAN_POINT ( 'NONE',  ( 3.284318927891251994E-17, -0.3214822359457744638, 0.1787899950787401882 ) ) ;
#35701=CARTESIAN_POINT ( 'NONE',  ( -1.094772975963752103E-17, -1.156988188922614125, -0.1787899950787401882 ) ) ;
#35702=CARTESIAN_POINT ( 'NONE',  ( 0.1264236179284866091, -1.363681102308440973, 0.1264236179284866091 ) ) ;
#35704=CARTESIAN_POINT ( 'NONE',  ( -0.07444174185955065859, -0.5054571954098173725, 0.1797182628040039087 ) ) ;
#35708=CARTESIAN_POINT ( 'NONE',  ( 0.1574803149606300301, -0.08907480314960623813, 0.06523048226347956391 ) ) ;
#35724=CARTESIAN_POINT ( 'NONE',  ( -0.07405724077823318263, -0.6427165353793066194, -0.1787899950787401604 ) ) ;
#35725=CARTESIAN_POINT ( 'NONE',  ( 0.1574803149606300301, -1.107775590551181688, -0.06523048226347956391 ) ) ;
#35741=CARTESIAN_POINT ( 'NONE',  ( -9.642888182262618425E-18, -0.1850393699712129802, -0.1574803149606299191 ) ) ;
#35747=CARTESIAN_POINT ( 'NONE',  ( -0.09636693384614980484, -0.09851383887303406806, -0.1572292210079062891 ) ) ;
#35748=B_SPLINE_CURVE_WITH_KNOTS ( 'NONE', 3,
 ( #19883, #34994, #31640, #13632, #24427, #27355, #5504, #1665, #45743, #42139, #16312, #20117, #45981, #6196, #41898, #2364, #12952, #17234, #8867 ),
 .UNSPECIFIED., .F., .F.,
 ( 4, 1, 1, 1, 2, 2, 1, 1, 1, 1, 2, 2, 4 ),
 ( 0.000000000000000000, 0.1249999999999964473, 0.1874999999999945599, 0.2187499999999934497, 0.2343749999999929223, 0.2499999999999923950, 0.3749999999999917843, 0.4374999999999915068, 0.4687499999999910627, 0.4843749999999910627, 0.4921874999999908407, 0.4999999999999905631, 1.000000000000000000 ),
 .UNSPECIFIED. ) ;
#35755=CARTESIAN_POINT ( 'NONE',  ( 0.1787899950787401882, -0.8075787401037164415, -2.189545951927503898E-17 ) ) ;
#35757=LINE ( 'NONE', #2897, #43126 ) ;
#35759=CARTESIAN_POINT ( 'NONE',  ( -0.1787899950787401604, -0.05327357452845130764, 0.07405724077823318263 ) ) ;
#35760=CARTESIAN_POINT ( 'NONE',  ( -0.1264236179284866091, -0.2416338582139531399, -0.1264236179284866091 ) ) ;
#35761=CARTESIAN_POINT ( 'NONE',  ( -0.07405724077823318263, 0.001968503990771400605, 0.1787899950787401604 ) ) ;
#35766=EDGE_CURVE ( 'NONE', #763, #34774, #3960, .T. ) ;
#35768=CARTESIAN_POINT ( 'NONE',  ( -0.06523048226347956391, -0.9650590551181117416, 0.1574803149606297803 ) ) ;
#35769=CARTESIAN_POINT ( 'NONE',  ( -0.1797182628040039087, -1.657031998559424846, -0.07444174185955065859 ) ) ;
#35776=EDGE_CURVE ( 'NONE', #27412, #30178, #12509, .T. ) ;
#35778=CARTESIAN_POINT ( 'NONE',  ( 3.284318927891251994E-17, -0.1530511810485986057, 0.1787899950787401882 ) ) ;
#35780=CARTESIAN_POINT ( 'NONE',  ( 0.1264236179284866091, -0.8813976377415118080, -0.1264236179284866091 ) ) ;
#35797=CARTESIAN_POINT ( 'NONE',  ( 0.1787899950787401604, -0.06692913380450424277, 0.07405724077823318263 ) ) ;
#35806=CARTESIAN_POINT ( 'NONE',  ( -0.1264236179284866091, -1.310655464292230565, 0.1264236179284866091 ) ) ;
#35808=CARTESIAN_POINT ( 'NONE',  ( -0.1787899950787401604, -0.1555118109698585271, 0.07405724077823318263 ) ) ;
#35813=CARTESIAN_POINT ( 'NONE',  ( 0.1787899950787401604, -1.479330708607653699, -0.07405724077823318263 ) ) ;
#35814=CARTESIAN_POINT ( 'NONE',  ( 0.1264236179284866091, -0.7682086613635590311, -0.1264236179284866091 ) ) ;
#35818=CARTESIAN_POINT ( 'NONE',  ( -0.1270800023317771588, -1.295319400134226306, 0.1270800023317771588 ) ) ;
#35825=CARTESIAN_POINT ( 'NONE',  ( -0.07154104892864131260, 0.1299212598425195930, 0.1541805736627041012 ) ) ;
#35831=CARTESIAN_POINT ( 'NONE',  ( 0.1264236179284866091, 0.01427165359707059308, 0.1264236179284866091 ) ) ;
#35843=CARTESIAN_POINT ( 'NONE',  ( 0.1787899950787401604, -0.02263779522182702078, 0.07405724077823318263 ) ) ;
#35850=CARTESIAN_POINT ( 'NONE',  ( -0.07405724077823318263, -1.651574803095843258, 0.1787899950787401604 ) ) ;
#35859=CARTESIAN_POINT ( 'NONE',  ( -0.1264236179284866091, -0.8480570390953799942, -0.1264236179284866091 ) ) ;
#35861=CARTESIAN_POINT ( 'NONE',  ( -0.06485735496959410540, -0.08956202182541239676, 0.1433340101501935082 ) ) ;
#35875=CARTESIAN_POINT ( 'NONE',  ( 0.1797182628040039087, -0.9237642820239904129, -0.07444174185955065859 ) ) ;
#35876=CARTESIAN_POINT ( 'NONE',  ( 0.2471922904502826535, 0.09123121687245852596, 0.04590630800384764426 ) ) ;
#35879=CARTESIAN_POINT ( 'NONE',  ( -0.06523048226347956391, -0.6107283464566929387, 0.1574803149606297803 ) ) ;
#35880=CARTESIAN_POINT ( 'NONE',  ( -0.1485133662041858704, 0.1246681010365934816, -0.06542554175153637852 ) ) ;
#35894=VERTEX_POINT ( 'NONE', #25274 ) ;
#35897=CARTESIAN_POINT ( 'NONE',  ( -0.1797182628040039087, 0.1195428045901827108, 0.07444174185955065859 ) ) ;
#35898=CARTESIAN_POINT ( 'NONE',  ( -0.1787899950787401604, -1.110236220418677533, -0.07405724077823318263 ) ) ;
#35899=CARTESIAN_POINT ( 'NONE',  ( -0.06523048226347956391, -1.476870078740157188, 0.1574803149606297803 ) ) ;
#35904=CARTESIAN_POINT ( 'NONE',  ( 2.892866454678787531E-17, 0.07086614183981043702, 0.1574803149606299191 ) ) ;
#35910=CARTESIAN_POINT ( 'NONE',  ( -0.2471922904502826535, 0.09660984127287175482, 0.02629157619858309841 ) ) ;
#35912=CARTESIAN_POINT ( 'NONE',  ( 0.08640460078259740162, -0.09201407021830487754, -0.2355472506762735785 ) ) ;
#35914=CARTESIAN_POINT ( 'NONE',  ( -0.1264236179284866091, -0.2476633383079787365, 0.1264236179284866091 ) ) ;
#35924=CARTESIAN_POINT ( 'NONE',  ( -0.1787899950787401604, -1.149606299158835387, -0.07405724077823318263 ) ) ;
#35925=CARTESIAN_POINT ( 'NONE',  ( -0.1787899950787401604, -1.375984251914741163, 0.07405724077823318263 ) ) ;
#35934=CARTESIAN_POINT ( 'NONE',  ( -0.06523048226347956391, -0.1776574803149607584, 0.1574803149606297803 ) ) ;
#35938=EDGE_CURVE ( 'NONE', #43256, #13671, #9394, .T. ) ;
#35946=VERTEX_POINT ( 'NONE', #9547 ) ;
#35948=CARTESIAN_POINT ( 'NONE',  ( -0.06523048226347956391, 0.09301181113114896648, -0.1574803149606300301 ) ) ;
#35949=B_SPLINE_CURVE_WITH_KNOTS ( 'NONE', 3,
 ( #2022, #19521, #5372, #12603, #34631, #20227, #23373, #41776, #8497, #37500, #1781, #30358, #1061, #9218, #27706, #37981, #34171, #12360, #22886, #5133, #33939 ),
 .UNSPECIFIED., .F., .F.,
 ( 4, 2, 1, 1, 2, 2, 2, 1, 1, 1, 2, 2, 4 ),
 ( 0.000000000000000000, 0.1249999999999948097, 0.1874999999999923672, 0.2187499999999910072, 0.2343749999999906186, 0.2499999999999902855, 0.3749999999999891753, 0.4374999999999888423, 0.4687499999999888423, 0.4843749999999888978, 0.4921874999999891753, 0.4999999999999894529, 1.000000000000000000 ),
 .UNSPECIFIED. ) ;
#35951=CARTESIAN_POINT ( 'NONE',  ( 0.1574803149606300301, -1.609744094380661572, -0.06523048226347956391 ) ) ;
#35952=CARTESIAN_POINT ( 'NONE',  ( 0.1264236179284866091, -0.6205708660879685201, 0.1264236179284866091 ) ) ;
#35953=CARTESIAN_POINT ( 'NONE',  ( -0.1574803149606297803, -1.048720472440944684, 0.06523048226347956391 ) ) ;
#35958=ORIENTED_EDGE ( 'NONE', *, *, #28013, .T. ) ;
#35968=CARTESIAN_POINT ( 'NONE',  ( 0.1588219152425836833, -0.09266989036297294813, 0.1937372027061967927 ) ) ;
#35970=CARTESIAN_POINT ( 'NONE',  ( 0.1574803149606300301, -0.2711614172153075097, -0.06523048226347956391 ) ) ;
#35978=CARTESIAN_POINT ( 'NONE',  ( 0.07405724077823318263, -1.696974361930027708, 0.1787899950787401604 ) ) ;
#35985=CARTESIAN_POINT ( 'NONE',  ( 0.07405724077823318263, -0.8543307086076546986, 0.1787899950787401604 ) ) ;
#35990=CARTESIAN_POINT ( 'NONE',  ( 0.1787899950787401604, -0.1566200312213647527, 0.07405724077823318263 ) ) ;
#35991=CARTESIAN_POINT ( 'NONE',  ( 3.284318927891251994E-17, -0.3056102361667090705, 0.1787899950787401882 ) ) ;
#35993=CARTESIAN_POINT ( 'NONE',  ( 3.284318927891251994E-17, 0.04379921265218874454, 0.1787899950787401882 ) ) ;
#36001=CARTESIAN_POINT ( 'NONE',  ( 0.1270800023317771588, -1.669335148165722371, -0.1270800023317771588 ) ) ;
#36002=CARTESIAN_POINT ( 'NONE',  ( -0.1264236179284866091, -0.4384842519147402196, -0.1264236179284866091 ) ) ;
#36008=CARTESIAN_POINT ( 'NONE',  ( -0.1113553986120547346, -0.9183070865066457200, 0.1113553986120547346 ) ) ;
#36009=CARTESIAN_POINT ( 'NONE',  ( -0.1787899950787401604, -0.08169291333206318839, 0.07405724077823318263 ) ) ;
#36011=CARTESIAN_POINT ( 'NONE',  ( 0.1787899950787401882, -1.083169291284818980, -2.189545951927503898E-17 ) ) ;
#36031=CARTESIAN_POINT ( 'NONE',  ( 3.284318927891251994E-17, -0.03494094482812622193, 0.1787899950787401882 ) ) ;
#36041=CARTESIAN_POINT ( 'NONE',  ( 3.284318927891251994E-17, -1.266364125709553257, 0.1787899950787401882 ) ) ;
#36043=CARTESIAN_POINT ( 'NONE',  ( -1.094772975963752103E-17, -0.2071850393163153503, -0.1787899950787401882 ) ) ;
#36050=CARTESIAN_POINT ( 'NONE',  ( 0.1787899950787401604, -1.641732283410802573, 0.07405724077823318263 ) ) ;
#36051=CARTESIAN_POINT ( 'NONE',  ( 0.1787899950787401604, -0.7312992125446612368, -0.07405724077823318263 ) ) ;
#36057=VECTOR ( 'NONE', #38279, 39.37007874015748143 ) ;
#36079=DIRECTION ( 'NONE',  ( 0.000000000000000000, 0.000000000000000000, 1.000000000000000000 ) ) ;
#36080=CARTESIAN_POINT ( 'NONE',  ( 0.1787899950787401882, -0.02017716530056720692, -2.189545951927503898E-17 ) ) ;
#36082=( BOUNDED_CURVE ( )  B_SPLINE_CURVE ( 2, ( #14057, #18122, #3260, #24841, #43753, #25325, #32042, #3511, #32768 ),
 .UNSPECIFIED., .F., .F. ) 
 B_SPLINE_CURVE_WITH_KNOTS ( ( 3, 2, 2, 2, 3 ),
 ( 0.07499999999999999722, 0.07749999999999999944, 0.08000000000000000167, 0.08250000000000000389, 0.08500000000000000611 ),
 .UNSPECIFIED. ) 
 CURVE ( )  GEOMETRIC_REPRESENTATION_ITEM ( )  RATIONAL_B_SPLINE_CURVE ( ( 1.000000000000000000, 0.9238795325112869605, 1.000000000000000000, 0.9238795325112869605, 1.000000000000000000, 0.9238795325112869605, 1.000000000000000000, 0.9238795325112869605, 1.000000000000000000 ) ) 
 REPRESENTATION_ITEM ( '' )  ) ;
#36084=CARTESIAN_POINT ( 'NONE',  ( 0.1293255151920606749, -0.09842519685039366473, -0.2107669498569183786 ) ) ;
#36091=CARTESIAN_POINT ( 'NONE',  ( 0.1574803149606300301, 0.07824803160359000698, 0.06523048226347956391 ) ) ;
#36099=CARTESIAN_POINT ( 'NONE',  ( -0.1787899950787401604, -0.8800452280717578901, 0.07405724077823318263 ) ) ;
#36119=CARTESIAN_POINT ( 'NONE',  ( -0.1797182628040039365, -0.8277997150948562810, 0.000000000000000000 ) ) ;
#36120=CARTESIAN_POINT ( 'NONE',  ( 0.2471922904502826257, 0.09842519685039370636, 0.006585516632626051831 ) ) ;
#36123=CARTESIAN_POINT ( 'NONE',  ( -0.1113553986120547346, -0.6525590551181101873, 0.1113553986120547346 ) ) ;
#36145=CARTESIAN_POINT ( 'NONE',  ( 0.07444174185955046430, 0.02603886758230882295, -0.1797182628040039087 ) ) ;
#36146=CARTESIAN_POINT ( 'NONE',  ( 0.1264236179284866091, -1.161909448765133801, -0.1264236179284866091 ) ) ;
#36147=CARTESIAN_POINT ( 'NONE',  ( 0.06523048226347956391, -1.550688976377951889, 0.1574803149606297803 ) ) ;
#36155=CARTESIAN_POINT ( 'NONE',  ( 0.06523048226347956391, -1.407972440837354622, -0.1574803149606300301 ) ) ;
#36167=CARTESIAN_POINT ( 'NONE',  ( 0.07405724077823318263, -0.3977617635048297240, 0.1787899950787401604 ) ) ;
#36168=CARTESIAN_POINT ( 'NONE',  ( -0.07591074332868011365, -0.09842519685039370636, 0.1427273573094925141 ) ) ;
#36178=ORIENTED_EDGE ( 'NONE', *, *, #476, .F. ) ;
#36180=CARTESIAN_POINT ( 'NONE',  ( -0.1264236179284866091, -1.220964566875370139, 0.1264236179284866091 ) ) ;
#36181=CARTESIAN_POINT ( 'NONE',  ( -0.07405724077823318263, -1.410433070812377565, 0.1787899950787401604 ) ) ;
#36187=AXIS2_PLACEMENT_3D ( 'NONE', #11552, #41623, #9071 ) ;
#36194=FACE_OUTER_BOUND ( 'NONE', #38021, .T. ) ;
#36199=CARTESIAN_POINT ( 'NONE',  ( -0.1787899950787401604, -0.04232283459190579189, -0.07405724077823318263 ) ) ;
#36201=CARTESIAN_POINT ( 'NONE',  ( 2.892866454678787531E-17, 0.1102362205799679168, 0.1574803149606299191 ) ) ;
#36203=CARTESIAN_POINT ( 'NONE',  ( 0.1574803149606300301, -1.531003936900347639, -0.06523048226347956391 ) ) ;
#36204=CARTESIAN_POINT ( 'NONE',  ( -0.1787899950787401882, -0.6747047243556849594, 0.000000000000000000 ) ) ;
#36206=CARTESIAN_POINT ( 'NONE',  ( -0.1574803149606297803, -1.088090551181102539, 0.06523048226347956391 ) ) ;
#36213=VERTEX_POINT ( 'NONE', #5333 ) ;
#36227=CARTESIAN_POINT ( 'NONE',  ( 0.1574803149606299191, -0.1948818896562523328, -1.928577636452523993E-17 ) ) ;
#36236=CARTESIAN_POINT ( 'NONE',  ( 0.1264236179284866091, -1.763411369804041451, -0.1264236179284866091 ) ) ;
#36240=CARTESIAN_POINT ( 'NONE',  ( 0.1787899950787401604, -0.4212598424659216856, 0.07405724077823318263 ) ) ;
#36241=CARTESIAN_POINT ( 'NONE',  ( 0.1264236179284866091, -0.9207677164816693294, -0.1264236179284866091 ) ) ;
#36242=CARTESIAN_POINT ( 'NONE',  ( -0.2471902452994138577, -0.09796597228571106430, -0.01325394226265560506 ) ) ;
#36244=CARTESIAN_POINT ( 'NONE',  ( -0.1797182628040039087, -0.2347879040712344823, 0.07444174185955065859 ) ) ;
#36246=CARTESIAN_POINT ( 'NONE',  ( -1.094772975963752103E-17, -0.1443168816150655620, -0.1787899950787401882 ) ) ;
#36247=CARTESIAN_POINT ( 'NONE',  ( -0.1787899950787401604, -0.2785433070328505734, -0.07405724077823318263 ) ) ;
#36248=CARTESIAN_POINT ( 'NONE',  ( -0.07405724077823318263, -0.07677165348954355373, 0.1787899950787401604 ) ) ;
#36249=DIRECTION ( 'NONE',  ( 0.000000000000000000, 1.000000000000000000, 0.000000000000000000 ) ) ;
#36254=CARTESIAN_POINT ( 'NONE',  ( -0.1270800023317771588, -1.767760345016116119, 0.1270800023317771588 ) ) ;
#36263=CARTESIAN_POINT ( 'NONE',  ( -0.1113553986120547346, -0.9281496061916850726, -0.1113553986120547346 ) ) ;
#36264=CARTESIAN_POINT ( 'NONE',  ( -0.1264236179284866091, -0.04970472435568527164, -0.1264236179284866091 ) ) ;
#36267=CARTESIAN_POINT ( 'NONE',  ( -0.1787899950787401882, -1.063484251914740275, 0.000000000000000000 ) ) ;
#36271=VERTEX_POINT ( 'NONE', #16388 ) ;
#36287=CARTESIAN_POINT ( 'NONE',  ( -0.07405724077823318263, -0.01279527553678766298, -0.1787899950787401604 ) ) ;
#36295=CARTESIAN_POINT ( 'NONE',  ( 0.1264236179284866091, -1.330340503662309271, -0.1264236179284866091 ) ) ;
#36298=CARTESIAN_POINT ( 'NONE',  ( 0.1264236179284866091, -0.3400590550643468601, 0.1264236179284866091 ) ) ;
#36303=CARTESIAN_POINT ( 'NONE',  ( -0.2471922891335203709, -0.07779967023288102135, 0.07764737426212238447 ) ) ;
#36305=CARTESIAN_POINT ( 'NONE',  ( 0.1787899950787401882, -1.639271653489543290, -2.189545951927503898E-17 ) ) ;
#36306=CARTESIAN_POINT ( 'NONE',  ( -0.1264236179284866091, -0.7977362204186770889, -0.1264236179284866091 ) ) ;
#36309=CARTESIAN_POINT ( 'NONE',  ( 0.1797182628040039087, -1.317465069425564295, -0.07444174185955065859 ) ) ;
#36337=CARTESIAN_POINT ( 'NONE',  ( -0.1787899950787401882, -0.0004921259304884630223, 0.000000000000000000 ) ) ;
#36346=CARTESIAN_POINT ( 'NONE',  ( 0.1574803149606299191, 0.08070866152484981737, -1.928577636452523993E-17 ) ) ;
#36349=ORIENTED_EDGE ( 'NONE', *, *, #9712, .F. ) ;
#36356=CARTESIAN_POINT ( 'NONE',  ( -1.094772975963752103E-17, -0.8529782989378996705, -0.1787899950787401882 ) ) ;
#36357=CARTESIAN_POINT ( 'NONE',  ( 0.01517891734636545205, -0.08956197014793249034, 0.1509071277318320969 ) ) ;
#36358=CARTESIAN_POINT ( 'NONE',  ( -0.1264236179284866091, 0.1126968504474643862, -0.1264236179284866091 ) ) ;
#36364=DIRECTION ( 'NONE',  ( 0.000000000000000000, -1.000000000000000000, 0.000000000000000000 ) ) ;
#36369=CARTESIAN_POINT ( 'NONE',  ( -0.1270800023317771588, -0.7835083765121790833, 0.1270800023317771588 ) ) ;
#36373=CARTESIAN_POINT ( 'NONE',  ( -0.06523048226347956391, -0.5861220472440943352, -0.1574803149606300301 ) ) ;
#36374=CARTESIAN_POINT ( 'NONE',  ( -0.01694847244370521061, 0.1204840602458819576, -0.1578856350490314697 ) ) ;
#36381=( BOUNDED_CURVE ( )  B_SPLINE_CURVE ( 2, ( #9827, #38811, #35463, #27832, #31645, #9590, #24211, #38578, #21054 ),
 .UNSPECIFIED., .F., .T. ) 
 B_SPLINE_CURVE_WITH_KNOTS ( ( 3, 2, 2, 2, 3 ),
 ( 0.07499999999999999722, 0.07749999999999999944, 0.08000000000000000167, 0.08250000000000000389, 0.08500000000000000611 ),
 .UNSPECIFIED. ) 
 CURVE ( )  GEOMETRIC_REPRESENTATION_ITEM ( )  RATIONAL_B_SPLINE_CURVE ( ( 1.000000000000000000, 0.9238795325112869605, 1.000000000000000000, 0.9238795325112869605, 1.000000000000000000, 0.9238795325112869605, 1.000000000000000000, 0.9238795325112869605, 1.000000000000000000 ) ) 
 REPRESENTATION_ITEM ( '' )  ) ;
#36395=CARTESIAN_POINT ( 'NONE',  ( 3.284318927891251994E-17, -1.255413385773007873, 0.1787899950787401882 ) ) ;
#36396=CARTESIAN_POINT ( 'NONE',  ( 0.06523048226347956391, -1.471948818897638178, 0.1574803149606297803 ) ) ;
#36403=CARTESIAN_POINT ( 'NONE',  ( -0.2471922904502826535, 0.06774690380565037695, 0.09545378441109995948 ) ) ;
#36407=CARTESIAN_POINT ( 'NONE',  ( -0.1787899950787401882, -0.4494349918512858255, 0.000000000000000000 ) ) ;
#36408=CARTESIAN_POINT ( 'NONE',  ( 0.05546883683243283847, -0.09842519685039370636, 0.1418485093170885891 ) ) ;
#36416=CARTESIAN_POINT ( 'NONE',  ( -0.1787899950787401882, -1.107775590497417362, 0.000000000000000000 ) ) ;
#36417=CARTESIAN_POINT ( 'NONE',  ( -0.1264236179284866091, -1.373523621993480326, 0.1264236179284866091 ) ) ;
#36420=CARTESIAN_POINT ( 'NONE',  ( 0.1270800023317771588, -0.5768154631263527898, 0.1270800023317771588 ) ) ;
#36424=CARTESIAN_POINT ( 'NONE',  ( 0.1113553986120547346, -0.1210629921259842590, -0.1113553986120547346 ) ) ;
#36436=CARTESIAN_POINT ( 'NONE',  ( 0.07405724077823318263, -0.02755905506434671789, 0.1787899950787401604 ) ) ;
#36438=ORIENTED_EDGE ( 'NONE', *, *, #45043, .T. ) ;
#36440=CARTESIAN_POINT ( 'NONE',  ( 0.1264236179284866091, -1.629429133804503937, -0.1264236179284866091 ) ) ;
#36441=CARTESIAN_POINT ( 'NONE',  ( 2.892866454678787531E-17, -1.582677165246803019, 0.1574803149606299191 ) ) ;
#36442=CARTESIAN_POINT ( 'NONE',  ( -0.1787899950787401604, -0.7116141731745821986, 0.07405724077823318263 ) ) ;
#36444=CARTESIAN_POINT ( 'NONE',  ( -0.1113553986120547346, -1.006889763779527547, 0.1113553986120547346 ) ) ;
#36462=CARTESIAN_POINT ( 'NONE',  ( 0.09178263254600295407, -0.09851384182930648936, -0.1728663888072523580 ) ) ;
#36464=VERTEX_POINT ( 'NONE', #3404 ) ;
#36466=CARTESIAN_POINT ( 'NONE',  ( -0.1787899950787401604, -1.667446802874908096, 0.07405724077823318263 ) ) ;
#36471=CARTESIAN_POINT ( 'NONE',  ( 3.284318927891251994E-17, -0.8567913385289133155, 0.1787899950787401882 ) ) ;
#36477=CARTESIAN_POINT ( 'NONE',  ( 0.1270800023317771588, -0.1339020772995811182, -0.1270800023317771588 ) ) ;
#36478=CARTESIAN_POINT ( 'NONE',  ( -0.1264236179284866091, -0.06065546429223091229, -0.1264236179284866091 ) ) ;
#36479=CARTESIAN_POINT ( 'NONE',  ( 0.1264236179284866091, -0.3006889763241893943, 0.1264236179284866091 ) ) ;
#36480=CARTESIAN_POINT ( 'NONE',  ( 0.1264236179284866091, -0.09891732278088229136, -0.1264236179284866091 ) ) ;
#36481=DIRECTION ( 'NONE',  ( 0.000000000000000000, 0.000000000000000000, 1.000000000000000000 ) ) ;
#36493=CARTESIAN_POINT ( 'NONE',  ( 0.1787899950787401604, -0.2588582676627719792, -0.07405724077823318263 ) ) ;
#36495=CARTESIAN_POINT ( 'NONE',  ( 0.07405724077823318263, -1.051181102308440529, 0.1787899950787401604 ) ) ;
#36500=ORIENTED_EDGE ( 'NONE', *, *, #4790, .F. ) ;
#36515=CARTESIAN_POINT ( 'NONE',  ( 0.1264236179284866091, 0.009350393754550925460, 0.1264236179284866091 ) ) ;
#36522=CARTESIAN_POINT ( 'NONE',  ( 0.1264236179284866091, -1.222072787126875948, 0.1264236179284866091 ) ) ;
#36524=CARTESIAN_POINT ( 'NONE',  ( 0.1787899950787401604, -0.2145669290800947537, -0.07405724077823318263 ) ) ;
#36533=CARTESIAN_POINT ( 'NONE',  ( 0.1264236179284866091, -1.683562992072220599, 0.1264236179284866091 ) ) ;
#36534=CARTESIAN_POINT ( 'NONE',  ( -1.094772975963752103E-17, -1.624507873961984261, -0.1787899950787401882 ) ) ;
#36537=CARTESIAN_POINT ( 'NONE',  ( 3.301370929368692659E-17, -1.251028061551548998, 0.1797182628040039365 ) ) ;
#36556=CARTESIAN_POINT ( 'NONE',  ( 0.06523048226347956391, -1.029035432963338215, 0.1574803149606297803 ) ) ;
#36562=CARTESIAN_POINT ( 'NONE',  ( -0.1264236179284866091, -0.2022637794737956740, -0.1264236179284866091 ) ) ;
#36567=CARTESIAN_POINT ( 'NONE',  ( -0.1006623723854965097, 0.09658349877441903264, 0.2273156230721088411 ) ) ;
#36571=CARTESIAN_POINT ( 'NONE',  ( -0.1113553986120547346, 0.05610236231225141507, -0.1113553986120547346 ) ) ;
#36577=CARTESIAN_POINT ( 'NONE',  ( -0.1264236179284866091, -0.7594743619300257098, 0.1264236179284866091 ) ) ;
#36588=MANIFOLD_SOLID_BREP ( 'Threaded Bushing', #18609 ) ;
#36594=CARTESIAN_POINT ( 'NONE',  ( 3.301370929368692659E-17, -0.7785871166696594070, 0.1797182628040039365 ) ) ;
#36603=VERTEX_POINT ( 'NONE', #37649 ) ;
#36606=CARTESIAN_POINT ( 'NONE',  ( 0.07405724077823318263, -0.6968503936470246130, 0.1787899950787401604 ) ) ;
#36613=CARTESIAN_POINT ( 'NONE',  ( 0.1113553986120547346, -1.538385826771653475, -0.1113553986120547346 ) ) ;
#36616=VERTEX_POINT ( 'NONE', #36943 ) ;
#36619=ORIENTED_EDGE ( 'NONE', *, *, #39590, .F. ) ;
#36629=CARTESIAN_POINT ( 'NONE',  ( 0.1787899950787401604, -0.3928405036623095481, 0.07405724077823318263 ) ) ;
#36630=CARTESIAN_POINT ( 'NONE',  ( 0.01579235578554630259, -0.09842519685039370636, 0.1544717903359340561 ) ) ;
#36631=ADVANCED_FACE ( 'NONE', ( #40979 ), #22794, .T. ) ;
#36640=CARTESIAN_POINT ( 'NONE',  ( 0.1787899950787401882, -1.166830708607653477, -2.189545951927503898E-17 ) ) ;
#36641=CARTESIAN_POINT ( 'NONE',  ( -0.07405724077823318263, -1.307086614119465695, -0.1787899950787401604 ) ) ;
#36648=CARTESIAN_POINT ( 'NONE',  ( -0.1574803149606299191, -0.1062992125984252023, 0.000000000000000000 ) ) ;
#36653=AXIS2_PLACEMENT_3D ( 'NONE', #17644, #25073, #13358 ) ;
#36659=CARTESIAN_POINT ( 'NONE',  ( -0.07405724077823318263, -0.04724409443442544737, -0.1787899950787401604 ) ) ;
#36663=CARTESIAN_POINT ( 'NONE',  ( -0.1264236179284866091, -1.540846456639149542, -0.1264236179284866091 ) ) ;
#36664=CARTESIAN_POINT ( 'NONE',  ( -0.06523048226347956391, -1.585137795168063413, 0.1574803149606297803 ) ) ;
#36665=CARTESIAN_POINT ( 'NONE',  ( 0.07405724077823318263, -0.7017716534895438452, 0.1787899950787401604 ) ) ;
#36667=CARTESIAN_POINT ( 'NONE',  ( 0.1574803149606300301, -1.073326771653543066, 0.06523048226347956391 ) ) ;
#36694=AXIS2_PLACEMENT_3D ( 'NONE', #13672, #38839, #46019 ) ;
#36699=CARTESIAN_POINT ( 'NONE',  ( 0.07405724077823318263, -0.4261811023084413064, 0.1787899950787401604 ) ) ;
#36700=CARTESIAN_POINT ( 'NONE',  ( -0.1787899950787401882, -0.9453740156942677109, 0.000000000000000000 ) ) ;
#36703=CARTESIAN_POINT ( 'NONE',  ( 0.1797182628040039365, -0.2569335733625732199, -2.200913952912460540E-17 ) ) ;
#36704=CARTESIAN_POINT ( 'NONE',  ( -0.1264236179284866091, -0.1787657005127031573, -0.1264236179284866091 ) ) ;
#36705=CARTESIAN_POINT ( 'NONE',  ( 0.2471889898699782262, -0.06575181108683454678, -0.09853485309448883900 ) ) ;
#36716=CARTESIAN_POINT ( 'NONE',  ( -1.094772975963752103E-17, -0.2908464566391499861, -0.1787899950787401882 ) ) ;
#36720=CARTESIAN_POINT ( 'NONE',  ( 0.07405724077823318263, -1.090551181048598606, 0.1787899950787401604 ) ) ;
#36729=CARTESIAN_POINT ( 'NONE',  ( -0.1113553986120547346, -1.203740157372787500, -0.1113553986120547346 ) ) ;
#36738=CARTESIAN_POINT ( 'NONE',  ( -0.1264236179284866091, 0.02903543312462964626, -0.1264236179284866091 ) ) ;
#36747=AXIS2_PLACEMENT_3D ( 'NONE', #2295, #27033, #20275 ) ;
#36749=CARTESIAN_POINT ( 'NONE',  ( -0.1787899950787401882, -1.354946802874907652, 0.000000000000000000 ) ) ;
#36751=CARTESIAN_POINT ( 'NONE',  ( 3.284318927891251994E-17, -0.2662401574265516047, 0.1787899950787401882 ) ) ;
#36761=CARTESIAN_POINT ( 'NONE',  ( -0.1787899950787401604, -1.622047244040725866, -0.07405724077823318263 ) ) ;
#36762=CARTESIAN_POINT ( 'NONE',  ( 0.1264236179284866091, -1.747539370024976391, -0.1264236179284866091 ) ) ;
#36765=CARTESIAN_POINT ( 'NONE',  ( -0.1797182628040039365, -1.339610738716903393, 0.000000000000000000 ) ) ;
#36770=CARTESIAN_POINT ( 'NONE',  ( -0.03645729789547116212, 0.1299212598425194265, 0.1690525858836274820 ) ) ;
#36774=DIRECTION ( 'NONE',  ( 0.000000000000000000, 0.000000000000000000, 1.000000000000000000 ) ) ;
#36775=( BOUNDED_CURVE ( )  B_SPLINE_CURVE ( 2, ( #2103, #45947, #38064, #13159, #9550, #38773, #5933, #35191, #18144 ),
 .UNSPECIFIED., .F., .F. ) 
 B_SPLINE_CURVE_WITH_KNOTS ( ( 3, 2, 2, 2, 3 ),
 ( 0.06500000000000000222, 0.06750000000000000444, 0.07000000000000000666, 0.07249999999999999500, 0.07499999999999999722 ),
 .UNSPECIFIED. ) 
 CURVE ( )  GEOMETRIC_REPRESENTATION_ITEM ( )  RATIONAL_B_SPLINE_CURVE ( ( 1.000000000000000000, 0.9238795325112869605, 1.000000000000000000, 0.9238795325112869605, 1.000000000000000000, 0.9238795325112869605, 1.000000000000000000, 0.9238795325112869605, 1.000000000000000000 ) ) 
 REPRESENTATION_ITEM ( '' )  ) ;
#36793=CARTESIAN_POINT ( 'NONE',  ( 2.892866454678787531E-17, 0.06102362204724409711, 0.1574803149606299191 ) ) ;
#36795=CARTESIAN_POINT ( 'NONE',  ( -0.1787899950787401604, -0.1604330708123782034, -0.07405724077823318263 ) ) ;
#36799=CARTESIAN_POINT ( 'NONE',  ( -0.04858533447342696515, -0.07294156354243679086, 0.2573812140284292838 ) ) ;
#36802=EDGE_CURVE ( 'NONE', #35946, #7112, #28790, .T. ) ;
#36804=CARTESIAN_POINT ( 'NONE',  ( -9.642888182262618425E-18, 0.05118110246973173183, -0.1574803149606299191 ) ) ;
#36812=CARTESIAN_POINT ( 'NONE',  ( 0.1787899950787401882, -0.8628208186229389121, -2.189545951927503898E-17 ) ) ;
#36814=CARTESIAN_POINT ( 'NONE',  ( 0.07405724077823318263, 0.1299212598962831977, 0.1787899950787401604 ) ) ;
#36828=CARTESIAN_POINT ( 'NONE',  ( -0.1797182628040039365, -0.9852800300554862556, 0.000000000000000000 ) ) ;
#36838=CARTESIAN_POINT ( 'NONE',  ( -0.1264236179284866091, -0.7829724408911181710, 0.1264236179284866091 ) ) ;
#36839=DIRECTION ( 'NONE',  ( 0.000000000000000000, 1.000000000000000000, 0.000000000000000000 ) ) ;
#36842=CARTESIAN_POINT ( 'NONE',  ( 0.1574803149606300301, -1.658956692913385655, -0.06523048226347956391 ) ) ;
#36849=CARTESIAN_POINT ( 'NONE',  ( -0.1574803149606300301, 0.05856299223351124628, -0.06523048226347956391 ) ) ;
#36850=CARTESIAN_POINT ( 'NONE',  ( 3.284318927891251994E-17, -1.452263779473795369, 0.1787899950787401882 ) ) ;
#36855=AXIS2_PLACEMENT_3D ( 'NONE', #38717, #27013, #23629 ) ;
#36859=CARTESIAN_POINT ( 'NONE',  ( 0.07975836855958620686, 0.08959396230938582173, -0.2393845553081391520 ) ) ;
#36861=CARTESIAN_POINT ( 'NONE',  ( -1.094772975963752103E-17, -0.4199074327961677122, -0.1787899950787401882 ) ) ;
#36862=CARTESIAN_POINT ( 'NONE',  ( -0.2158178664699031413, -0.08955986809707854046, 0.08935017772872932973 ) ) ;
#36872=CARTESIAN_POINT ( 'NONE',  ( -0.07405724077823318263, -1.257874015694269376, 0.1787899950787401604 ) ) ;
#36873=CARTESIAN_POINT ( 'NONE',  ( -0.07405724077823318263, -1.582677165300567346, -0.1787899950787401604 ) ) ;
#36878=CARTESIAN_POINT ( 'NONE',  ( -0.1270800023317771588, -0.6358705812365885723, -0.1270800023317771588 ) ) ;
#36882=CARTESIAN_POINT ( 'NONE',  ( -0.1113553986120547346, -0.3080708661417322913, -0.1113553986120547346 ) ) ;
#36888=CARTESIAN_POINT ( 'NONE',  ( -0.1251538622671300172, -0.09137144579352629581, -0.1276842799123791561 ) ) ;
#36891=CARTESIAN_POINT ( 'NONE',  ( -0.1113553986120547346, -0.5246062991050708391, 0.1113553986120547346 ) ) ;
#36894=CARTESIAN_POINT ( 'NONE',  ( -0.1715440989618680079, -0.08785038237295542118, -0.1863907177286787953 ) ) ;
#36901=CARTESIAN_POINT ( 'NONE',  ( -0.07405724077823318263, -1.489173228292693718, 0.1787899950787401604 ) ) ;
#36902=CARTESIAN_POINT ( 'NONE',  ( 0.1787899950787401604, -0.7706692912848194243, -0.07405724077823318263 ) ) ;
#36903=CARTESIAN_POINT ( 'NONE',  ( 2.892866454678787531E-17, -1.238188976377952777, 0.1574803149606299191 ) ) ;
#36909=VERTEX_POINT ( 'NONE', #14200 ) ;
#36920=CARTESIAN_POINT ( 'NONE',  ( 0.1113553986120547346, -0.08169291327829980576, 0.1113553986120547346 ) ) ;
#36928=CARTESIAN_POINT ( 'NONE',  ( -0.07592550097138189846, -0.09851382931116220432, 0.1427603709231669293 ) ) ;
#36934=CARTESIAN_POINT ( 'NONE',  ( -0.07405724077823318263, -0.8641732282926931630, 0.1787899950787401604 ) ) ;
#36935=CARTESIAN_POINT ( 'NONE',  ( -1.094772975963752103E-17, -0.4089566928596221063, -0.1787899950787401882 ) ) ;
#36936=CARTESIAN_POINT ( 'NONE',  ( -0.1264236179284866091, -0.9798228345919054449, 0.1264236179284866091 ) ) ;
#36937=CARTESIAN_POINT ( 'NONE',  ( -1.100456976456230270E-17, -0.2077209749373763736, -0.1797182628040039365 ) ) ;
#36938=CARTESIAN_POINT ( 'NONE',  ( -0.1113553986120547346, 0.1348425196850393804, 0.1113553986120547346 ) ) ;
#36939=CARTESIAN_POINT ( 'NONE',  ( -0.1264236179284866091, -0.01033464561552783524, -0.1264236179284866091 ) ) ;
#36943=CARTESIAN_POINT ( 'NONE',  ( -9.642888182262618425E-18, -0.03740157480314960925, -0.1574803149606299191 ) ) ;
#36950=CARTESIAN_POINT ( 'NONE',  ( 0.1574803149606300301, -0.9453740156405048278, 0.06523048226347956391 ) ) ;
#36951=CARTESIAN_POINT ( 'NONE',  ( -1.094772975963752103E-17, -0.3302165353793074520, -0.1787899950787401882 ) ) ;
#36953=CARTESIAN_POINT ( 'NONE',  ( -0.1264236179284866091, -1.019192913332062966, 0.1264236179284866091 ) ) ;
#36979=CARTESIAN_POINT ( 'NONE',  ( 0.1787899950787401604, -1.529651527284356494, -0.07405724077823318263 ) ) ;
#36981=CARTESIAN_POINT ( 'NONE',  ( 3.284318927891251994E-17, -0.3056102361667090705, 0.1787899950787401882 ) ) ;
#36991=CARTESIAN_POINT ( 'NONE',  ( 0.07405724077823318263, -1.686023621993479882, 0.1787899950787401604 ) ) ;
#36992=CARTESIAN_POINT ( 'NONE',  ( -0.07405724077823318263, -1.686023621993479882, 0.1787899950787401604 ) ) ;
#36997=CARTESIAN_POINT ( 'NONE',  ( -0.1797182628040039087, -1.415890266275959375, 0.07444174185955065859 ) ) ;
#37004=CARTESIAN_POINT ( 'NONE',  ( 0.1574803149606300301, -0.8272637794200329298, 0.06523048226347956391 ) ) ;
#37018=CARTESIAN_POINT ( 'NONE',  ( 0.1574803149606299191, -0.04724409448818897572, -1.928577636452523993E-17 ) ) ;
#37020=CARTESIAN_POINT ( 'NONE',  ( 3.301370929368692659E-17, -0.03055562060666760019, 0.1797182628040039365 ) ) ;
#37028=CARTESIAN_POINT ( 'NONE',  ( 0.07405724077823318263, -0.1309055117572600901, -0.1787899950787401604 ) ) ;
#37031=CARTESIAN_POINT ( 'NONE',  ( 0.1854358583631518231, -0.08093302715450646778, -0.1783713581459814845 ) ) ;
#37035=CARTESIAN_POINT ( 'NONE',  ( 2.892866454678787531E-17, 0.03149606309965303358, 0.1574803149606299191 ) ) ;
#37041=CARTESIAN_POINT ( 'NONE',  ( 0.1787899950787401882, -0.9415609761032539549, -2.189545951927503898E-17 ) ) ;
#37044=ORIENTED_EDGE ( 'NONE', *, *, #42296, .T. ) ;
#37051=CARTESIAN_POINT ( 'NONE',  ( -0.07444174185955065859, -1.017268219031864263, 0.1797182628040039087 ) ) ;
#37065=CARTESIAN_POINT ( 'NONE',  ( 0.07405724077823318263, -0.8395669290800948925, -0.1787899950787401604 ) ) ;
#37071=CARTESIAN_POINT ( 'NONE',  ( -0.1574803149606297803, -1.639271653543306506, 0.06523048226347956391 ) ) ;
#37078=CARTESIAN_POINT ( 'NONE',  ( 0.1113553986120547346, -0.3080708660342051375, -0.1113553986120547346 ) ) ;
#37089=CARTESIAN_POINT ( 'NONE',  ( -0.1787899950787401604, -0.4469743619300260984, 0.07405724077823318263 ) ) ;
#37090=CARTESIAN_POINT ( 'NONE',  ( -0.2150476131984622175, -0.08955971513628484260, -0.1130403609974334617 ) ) ;
#37098=CARTESIAN_POINT ( 'NONE',  ( 0.1264236179284866091, -1.329232283410803239, 0.1264236179284866091 ) ) ;
#37099=CARTESIAN_POINT ( 'NONE',  ( 0.1787899950787401604, -1.558070866087969630, 0.07405724077823318263 ) ) ;
#37109=CARTESIAN_POINT ( 'NONE',  ( 0.1113553986120547346, -0.2883858267716535306, 0.1113553986120547346 ) ) ;
#37111=CIRCLE ( 'NONE', #11106, 0.2471922904502826812 ) ;
#37114=CARTESIAN_POINT ( 'NONE',  ( -0.1174123764687494409, -0.08986489419234251763, -0.1348499909742253422 ) ) ;
#37118=CARTESIAN_POINT ( 'NONE',  ( -0.1523463298590899406, -0.08956081936279648714, 0.06373561487467800657 ) ) ;
#37125=CARTESIAN_POINT ( 'NONE',  ( -0.1264236179284866091, -1.491633858213953001, 0.1264236179284866091 ) ) ;
#37126=CARTESIAN_POINT ( 'NONE',  ( -0.1574803149606299191, -1.287401574803149540, 0.000000000000000000 ) ) ;
#37134=CARTESIAN_POINT ( 'NONE',  ( 0.1113553986120547346, -1.302165354223181026, 0.1113553986120547346 ) ) ;
#37142=CARTESIAN_POINT ( 'NONE',  ( -9.642888182262618425E-18, -0.06692913375074074911, -0.1574803149606299191 ) ) ;
#37143=CARTESIAN_POINT ( 'NONE',  ( 0.01993724539804073159, 0.05212746764708663105, 0.2739222968686834125 ) ) ;
#37151=CARTESIAN_POINT ( 'NONE',  ( -0.09426105192651733355, -0.09851383153318916952, 0.1330962383627474210 ) ) ;
#37159=CARTESIAN_POINT ( 'NONE',  ( -0.1787899950787401604, -0.9084645668753701386, 0.07405724077823318263 ) ) ;
#37162=CARTESIAN_POINT ( 'NONE',  ( -0.1787899950787401882, -1.142224409395055096, 0.000000000000000000 ) ) ;
#37164=CARTESIAN_POINT ( 'NONE',  ( 0.1797182628040039087, -0.3725831796617855018, -0.07444174185955065859 ) ) ;
#37166=CARTESIAN_POINT ( 'NONE',  ( 0.1574803149606300301, 0.1471456692913385988, 0.06523048226347956391 ) ) ;
#37173=FACE_BOUND ( 'NONE', #6979, .T. ) ;
#37181=CARTESIAN_POINT ( 'NONE',  ( -0.07405724077823318263, -0.3129921259304885850, 0.1787899950787401604 ) ) ;
#37183=CARTESIAN_POINT ( 'NONE',  ( 0.1787899950787401604, -1.238188976324190005, -0.07405724077823318263 ) ) ;
#37191=CARTESIAN_POINT ( 'NONE',  ( -0.06523048226347956391, -1.191437007766489531, 0.1574803149606297803 ) ) ;
#37193=CARTESIAN_POINT ( 'NONE',  ( -0.07175194912964910632, -0.09842519594091171664, -0.1637606677113847553 ) ) ;
#37205=ORIENTED_EDGE ( 'NONE', *, *, #21368, .T. ) ;
#37210=CARTESIAN_POINT ( 'NONE',  ( -0.1787899950787401604, -1.509966487914277788, 0.07405724077823318263 ) ) ;
#37212=CARTESIAN_POINT ( 'NONE',  ( 3.284318927891251994E-17, -0.3843503936470239468, 0.1787899950787401882 ) ) ;
#37215=CARTESIAN_POINT ( 'NONE',  ( 0.000000000000000000, -0.09842519685039370636, 0.1574803149606299191 ) ) ;
#37222=CARTESIAN_POINT ( 'NONE',  ( -0.1787899950787401604, -1.813976377898992354, 0.07405724077823318263 ) ) ;
#37223=CARTESIAN_POINT ( 'NONE',  ( -0.1787899950787401604, -1.617125984198204414, -0.07405724077823318263 ) ) ;
#37228=CARTESIAN_POINT ( 'NONE',  ( 2.892866454678787531E-17, -0.8051181102362204856, 0.1574803149606299191 ) ) ;
#37230=CARTESIAN_POINT ( 'NONE',  ( 0.1270800023317771588, -1.442957195409817039, 0.1270800023317771588 ) ) ;
#37238=FACE_OUTER_BOUND ( 'NONE', #29110, .T. ) ;
#37246=CARTESIAN_POINT ( 'NONE',  ( -0.1797182628040039087, -0.07730758911060468808, 0.07444174185955065859 ) ) ;
#37248=CARTESIAN_POINT ( 'NONE',  ( -0.1113553986120547346, -1.046259842412157637, -0.1113553986120547346 ) ) ;
#37249=CARTESIAN_POINT ( 'NONE',  ( -0.1787899950787401604, -1.223425196796630532, 0.07405724077823318263 ) ) ;
#37256=CARTESIAN_POINT ( 'NONE',  ( -0.1787899950787401604, -0.1555118109698585271, 0.07405724077823318263 ) ) ;
#37259=CARTESIAN_POINT ( 'NONE',  ( -0.1120715992846887249, -0.09842519685039369248, 0.2207285028506147662 ) ) ;
#37261=CARTESIAN_POINT ( 'NONE',  ( 0.1574803149606300301, -0.1136811022546777433, -0.06523048226347956391 ) ) ;
#37266=CARTESIAN_POINT ( 'NONE',  ( -0.1787899950787401604, -1.037525543032389974, 0.07405724077823318263 ) ) ;
#37268=CARTESIAN_POINT ( 'NONE',  ( -0.1264236179284866091, 0.08316929139234625901, 0.1264236179284866091 ) ) ;
#37277=CARTESIAN_POINT ( 'NONE',  ( -0.1270800023317771588, -1.029571368638163342, -0.1270800023317771588 ) ) ;
#37287=CARTESIAN_POINT ( 'NONE',  ( 2.892866454678787531E-17, -0.6771653542231811373, 0.1574803149606299191 ) ) ;
#37292=CARTESIAN_POINT ( 'NONE',  ( -0.1264236179284866091, -0.7140748030958424808, -0.1264236179284866091 ) ) ;
#37298=CARTESIAN_POINT ( 'NONE',  ( 0.1113553986120547346, -1.695866141732283561, -0.1113553986120547346 ) ) ;
#37305=CARTESIAN_POINT ( 'NONE',  ( 0.1574803149606300301, 0.1077755905511812162, 0.06523048226347956391 ) ) ;
#37307=CARTESIAN_POINT ( 'NONE',  ( -0.1787899950787401604, -1.459645669237573884, 0.07405724077823318263 ) ) ;
#37313=FACE_OUTER_BOUND ( 'NONE', #39316, .T. ) ;
#37314=CARTESIAN_POINT ( 'NONE',  ( 0.1439410204707495533, 0.1277165727045734556, -0.08101594287816436812 ) ) ;
#37317=CARTESIAN_POINT ( 'NONE',  ( 0.1264236179284866091, -0.5921515272843562716, 0.1264236179284866091 ) ) ;
#37318=CARTESIAN_POINT ( 'NONE',  ( -0.1577829598938297606, -0.08955953743824469904, -0.1904640068750519943 ) ) ;
#37327=CARTESIAN_POINT ( 'NONE',  ( 0.2471911001155728260, -0.08911307781772316583, 0.05219320342793875439 ) ) ;
#37332=CARTESIAN_POINT ( 'NONE',  ( 0.07405724077823318263, -1.371062992072219489, 0.1787899950787401604 ) ) ;
#37333=CARTESIAN_POINT ( 'NONE',  ( 0.1787899950787401882, -1.516240157426551161, -2.189545951927503898E-17 ) ) ;
#37338=CARTESIAN_POINT ( 'NONE',  ( 0.06523048226347956391, -0.2760826771653543954, -0.1574803149606300301 ) ) ;
#37347=CARTESIAN_POINT ( 'NONE',  ( -0.1461630486916919713, -0.08955915398144619066, 0.07502663895056801979 ) ) ;
#37352=CARTESIAN_POINT ( 'NONE',  ( -0.1093692153654682031, 0.09774221684002692978, -0.2222887249338305893 ) ) ;
#37353=CARTESIAN_POINT ( 'NONE',  ( -0.1574803149606300301, -0.03001968503937006705, -0.06523048226347956391 ) ) ;
#37354=CARTESIAN_POINT ( 'NONE',  ( -0.07405724077823318263, -1.503937007820251637, -0.1787899950787401604 ) ) ;
#37355=CARTESIAN_POINT ( 'NONE',  ( 0.1264236179284866091, -0.8961614172690708369, 0.1264236179284866091 ) ) ;
#37356=CARTESIAN_POINT ( 'NONE',  ( 0.1574803149606300301, -1.225885826771653697, -0.06523048226347956391 ) ) ;
#37364=CARTESIAN_POINT ( 'NONE',  ( 0.1574803149606299191, -1.297244094380661350, -1.928577636452523993E-17 ) ) ;
#37380=CARTESIAN_POINT ( 'NONE',  ( -0.2340881785939889770, -0.09842519685039370636, -0.07097624971890235945 ) ) ;
#37388=CARTESIAN_POINT ( 'NONE',  ( 0.1787899950787401882, -0.8912401574265511606, -2.189545951927503898E-17 ) ) ;
#37390=CARTESIAN_POINT ( 'NONE',  ( 0.07405724077823318263, -1.011811023568284451, 0.1787899950787401604 ) ) ;
#37395=CARTESIAN_POINT ( 'NONE',  ( -0.1797182628040039087, -0.2741579828113920869, 0.07444174185955065859 ) ) ;
#37401=FACE_OUTER_BOUND ( 'NONE', #10579, .T. ) ;
#37406=CARTESIAN_POINT ( 'NONE',  ( -0.1574803149606297803, -0.9601377951680625245, 0.06523048226347956391 ) ) ;
#37407=CARTESIAN_POINT ( 'NONE',  ( 0.1264236179284866091, -0.2957677164816697180, -0.1264236179284866091 ) ) ;
#37409=CARTESIAN_POINT ( 'NONE',  ( 0.07405724077823318263, -1.287401574749386768, 0.1787899950787401604 ) ) ;
#37419=CARTESIAN_POINT ( 'NONE',  ( -0.1574803149606299191, -1.198818897530267824, 0.000000000000000000 ) ) ;
#37425=CARTESIAN_POINT ( 'NONE',  ( -0.008273236941784495660, -0.09842493939591641372, -0.1788444388497219262 ) ) ;
#37446=CARTESIAN_POINT ( 'NONE',  ( 0.1787899950787401604, -1.495202708386720092, 0.07405724077823318263 ) ) ;
#37449=CARTESIAN_POINT ( 'NONE',  ( 0.1264236179284866091, -0.4187992125446614589, 0.1264236179284866091 ) ) ;
#37451=ORIENTED_EDGE ( 'NONE', *, *, #9215, .F. ) ;
#37459=CARTESIAN_POINT ( 'NONE',  ( -0.1264236179284866091, 0.09682485066839900678, -0.1264236179284866091 ) ) ;
#37460=CARTESIAN_POINT ( 'NONE',  ( -0.1787899950787401604, -1.656496062938362268, -0.07405724077823318263 ) ) ;
#37466=CARTESIAN_POINT ( 'NONE',  ( -9.642888182262618425E-18, -0.7066929133858268486, -0.1574803149606299191 ) ) ;
#37468=CARTESIAN_POINT ( 'NONE',  ( -0.07444174185955065859, -1.371598927693281844, 0.1797182628040039087 ) ) ;
#37477=LINE ( 'NONE', #23808, #21337 ) ;
#37487=CARTESIAN_POINT ( 'NONE',  ( -9.642888182262618425E-18, -0.03740157480314960925, -0.1574803149606299191 ) ) ;
#37489=CARTESIAN_POINT ( 'NONE',  ( 0.1797182628040039087, -0.05762254974052589268, -0.07444174185955065859 ) ) ;
#37490=CARTESIAN_POINT ( 'NONE',  ( -0.07405724077823318263, -1.154527559001354842, -0.1787899950787401604 ) ) ;
#37500=CARTESIAN_POINT ( 'NONE',  ( -0.08392772586492357190, -0.09126532511089867350, -0.2369773207361680067 ) ) ;
#37503=CARTESIAN_POINT ( 'NONE',  ( 0.1113553986120547346, -0.1210629920184572855, 0.1113553986120547346 ) ) ;
#37511=CARTESIAN_POINT ( 'NONE',  ( -0.1787899950787401882, -1.000616094213490292, 0.000000000000000000 ) ) ;
#37513=CARTESIAN_POINT ( 'NONE',  ( 0.07405724077823318263, 0.1053149606836847191, -0.1787899950787401604 ) ) ;
#37519=CARTESIAN_POINT ( 'NONE',  ( 0.1264236179284866091, -0.5024606298674960669, 0.1264236179284866091 ) ) ;
#37524=CARTESIAN_POINT ( 'NONE',  ( 3.301370929368692659E-17, -0.9754375103704467920, 0.1797182628040039365 ) ) ;
#37536=CARTESIAN_POINT ( 'NONE',  ( -0.1264236179284866091, -0.7928149605761574126, -0.1264236179284866091 ) ) ;
#37540=CARTESIAN_POINT ( 'NONE',  ( 0.1113553986120547346, -1.607283464459401401, -0.1113553986120547346 ) ) ;
#37543=CARTESIAN_POINT ( 'NONE',  ( 0.1113553986120547346, -1.745078740157480546, 0.1113553986120547346 ) ) ;
#37550=CARTESIAN_POINT ( 'NONE',  ( -0.06523048226347956391, -0.3646653542231817480, 0.1574803149606297803 ) ) ;
#37551=CARTESIAN_POINT ( 'NONE',  ( 3.284318927891251994E-17, -1.609744094434425232, 0.1787899950787401882 ) ) ;
#37562=CARTESIAN_POINT ( 'NONE',  ( 0.1787899950787401882, -0.6266003461819942277, -2.189545951927503898E-17 ) ) ;
#37563=CARTESIAN_POINT ( 'NONE',  ( -0.1975987513857511702, -0.08955961876119605813, -0.1443798108109194955 ) ) ;
#37569=LINE ( 'NONE', #33780, #36057 ) ;
#37571=CARTESIAN_POINT ( 'NONE',  ( -0.1787899950787401882, -1.383366141678519678, 0.000000000000000000 ) ) ;
#37573=CARTESIAN_POINT ( 'NONE',  ( 0.1787899950787401604, -1.479330708607653699, 0.07405724077823318263 ) ) ;
#37579=CARTESIAN_POINT ( 'NONE',  ( 0.06523048226347956391, -0.3154527559055120278, -0.1574803149606300301 ) ) ;
#37587=DIRECTION ( 'NONE',  ( 0.000000000000000000, 1.000000000000000000, 0.000000000000000000 ) ) ;
#37592=CARTESIAN_POINT ( 'NONE',  ( -0.1481685473978694711, -0.08955954485027488310, 0.07164615537806104384 ) ) ;
#37599=CARTESIAN_POINT ( 'NONE',  ( -0.08994717584591646609, 0.09317026862874071280, -0.2335020446786553738 ) ) ;
#37601=CARTESIAN_POINT ( 'NONE',  ( 0.1787899950787401604, -1.671259842465922407, -0.07405724077823318263 ) ) ;
#37602=CARTESIAN_POINT ( 'NONE',  ( -0.1264236179284866091, -0.8764763778989921317, -0.1264236179284866091 ) ) ;
#37604=CARTESIAN_POINT ( 'NONE',  ( 0.1574803149606299191, -1.267716535433070835, -1.928577636452523993E-17 ) ) ;
#37608=VERTEX_POINT ( 'NONE', #46716 ) ;
#37612=CARTESIAN_POINT ( 'NONE',  ( -0.1113553986120547346, -1.312007873908220379, 0.1113553986120547346 ) ) ;
#37621=CARTESIAN_POINT ( 'NONE',  ( 0.03894127257533385594, 0.06746187776217156540, 0.2629503166621862120 ) ) ;
#37628=CARTESIAN_POINT ( 'NONE',  ( -0.1459848668369287394, -0.09851383230118682111, 0.08268675942001851853 ) ) ;
#37638=CARTESIAN_POINT ( 'NONE',  ( -0.1264236179284866091, -0.8371062991588346103, -0.1264236179284866091 ) ) ;
#37639=CARTESIAN_POINT ( 'NONE',  ( 0.1264236179284866091, -1.078248031442299304, -0.1264236179284866091 ) ) ;
#37642=CARTESIAN_POINT ( 'NONE',  ( 0.1270800023317771588, -0.3012249119452504176, 0.1270800023317771588 ) ) ;
#37643=CARTESIAN_POINT ( 'NONE',  ( 0.1113553986120547346, -1.804133858160189119, -0.1113553986120547346 ) ) ;
#37644=CARTESIAN_POINT ( 'NONE',  ( 0.06523048226347956391, 0.1422244094488189503, 0.1574803149606297803 ) ) ;
#37645=CARTESIAN_POINT ( 'NONE',  ( 0.07405724077823318263, -0.1505905511273389341, 0.1787899950787401604 ) ) ;
#37649=CARTESIAN_POINT ( 'NONE',  ( -9.642888182262618425E-18, -0.02755905501058318954, -0.1574803149606299191 ) ) ;
#37658=CARTESIAN_POINT ( 'NONE',  ( -0.07405724077823318263, -0.4458661416785199560, -0.1787899950787401604 ) ) ;
#37660=CARTESIAN_POINT ( 'NONE',  ( -0.07405724077823318263, -1.228346456639149542, -0.1787899950787401604 ) ) ;
#37673=CARTESIAN_POINT ( 'NONE',  ( -0.1360271360007213048, -0.09844179429577380736, -0.1161711393741745174 ) ) ;
#37689=CARTESIAN_POINT ( 'NONE',  ( -1.094772975963752103E-17, -1.404159401300104415, -0.1787899950787401882 ) ) ;
#37691=CARTESIAN_POINT ( 'NONE',  ( -1.094772975963752103E-17, -0.4827755904974173617, -0.1787899950787401882 ) ) ;
#37701=CARTESIAN_POINT ( 'NONE',  ( -0.1787899950787401882, -1.816437007820251859, 0.000000000000000000 ) ) ;
#37702=CARTESIAN_POINT ( 'NONE',  ( 0.1787899950787401604, -1.794291338528913426, 0.07405724077823318263 ) ) ;
#37707=CARTESIAN_POINT ( 'NONE',  ( -0.1574803149606299191, -0.6968503937007873850, 0.000000000000000000 ) ) ;
#37708=CARTESIAN_POINT ( 'NONE',  ( 0.1797182628040039365, -1.398665856827139731, -2.200913952912460540E-17 ) ) ;
#37710=CARTESIAN_POINT ( 'NONE',  ( -9.642888182262618425E-18, -0.4606299211523149362, -0.1574803149606299191 ) ) ;
#37722=CARTESIAN_POINT ( 'NONE',  ( -0.07405724077823318263, -0.03740157474938609478, 0.1787899950787401604 ) ) ;
#37732=CARTESIAN_POINT ( 'NONE',  ( -0.1797182628040039087, -0.03793751037044712504, 0.07444174185955065859 ) ) ;
#37733=CARTESIAN_POINT ( 'NONE',  ( 0.1264236179284866091, -1.250492125930488196, 0.1264236179284866091 ) ) ;
#37745=CARTESIAN_POINT ( 'NONE',  ( -0.1574803149606300301, -0.05954724398696115140, -0.06523048226347956391 ) ) ;
#37755=CARTESIAN_POINT ( 'NONE',  ( -0.1264236179284866091, -0.9169546768906554624, 0.1264236179284866091 ) ) ;
#37757=CARTESIAN_POINT ( 'NONE',  ( -0.1787899950787401604, -0.002952755851748307785, -0.07405724077823318263 ) ) ;
#37763=CARTESIAN_POINT ( 'NONE',  ( 0.1787899950787401604, -0.6968503936470246130, 0.07405724077823318263 ) ) ;
#37764=EDGE_CURVE ( 'NONE', #4939, #43211, #26411, .T. ) ;
#37767=DIRECTION ( 'NONE',  ( 0.000000000000000000, -1.000000000000000000, 0.000000000000000000 ) ) ;
#37768=CARTESIAN_POINT ( 'NONE',  ( -0.1797182628040039365, -1.024650108795643666, 0.000000000000000000 ) ) ;
#37779=CARTESIAN_POINT ( 'NONE',  ( 0.1574803149606300301, -0.6697834644594027331, 0.06523048226347956391 ) ) ;
#37780=CARTESIAN_POINT ( 'NONE',  ( 0.07405724077823318263, 0.1053149606836847191, -0.1787899950787401604 ) ) ;
#37785=CARTESIAN_POINT ( 'NONE',  ( -0.07405724077823318263, -0.9379921259304876413, 0.1787899950787401604 ) ) ;
#37790=CARTESIAN_POINT ( 'NONE',  ( -9.642888182262618425E-18, -1.759842519577511810, -0.1574803149606299191 ) ) ;
#37792=CARTESIAN_POINT ( 'NONE',  ( -8.354793841626791791E-17, -0.09842519685039370636, -0.2854330708661417804 ) ) ;
#37795=CARTESIAN_POINT ( 'NONE',  ( 0.1574803149606300301, -1.619586614173227579, -0.06523048226347956391 ) ) ;
#37799=CARTESIAN_POINT ( 'NONE',  ( -0.1113553986120547346, -0.3375984250893232508, -0.1113553986120547346 ) ) ;
#37800=CARTESIAN_POINT ( 'NONE',  ( -0.1264236179284866091, -1.545767716481669218, -0.1264236179284866091 ) ) ;
#37809=CARTESIAN_POINT ( 'NONE',  ( -0.1787899950787401604, -0.5306357792528606510, -0.07405724077823318263 ) ) ;
#37810=CARTESIAN_POINT ( 'NONE',  ( 0.08588050461400061064, -0.08956016273386613324, 0.1986011934319732164 ) ) ;
#37811=CARTESIAN_POINT ( 'NONE',  ( -9.642888182262618425E-18, 0.05118110246973173183, -0.1574803149606299191 ) ) ;
#37818=CARTESIAN_POINT ( 'NONE',  ( 0.2471922963015218966, -0.09312803950197923175, 0.03901180619690218510 ) ) ;
#37821=CARTESIAN_POINT ( 'NONE',  ( -0.07405724077823318263, -1.508858267662772867, -0.1787899950787401604 ) ) ;
#37822=CARTESIAN_POINT ( 'NONE',  ( -0.1787899950787401882, -1.535925196796629866, 0.000000000000000000 ) ) ;
#37826=ORIENTED_EDGE ( 'NONE', *, *, #14578, .F. ) ;
#37831=CARTESIAN_POINT ( 'NONE',  ( 0.1574803149606299191, -0.2440944881889763884, -1.928577636452523993E-17 ) ) ;
#37836=CARTESIAN_POINT ( 'NONE',  ( -0.1267356318029559670, -0.09168894753733079772, -0.1261112482890841824 ) ) ;
#37842=CARTESIAN_POINT ( 'NONE',  ( -0.09445526594068323623, -0.08956264882496832447, 0.1283258905068025424 ) ) ;
#37843=CARTESIAN_POINT ( 'NONE',  ( -0.1787899950787401604, -0.5098425196312756924, 0.07405724077823318263 ) ) ;
#37853=CARTESIAN_POINT ( 'NONE',  ( -0.1264236179284866091, -0.8666338582139527791, 0.1264236179284866091 ) ) ;
#37854=CARTESIAN_POINT ( 'NONE',  ( -0.1574803149606299191, -1.169291338582677309, 0.000000000000000000 ) ) ;
#37863=CARTESIAN_POINT ( 'NONE',  ( -0.06523048226347956391, -1.388287401467275917, 0.1574803149606297803 ) ) ;
#37878=CARTESIAN_POINT ( 'NONE',  ( -0.1097920307064556983, -0.09842519685039370636, -0.2293370477459909240 ) ) ;
#37883=CARTESIAN_POINT ( 'NONE',  ( -0.1264236179284866091, -0.9453740156942677109, 0.1264236179284866091 ) ) ;
#37884=CARTESIAN_POINT ( 'NONE',  ( 0.1264236179284866091, -0.9995078739619842612, -0.1264236179284866091 ) ) ;
#37886=CARTESIAN_POINT ( 'NONE',  ( 0.1797182628040039087, -0.3332131009216283135, -0.07444174185955065859 ) ) ;
#37887=CARTESIAN_POINT ( 'NONE',  ( -0.1113553986120547346, -1.794291338475149766, -0.1113553986120547346 ) ) ;
#37888=CARTESIAN_POINT ( 'NONE',  ( -9.642888182262618425E-18, 0.1594488188976377896, -0.1574803149606299191 ) ) ;
#37889=CARTESIAN_POINT ( 'NONE',  ( 0.07405724077823318263, -0.1751968503399373434, -0.1787899950787401604 ) ) ;
#37899=CARTESIAN_POINT ( 'NONE',  ( -0.1787899950787401604, -0.3622047243556850704, -0.07405724077823318263 ) ) ;
#37901=CARTESIAN_POINT ( 'NONE',  ( -0.1787899950787401882, -1.181594488135212506, 0.000000000000000000 ) ) ;
#37914=CARTESIAN_POINT ( 'NONE',  ( 0.03838706947536870556, -0.09842268942605733595, -0.1746209144150240034 ) ) ;
#37925=ORIENTED_EDGE ( 'NONE', *, *, #19900, .F. ) ;
#37930=CARTESIAN_POINT ( 'NONE',  ( -0.1787899950787401882, -1.512427117835537516, 0.000000000000000000 ) ) ;
#37933=CARTESIAN_POINT ( 'NONE',  ( 0.1787899950787401882, -0.4138779527021417826, -2.189545951927503898E-17 ) ) ;
#37944=CARTESIAN_POINT ( 'NONE',  ( -0.1264236179284866091, -1.811515747977732405, 0.1264236179284866091 ) ) ;
#37945=CARTESIAN_POINT ( 'NONE',  ( -0.1787899950787401604, -1.769685039316315267, 0.07405724077823318263 ) ) ;
#37946=CARTESIAN_POINT ( 'NONE',  ( 0.1595297091834116943, -0.09842519685039372024, 0.06859577724087914663 ) ) ;
#37949=CARTESIAN_POINT ( 'NONE',  ( 0.1113553986120547346, -0.7903543307086614567, -0.1113553986120547346 ) ) ;
#37951=CARTESIAN_POINT ( 'NONE',  ( -0.1270800023317771588, -1.610280030055486034, 0.1270800023317771588 ) ) ;
#37961=CARTESIAN_POINT ( 'NONE',  ( 0.1264236179284866091, 0.05856299217974780119, -0.1264236179284866091 ) ) ;
#37981=CARTESIAN_POINT ( 'NONE',  ( -0.05836929678884612144, -0.07899262986803357034, -0.2517335218907394978 ) ) ;
#37984=CARTESIAN_POINT ( 'NONE',  ( -0.1113553986120547346, 0.01673228357209397693, -0.1113553986120547346 ) ) ;
#37988=CARTESIAN_POINT ( 'NONE',  ( 0.07405724077823318263, -0.9489428658670333583, 0.1787899950787401604 ) ) ;
#37990=CARTESIAN_POINT ( 'NONE',  ( 0.1787899950787401882, 0.09793307091990532953, -2.189545951927503898E-17 ) ) ;
#37997=CARTESIAN_POINT ( 'NONE',  ( 0.1787899950787401604, -0.6181102361667089040, 0.07405724077823318263 ) ) ;
#38001=CARTESIAN_POINT ( 'NONE',  ( -0.1270800023317771588, -1.137839085173596443, 0.1270800023317771588 ) ) ;
#38010=CARTESIAN_POINT ( 'NONE',  ( 0.1787899950787401882, 0.09793307091990532953, -2.189545951927503898E-17 ) ) ;
#38019=CARTESIAN_POINT ( 'NONE',  ( 0.06523048226347956391, -1.762303149498772425, -0.1574803149606300301 ) ) ;
#38021=EDGE_LOOP ( 'NONE', ( #28677, #46566, #2662, #45076 ) ) ;
#38024=CARTESIAN_POINT ( 'NONE',  ( 0.07405724077823318263, 0.1053149606836847191, -0.1787899950787401604 ) ) ;
#38030=ORIENTED_EDGE ( 'NONE', *, *, #380, .T. ) ;
#38031=CARTESIAN_POINT ( 'NONE',  ( -0.1264236179284866091, -1.506397637741511586, -0.1264236179284866091 ) ) ;
#38040=CARTESIAN_POINT ( 'NONE',  ( 0.1264236179284866091, -0.5429389288591598417, -0.1264236179284866091 ) ) ;
#38041=CARTESIAN_POINT ( 'NONE',  ( 0.1884186337727752070, -0.08956031548849312240, 0.08950290581337028151 ) ) ;
#38048=CARTESIAN_POINT ( 'NONE',  ( 0.2471922904502823481, -0.05170400041210165137, 0.1201839652823721433 ) ) ;
#38050=CARTESIAN_POINT ( 'NONE',  ( 0.1787899950787401882, -1.521161417269070837, -2.189545951927503898E-17 ) ) ;
#38060=CARTESIAN_POINT ( 'NONE',  ( 0.1113553986120547346, -0.4064960629921260393, 0.1113553986120547346 ) ) ;
#38064=CARTESIAN_POINT ( 'NONE',  ( 0.1113553986120547346, 0.03641732283464567399, -0.1113553986120547346 ) ) ;
#38069=CARTESIAN_POINT ( 'NONE',  ( 2.892866454678787531E-17, -0.5590551180027086842, 0.1574803149606299191 ) ) ;
#38073=CARTESIAN_POINT ( 'NONE',  ( -0.1690116988092786321, -0.08956104861086600089, -0.02641944785140138904 ) ) ;
#38074=CARTESIAN_POINT ( 'NONE',  ( -0.1787899950787401882, -0.5910433070328504623, 0.000000000000000000 ) ) ;
#38080=CARTESIAN_POINT ( 'NONE',  ( -0.09072581850463902475, 0.09340956239926205551, -0.2330524951300393943 ) ) ;
#38082=CARTESIAN_POINT ( 'NONE',  ( -0.1787899950787401882, -1.732775590497417362, 0.000000000000000000 ) ) ;
#38083=CARTESIAN_POINT ( 'NONE',  ( 0.1264236179284866091, -0.9650590550643465271, -0.1264236179284866091 ) ) ;
#38084=CARTESIAN_POINT ( 'NONE',  ( 0.1574803149606300301, -1.348917322834644938, 0.06523048226347956391 ) ) ;
#38088=ORIENTED_EDGE ( 'NONE', *, *, #43772, .F. ) ;
#38095=EDGE_CURVE ( 'NONE', #3096, #36213, #24789, .T. ) ;
#38105=CARTESIAN_POINT ( 'NONE',  ( 0.2014288353937744303, -0.09842519685039370636, 0.06137064346568976703 ) ) ;
#38114=CARTESIAN_POINT ( 'NONE',  ( -0.07405724077823318263, -0.9970472440407247561, -0.1787899950787401604 ) ) ;
#38115=CARTESIAN_POINT ( 'NONE',  ( 3.284318927891251994E-17, -1.132381889710015743, 0.1787899950787401882 ) ) ;
#38120=CARTESIAN_POINT ( 'NONE',  ( 0.1270800023317771588, -0.4193351481657228152, 0.1270800023317771588 ) ) ;
#38122=CARTESIAN_POINT ( 'NONE',  ( 0.1113553986120547346, -0.05216535433070866590, 0.1113553986120547346 ) ) ;
#38130=CARTESIAN_POINT ( 'NONE',  ( 0.07405724077823318263, -0.4507874015210400209, -0.1787899950787401604 ) ) ;
#38132=CARTESIAN_POINT ( 'NONE',  ( -0.1787899950787401882, -1.339074803095842592, 0.000000000000000000 ) ) ;
#38139=CARTESIAN_POINT ( 'NONE',  ( 0.06628613000900354657, -0.09842519684894961152, -0.1660483457538282914 ) ) ;
#38157=CARTESIAN_POINT ( 'NONE',  ( -0.07405724077823318263, -0.3622047243556850704, -0.1787899950787401604 ) ) ;
#38162=CARTESIAN_POINT ( 'NONE',  ( -1.094772975963752103E-17, -0.2514763778989925203, -0.1787899950787401882 ) ) ;
#38164=CARTESIAN_POINT ( 'NONE',  ( 0.1787899950787401604, 0.1189705199597376750, 0.07405724077823318263 ) ) ;
#38169=CARTESIAN_POINT ( 'NONE',  ( -0.1113553986120547346, -0.7411417322834646937, -0.1113553986120547346 ) ) ;
#38171=CARTESIAN_POINT ( 'NONE',  ( 0.1270800023317771588, -1.561067431630289271, 0.1270800023317771588 ) ) ;
#38173=CARTESIAN_POINT ( 'NONE',  ( -0.06523048226347956391, -0.4581692912310550425, -0.1574803149606300301 ) ) ;
#38175=CARTESIAN_POINT ( 'NONE',  ( -0.07405724077823318263, -0.3622047243556850704, -0.1787899950787401604 ) ) ;
#38185=CARTESIAN_POINT ( 'NONE',  ( -0.1264236179284866091, -0.01033464561552783524, -0.1264236179284866091 ) ) ;
#38198=CARTESIAN_POINT ( 'NONE',  ( -0.1787899950787401604, -1.307086614119465695, -0.07405724077823318263 ) ) ;
#38214=CARTESIAN_POINT ( 'NONE',  ( 0.1574803149606300301, -0.07923228335703978720, 0.06523048226347956391 ) ) ;
#38221=CARTESIAN_POINT ( 'NONE',  ( 0.07405724077823318263, -1.209769637520577312, -0.1787899950787401604 ) ) ;
#38223=CARTESIAN_POINT ( 'NONE',  ( 3.284318927891251994E-17, -0.03001968498560657339, 0.1787899950787401882 ) ) ;
#38232=CARTESIAN_POINT ( 'NONE',  ( 0.07405724077823318263, -0.6230314960092281362, 0.1787899950787401604 ) ) ;
#38235=CARTESIAN_POINT ( 'NONE',  ( 3.301370929368692659E-17, -1.093547746590919356, 0.1797182628040039365 ) ) ;
#38236=CARTESIAN_POINT ( 'NONE',  ( 0.1558288391422229802, 0.1299212598425196485, -0.06817221290114469645 ) ) ;
#38253=CARTESIAN_POINT ( 'NONE',  ( -0.1574803149606297803, -1.629429133750740721, 0.06523048226347956391 ) ) ;
#38258=CARTESIAN_POINT ( 'NONE',  ( -1.094772975963752103E-17, 0.1471456693451021758, -0.1787899950787401882 ) ) ;
#38265=CARTESIAN_POINT ( 'NONE',  ( -0.1787899950787401604, -1.582677165300567346, -0.07405724077823318263 ) ) ;
#38273=CARTESIAN_POINT ( 'NONE',  ( 0.07405724077823318263, -0.5011082201977427042, -0.1787899950787401604 ) ) ;
#38274=CARTESIAN_POINT ( 'NONE',  ( 0.1082782017465728358, -0.08956058681966397317, -0.1600574421723590657 ) ) ;
#38277=CARTESIAN_POINT ( 'NONE',  ( -0.05739891189368035579, -0.09221798112689158500, 0.1474577068024042759 ) ) ;
#38279=DIRECTION ( 'NONE',  ( 0.000000000000000000, 1.000000000000000000, 0.000000000000000000 ) ) ;
#38283=CARTESIAN_POINT ( 'NONE',  ( -0.1787899950787401604, -1.538385826717890703, 0.07405724077823318263 ) ) ;
#38284=AXIS2_PLACEMENT_3D ( 'NONE', #23724, #16075, #30938 ) ;
#38287=DIRECTION ( 'NONE',  ( 0.000000000000000000, -1.000000000000000000, 0.000000000000000000 ) ) ;
#38294=CARTESIAN_POINT ( 'NONE',  ( 0.1574803149606300301, -0.3597440944881892810, -0.06523048226347956391 ) ) ;
#38311=CARTESIAN_POINT ( 'NONE',  ( -0.06523048226347956391, -0.02017716535433068670, 0.1574803149606297803 ) ) ;
#38312=CARTESIAN_POINT ( 'NONE',  ( 0.1264236179284866091, -1.747539370024976391, -0.1264236179284866091 ) ) ;
#38313=CARTESIAN_POINT ( 'NONE',  ( -0.1787899950787401882, -0.9502952755367874982, 0.000000000000000000 ) ) ;
#38314=CARTESIAN_POINT ( 'NONE',  ( 0.1113553986120547346, -1.312007874015748143, 0.1113553986120547346 ) ) ;
#38335=CARTESIAN_POINT ( 'NONE',  ( 0.0007090829129236239431, -0.09842519685039370636, -0.1903984615526421176 ) ) ;
#38340=CARTESIAN_POINT ( 'NONE',  ( -0.1787899950787401604, -1.070866141678519456, -0.07405724077823318263 ) ) ;
#38341=CARTESIAN_POINT ( 'NONE',  ( -0.1787899950787401604, -1.184055118056472455, -0.07405724077823318263 ) ) ;
#38344=CARTESIAN_POINT ( 'NONE',  ( 0.1270800023317771588, -0.4980753056460377470, 0.1270800023317771588 ) ) ;
#38345=CARTESIAN_POINT ( 'NONE',  ( -0.1113553986120547346, -1.784448818790110192, 0.1113553986120547346 ) ) ;
#38347=CARTESIAN_POINT ( 'NONE',  ( -9.642888182262618425E-18, 0.04133858267716535029, -0.1574803149606299191 ) ) ;
#38360=CARTESIAN_POINT ( 'NONE',  ( 0.1787899950787401604, -0.3818897637257640532, 0.07405724077823318263 ) ) ;
#38362=CARTESIAN_POINT ( 'NONE',  ( -0.1787899950787401882, -1.417814960576157635, 0.000000000000000000 ) ) ;
#38364=ORIENTED_EDGE ( 'NONE', *, *, #586, .T. ) ;
#38376=CARTESIAN_POINT ( 'NONE',  ( -0.06756161724086527653, -0.08412760742771717426, 0.2464250160562324043 ) ) ;
#38382=CARTESIAN_POINT ( 'NONE',  ( 0.05363520799883866180, -0.09851384801570906014, 0.2150731022931543224 ) ) ;
#38391=CARTESIAN_POINT ( 'NONE',  ( 0.07405724077823318263, -1.642840503662309493, -0.1787899950787401604 ) ) ;
#38392=ORIENTED_EDGE ( 'NONE', *, *, #6371, .T. ) ;
#38394=CARTESIAN_POINT ( 'NONE',  ( -0.07405724077823318263, -0.5836614172690718361, 0.1787899950787401604 ) ) ;
#38400=CARTESIAN_POINT ( 'NONE',  ( 0.07405724077823318263, -0.8149606298674965110, 0.1787899950787401604 ) ) ;
#38403=CARTESIAN_POINT ( 'NONE',  ( 0.1264236179284866091, -0.04097042492215212384, 0.1264236179284866091 ) ) ;
#38404=CARTESIAN_POINT ( 'NONE',  ( -0.07405724077823318263, -1.764763779473795813, 0.1787899950787401604 ) ) ;
#38412=CARTESIAN_POINT ( 'NONE',  ( 0.1574803149606300301, -0.9502952755905519355, -0.06523048226347956391 ) ) ;
#38414=CARTESIAN_POINT ( 'NONE',  ( 0.1797182628040039087, -1.597976880449187398, 0.07444174185955046430 ) ) ;
#38416=CARTESIAN_POINT ( 'NONE',  ( 0.07405724077823318263, -0.4212598424659216856, 0.1787899950787401604 ) ) ;
#38427=DIRECTION ( 'NONE',  ( 0.000000000000000000, 1.000000000000000000, 0.000000000000000000 ) ) ;
#38428=CARTESIAN_POINT ( 'NONE',  ( 0.1787899950787401604, 0.01673228351833045899, -0.07405724077823318263 ) ) ;
#38438=CARTESIAN_POINT ( 'NONE',  ( 0.1574803149606299191, -1.100393700679874076, -1.928577636452523993E-17 ) ) ;
#38439=CARTESIAN_POINT ( 'NONE',  ( -0.1787899950787401604, -1.380905511757260173, 0.07405724077823318263 ) ) ;
#38449=DIRECTION ( 'NONE',  ( 0.000000000000000000, 1.000000000000000000, 0.000000000000000000 ) ) ;
#38452=CARTESIAN_POINT ( 'NONE',  ( 0.1113553986120547346, -0.2293307085538901779, -0.1113553986120547346 ) ) ;
#38457=CARTESIAN_POINT ( 'NONE',  ( 0.1787899950787401604, -1.219612157205616221, 0.07405724077823318263 ) ) ;
#38459=CARTESIAN_POINT ( 'NONE',  ( 0.1787899950787401882, -0.1776574802611972648, -2.189545951927503898E-17 ) ) ;
#38467=CARTESIAN_POINT ( 'NONE',  ( -0.1787899950787401604, -0.6771653542769455747, -0.07405724077823318263 ) ) ;
#38472=CARTESIAN_POINT ( 'NONE',  ( -0.07444174185955065859, -1.096008376512180194, 0.1797182628040039087 ) ) ;
#38492=CARTESIAN_POINT ( 'NONE',  ( 0.1574803149606300301, -1.654035432963339103, 0.06523048226347956391 ) ) ;
#38495=CARTESIAN_POINT ( 'NONE',  ( -1.094772975963752103E-17, 0.06840551186478720236, -0.1787899950787401882 ) ) ;
#38499=CARTESIAN_POINT ( 'NONE',  ( -0.05473164110560591739, 0.07681961335491412080, 0.2538337431406300637 ) ) ;
#38502=CARTESIAN_POINT ( 'NONE',  ( 0.1113553986120547346, -0.3572834644594020115, 0.1113553986120547346 ) ) ;
#38503=CARTESIAN_POINT ( 'NONE',  ( -0.1787899950787401604, -1.700787401521039355, -0.07405724077823318263 ) ) ;
#38512=ORIENTED_EDGE ( 'NONE', *, *, #26554, .T. ) ;
#38513=CARTESIAN_POINT ( 'NONE',  ( -0.1693402938160395443, -0.08956121756881751939, -0.02606734845562425421 ) ) ;
#38516=CARTESIAN_POINT ( 'NONE',  ( -0.2471922904502826812, -0.03219022224904098672, -0.1427165354330708902 ) ) ;
#38518=CARTESIAN_POINT ( 'NONE',  ( 0.1113553986120547346, 0.06594488188976378729, 0.1113553986120547346 ) ) ;
#38525=CARTESIAN_POINT ( 'NONE',  ( -0.1264236179284866091, -1.417814960576157635, 0.1264236179284866091 ) ) ;
#38529=CARTESIAN_POINT ( 'NONE',  ( 0.1270800023317771588, -0.6850831796617854463, -0.1270800023317771588 ) ) ;
#38533=CARTESIAN_POINT ( 'NONE',  ( 0.06523048226347956391, -0.4729330708661419469, -0.1574803149606300301 ) ) ;
#38548=CARTESIAN_POINT ( 'NONE',  ( -0.1684572903745232830, -0.08956285536357470878, -0.03266174313778202887 ) ) ;
#38549=CARTESIAN_POINT ( 'NONE',  ( 0.07405724077823318263, -0.5639763778989922427, -0.1787899950787401604 ) ) ;
#38557=CARTESIAN_POINT ( 'NONE',  ( 0.1264236179284866091, -1.786909448765134023, -0.1264236179284866091 ) ) ;
#38558=CARTESIAN_POINT ( 'NONE',  ( -0.1264236179284866091, -1.112696850339937038, -0.1264236179284866091 ) ) ;
#38559=CARTESIAN_POINT ( 'NONE',  ( 0.06523048226347956391, -1.339074803149606474, -0.1574803149606300301 ) ) ;
#38566=VERTEX_POINT ( 'NONE', #41343 ) ;
#38577=CARTESIAN_POINT ( 'NONE',  ( 0.1778667912632992121, -0.09842519685039370636, 0.1186629878957504020 ) ) ;
#38578=CARTESIAN_POINT ( 'NONE',  ( -0.06523048226347956391, 0.004429133858267709535, -0.1574803149606300301 ) ) ;
#38580=ORIENTED_EDGE ( 'NONE', *, *, #7959, .T. ) ;
#38581=EDGE_CURVE ( 'NONE', #23021, #22067, #620, .T. ) ;
#38583=CARTESIAN_POINT ( 'NONE',  ( -1.094772975963752103E-17, -0.9995078739619842612, -0.1787899950787401882 ) ) ;
#38584=CARTESIAN_POINT ( 'NONE',  ( 0.07405724077823318263, -1.248031496009228913, 0.1787899950787401604 ) ) ;
#38586=CARTESIAN_POINT ( 'NONE',  ( -0.07444174185955065859, -0.4808508961972187135, -0.1797182628040039087 ) ) ;
#38587=CARTESIAN_POINT ( 'NONE',  ( -0.1113553986120547346, -1.823818897530267602, 0.1113553986120547346 ) ) ;
#38590=CARTESIAN_POINT ( 'NONE',  ( 0.1113553986120547346, -0.002952755905511810983, -0.1113553986120547346 ) ) ;
#38593=( BOUNDED_CURVE ( )  B_SPLINE_CURVE ( 2, ( #18857, #14574, #18626, #26325, #29247, #37305, #10994, #18400, #43795 ),
 .UNSPECIFIED., .F., .T. ) 
 B_SPLINE_CURVE_WITH_KNOTS ( ( 3, 2, 2, 2, 3 ),
 ( 0.02500000000000000139, 0.02750000000000000014, 0.02999999999999999889, 0.03250000000000000111, 0.03500000000000000333 ),
 .UNSPECIFIED. ) 
 CURVE ( )  GEOMETRIC_REPRESENTATION_ITEM ( )  RATIONAL_B_SPLINE_CURVE ( ( 1.000000000000000000, 0.9238795325112869605, 1.000000000000000000, 0.9238795325112869605, 1.000000000000000000, 0.9238795325112869605, 1.000000000000000000, 0.9238795325112869605, 1.000000000000000000 ) ) 
 REPRESENTATION_ITEM ( '' )  ) ;
#38597=CARTESIAN_POINT ( 'NONE',  ( 0.1113553986120547346, -0.9773622046168818356, -0.1113553986120547346 ) ) ;
#38598=CARTESIAN_POINT ( 'NONE',  ( 0.1264236179284866091, -0.4138779527021417826, -0.1264236179284866091 ) ) ;
#38600=CARTESIAN_POINT ( 'NONE',  ( -0.1787899950787401604, -1.375984251914741163, 0.07405724077823318263 ) ) ;
#38606=CARTESIAN_POINT ( 'NONE',  ( 0.1113553986120547346, -1.252952755797984041, -0.1113553986120547346 ) ) ;
#38610=CARTESIAN_POINT ( 'NONE',  ( 0.1623548122380495395, -0.09842494649416595742, -0.07493597120910913678 ) ) ;
#38613=DIRECTION ( 'NONE',  ( 0.000000000000000000, 1.000000000000000000, 0.000000000000000000 ) ) ;
#38620=CARTESIAN_POINT ( 'NONE',  ( 0.02849075975873720593, -0.09851384916348070175, 0.2212810442481748241 ) ) ;
#38628=CARTESIAN_POINT ( 'NONE',  ( -0.1787899950787401882, -1.591167275315852558, 0.000000000000000000 ) ) ;
#38631=CARTESIAN_POINT ( 'NONE',  ( 0.1787899950787401604, -0.5295275590013543976, -0.07405724077823318263 ) ) ;
#38638=CARTESIAN_POINT ( 'NONE',  ( -0.07405724077823318263, -0.3277559054580475584, -0.1787899950787401604 ) ) ;
#38639=CARTESIAN_POINT ( 'NONE',  ( -0.1787899950787401604, -0.7116141731745821986, -0.07405724077823318263 ) ) ;
#38643=CARTESIAN_POINT ( 'NONE',  ( -0.1787899950787401604, 0.05991540184950147618, -0.07405724077823318263 ) ) ;
#38648=CARTESIAN_POINT ( 'NONE',  ( -0.1574803149606300301, -0.8567913385826780859, -0.06523048226347956391 ) ) ;
#38650=CARTESIAN_POINT ( 'NONE',  ( -0.07444174185955065859, -1.543843022181471847, -0.1797182628040039087 ) ) ;
#38654=CARTESIAN_POINT ( 'NONE',  ( -0.1787899950787401604, -0.3572834645131658382, -0.07405724077823318263 ) ) ;
#38657=CARTESIAN_POINT ( 'NONE',  ( 0.1572451146043649106, 0.09317026862874189241, -0.1946475616205581294 ) ) ;
#38664=CARTESIAN_POINT ( 'NONE',  ( -0.1574803149606297803, -0.8813976376877487029, 0.06523048226347956391 ) ) ;
#38665=CARTESIAN_POINT ( 'NONE',  ( 0.1787899950787401882, -0.02509842514308689362, -2.189545951927503898E-17 ) ) ;
#38667=CARTESIAN_POINT ( 'NONE',  ( -1.094772975963752103E-17, -0.04970472435568527164, -0.1787899950787401882 ) ) ;
#38669=CARTESIAN_POINT ( 'NONE',  ( 0.1264236179284866091, -0.9306102361667086820, 0.1264236179284866091 ) ) ;
#38676=DIRECTION ( 'NONE',  ( 0.000000000000000000, 0.000000000000000000, 1.000000000000000000 ) ) ;
#38679=CARTESIAN_POINT ( 'NONE',  ( -0.1787899950787401604, -1.302165354276944242, 0.07405724077823318263 ) ) ;
#38686=DIRECTION ( 'NONE',  ( 0.000000000000000000, 0.000000000000000000, 1.000000000000000000 ) ) ;
#38690=ORIENTED_EDGE ( 'NONE', *, *, #19690, .F. ) ;
#38697=CARTESIAN_POINT ( 'NONE',  ( -0.2471922904502826257, 0.09379707428445145656, -0.03645092102368886755 ) ) ;
#38699=CARTESIAN_POINT ( 'NONE',  ( 0.1787899950787401604, -1.135950739882782834, -0.07405724077823318263 ) ) ;
#38701=CARTESIAN_POINT ( 'NONE',  ( 0.07405724077823318263, -0.1062992125446616531, 0.1787899950787401604 ) ) ;
#38709=CARTESIAN_POINT ( 'NONE',  ( 0.1264236179284866091, -0.6599409448281259305, 0.1264236179284866091 ) ) ;
#38713=CARTESIAN_POINT ( 'NONE',  ( -0.1270800023317771588, -1.098469006433439032, 0.1270800023317771588 ) ) ;
#38717=CARTESIAN_POINT ( 'NONE',  ( 0.000000000000000000, -0.09842519685039370636, 0.000000000000000000 ) ) ;
#38729=CARTESIAN_POINT ( 'NONE',  ( 0.1113553986120547346, -1.656496062884598386, 0.1113553986120547346 ) ) ;
#38735=CARTESIAN_POINT ( 'NONE',  ( -0.1574803149606299191, -1.759842519685039353, 0.000000000000000000 ) ) ;
#38744=CARTESIAN_POINT ( 'NONE',  ( 0.1574803149606300301, -0.3941929132782996947, 0.06523048226347956391 ) ) ;
#38745=CARTESIAN_POINT ( 'NONE',  ( -0.07405724077823318263, -1.745078740103716886, -0.1787899950787401604 ) ) ;
#38754=CARTESIAN_POINT ( 'NONE',  ( 0.1577181258794738139, -0.08956002199932618091, 0.1424585403325043520 ) ) ;
#38757=CARTESIAN_POINT ( 'NONE',  ( -0.02739131347899105909, -0.09752745740044843625, 0.1550798682808147422 ) ) ;
#38766=CARTESIAN_POINT ( 'NONE',  ( 0.1797182628040039365, -0.7687445969846200544, -2.200913952912460540E-17 ) ) ;
#38769=CARTESIAN_POINT ( 'NONE',  ( -0.1574803149606297803, -0.4581692913385826404, 0.06523048226347956391 ) ) ;
#38770=CARTESIAN_POINT ( 'NONE',  ( -0.1738374315028377304, -0.09842519685039370636, 0.01279107473069981266 ) ) ;
#38773=CARTESIAN_POINT ( 'NONE',  ( 0.1574803149606300301, 0.02903543307086614220, 0.06523048226347956391 ) ) ;
#38782=CARTESIAN_POINT ( 'NONE',  ( -0.1688295671091639694, -0.08956462757123960505, -0.02832533445597745780 ) ) ;
#38783=CARTESIAN_POINT ( 'NONE',  ( -0.1787899950787401604, -0.5492125983714331028, 0.07405724077823318263 ) ) ;
#38788=CARTESIAN_POINT ( 'NONE',  ( -0.01993724539793482325, 0.05212746764698077823, -0.2739222968687445303 ) ) ;
#38790=CARTESIAN_POINT ( 'NONE',  ( 0.07444174185955046430, 0.06540894632246617435, -0.1797182628040039087 ) ) ;
#38791=CARTESIAN_POINT ( 'NONE',  ( -0.1787899950787401604, -1.026574803095842370, 0.07405724077823318263 ) ) ;
#38792=CARTESIAN_POINT ( 'NONE',  ( -0.1574803149606299191, -1.366141732283464583, 0.000000000000000000 ) ) ;
#38797=ORIENTED_EDGE ( 'NONE', *, *, #5852, .F. ) ;
#38798=CARTESIAN_POINT ( 'NONE',  ( -0.1574803149606300301, -1.437499999892472013, -0.06523048226347956391 ) ) ;
#38810=CARTESIAN_POINT ( 'NONE',  ( 0.2074171527642326707, -0.09842519685039548272, 0.02027778249552708578 ) ) ;
#38811=CARTESIAN_POINT ( 'NONE',  ( -0.06523048226347956391, 0.01919291338582680001, 0.1574803149606297803 ) ) ;
#38817=CARTESIAN_POINT ( 'NONE',  ( 3.284318927891251994E-17, -1.019192913332062966, 0.1787899950787401882 ) ) ;
#38818=CARTESIAN_POINT ( 'NONE',  ( 0.1264236179284866091, -1.235728346402928945, -0.1264236179284866091 ) ) ;
#38820=CARTESIAN_POINT ( 'NONE',  ( -0.1270800023317771588, -0.5472879040712346210, 0.1270800023317771588 ) ) ;
#38823=CARTESIAN_POINT ( 'NONE',  ( 0.1113553986120547346, -0.04232283464566929249, -0.1113553986120547346 ) ) ;
#38832=CARTESIAN_POINT ( 'NONE',  ( 0.1787899950787401604, -0.6525590550643474153, -0.07405724077823318263 ) ) ;
#38833=CARTESIAN_POINT ( 'NONE',  ( -1.094772975963752103E-17, -1.467027559001354398, -0.1787899950787401882 ) ) ;
#38837=EDGE_CURVE ( 'NONE', #36464, #28863, #43706, .T. ) ;
#38839=DIRECTION ( 'NONE',  ( 0.000000000000000000, 1.000000000000000000, 0.000000000000000000 ) ) ;
#38841=CARTESIAN_POINT ( 'NONE',  ( 0.1391909071597861591, -0.09842519806770759494, -0.1123953384983699400 ) ) ;
#38844=CARTESIAN_POINT ( 'NONE',  ( 0.1628039705523879055, -0.09131796649104584329, 0.1914378685689082094 ) ) ;
#38852=CARTESIAN_POINT ( 'NONE',  ( 0.2058001524074047073, -0.09851384666201024043, -0.01602185461346814985 ) ) ;
#38859=CARTESIAN_POINT ( 'NONE',  ( 0.1264236179284866091, -0.6451771653005667906, -0.1264236179284866091 ) ) ;
#38865=CARTESIAN_POINT ( 'NONE',  ( -0.07405724077823318263, -0.7165354330171036512, -0.1787899950787401604 ) ) ;
#38866=CARTESIAN_POINT ( 'NONE',  ( -0.2471922904502826812, -0.09842519685039370636, 5.914624404477007554E-17 ) ) ;
#38868=CARTESIAN_POINT ( 'NONE',  ( -0.1787899950787401604, 0.02054532310934393743, -0.07405724077823318263 ) ) ;
#38869=CARTESIAN_POINT ( 'NONE',  ( -0.1787899950787401882, 0.03395669296714932950, 0.000000000000000000 ) ) ;
#38874=CARTESIAN_POINT ( 'NONE',  ( 0.1574803149606300301, -0.9109251968503938590, -0.06523048226347956391 ) ) ;
#38876=CARTESIAN_POINT ( 'NONE',  ( -0.1797182628040039087, -1.534000502496431606, 0.07444174185955065859 ) ) ;
#38878=CARTESIAN_POINT ( 'NONE',  ( 3.284318927891251994E-17, -0.3449803149068665364, 0.1787899950787401882 ) ) ;
#38884=CARTESIAN_POINT ( 'NONE',  ( -0.1628039705528179781, -0.09131796649085367756, -0.1914378685686898007 ) ) ;
#38889=CARTESIAN_POINT ( 'NONE',  ( -0.06523048226347956391, -0.8764763778452294707, 0.1574803149606297803 ) ) ;
#38890=CARTESIAN_POINT ( 'NONE',  ( 0.1787899950787401604, -0.1013779527021420185, -0.07405724077823318263 ) ) ;
#38892=CARTESIAN_POINT ( 'NONE',  ( 3.284318927891251994E-17, -0.9749015747493857686, 0.1787899950787401882 ) ) ;
#38901=CARTESIAN_POINT ( 'NONE',  ( 0.07405724077823318263, -1.356299212544662014, -0.1787899950787401604 ) ) ;
#38907=DIRECTION ( 'NONE',  ( -0.000000000000000000, -1.000000000000000000, -0.000000000000000000 ) ) ;
#38917=CARTESIAN_POINT ( 'NONE',  ( -0.1787899950787401604, -1.076895621772545830, 0.07405724077823318263 ) ) ;
#38919=CARTESIAN_POINT ( 'NONE',  ( 0.07405724077823318263, -0.1456692912848192578, 0.1787899950787401604 ) ) ;
#38924=AXIS2_PLACEMENT_3D ( 'NONE', #612, #18843, #15043 ) ;
#38927=CARTESIAN_POINT ( 'NONE',  ( -0.1797182628040039087, -0.2397091639137541308, -0.07444174185955065859 ) ) ;
#38928=CARTESIAN_POINT ( 'NONE',  ( 0.1787899950787401604, -0.7755905511273385455, 0.07405724077823318263 ) ) ;
#38931=CARTESIAN_POINT ( 'NONE',  ( 0.07444174185955046430, -1.233803652102731352, -0.1797182628040039087 ) ) ;
#38941=CARTESIAN_POINT ( 'NONE',  ( -0.1787899950787401604, -0.002952755851748307785, -0.07405724077823318263 ) ) ;
#38955=CARTESIAN_POINT ( 'NONE',  ( -0.1787899950787401604, -0.08169291333206318839, -0.07405724077823318263 ) ) ;
#38962=CARTESIAN_POINT ( 'NONE',  ( 0.07405724077823318263, -1.725393700733637958, 0.1787899950787401604 ) ) ;
#38971=CARTESIAN_POINT ( 'NONE',  ( -0.009204872250209487905, -0.08956057363312637520, -0.1860142604523574716 ) ) ;
#38986=CARTESIAN_POINT ( 'NONE',  ( 0.1270800023317771588, -0.6555556206066672775, 0.1270800023317771588 ) ) ;
#38989=CARTESIAN_POINT ( 'NONE',  ( 0.06523048226347956391, -0.5270669291338577755, 0.1574803149606297803 ) ) ;
#38995=CARTESIAN_POINT ( 'NONE',  ( 0.1113553986120547346, 0.07578740168233012720, 0.1113553986120547346 ) ) ;
#39011=ORIENTED_EDGE ( 'NONE', *, *, #25927, .T. ) ;
#39014=CARTESIAN_POINT ( 'NONE',  ( 0.1797182628040039365, 0.1367672140390017721, -2.200913952912460540E-17 ) ) ;
#39015=CARTESIAN_POINT ( 'NONE',  ( 0.07405724077823318263, -1.080708661363559919, -0.1787899950787401604 ) ) ;
#39016=CARTESIAN_POINT ( 'NONE',  ( 0.1113553986120547346, -1.390748031496063186, 0.1113553986120547346 ) ) ;
#39026=CARTESIAN_POINT ( 'NONE',  ( -0.2471922904502826535, 0.09142184925109154980, 0.04493454898959751281 ) ) ;
#39030=CARTESIAN_POINT ( 'NONE',  ( -0.1787899950787401604, -0.2550452280717585563, -0.07405724077823318263 ) ) ;
#39031=CARTESIAN_POINT ( 'NONE',  ( 0.05862610683640598341, -0.09842519685039370636, 0.2134590741261405689 ) ) ;
#39038=CARTESIAN_POINT ( 'NONE',  ( -0.07405724077823318263, -1.100393700733639069, 0.1787899950787401604 ) ) ;
#39039=CARTESIAN_POINT ( 'NONE',  ( -0.1264236179284866091, -1.216043307032850462, 0.1264236179284866091 ) ) ;
#39042=CARTESIAN_POINT ( 'NONE',  ( 0.1270800023317771588, -0.5374453843861952684, 0.1270800023317771588 ) ) ;
#39046=CARTESIAN_POINT ( 'NONE',  ( -0.1574803149606297803, -0.02509842519685037687, 0.06523048226347956391 ) ) ;
#39048=CARTESIAN_POINT ( 'NONE',  ( 2.892866454678787531E-17, -0.05708661417322834220, 0.1574803149606299191 ) ) ;
#39054=CIRCLE ( 'NONE', #6146, 0.2204724409448818867 ) ;
#39058=CARTESIAN_POINT ( 'NONE',  ( -0.1787899950787401882, -0.5172244093950552069, 0.000000000000000000 ) ) ;
#39060=CARTESIAN_POINT ( 'NONE',  ( -1.094772975963752103E-17, -1.388287401521039355, -0.1787899950787401882 ) ) ;
#39077=CARTESIAN_POINT ( 'NONE',  ( -0.02315057879874008254, -0.09851384983704390697, 0.2241609000832641696 ) ) ;
#39081=CARTESIAN_POINT ( 'NONE',  ( -0.1787899950787401882, -1.630537354056009969, 0.000000000000000000 ) ) ;
#39083=CARTESIAN_POINT ( 'NONE',  ( 0.07405724077823318263, -0.6033464566391496531, -0.1787899950787401604 ) ) ;
#39089=CARTESIAN_POINT ( 'NONE',  ( 0.1787899950787401604, -0.3375984251430867999, -0.07405724077823318263 ) ) ;
#39090=CARTESIAN_POINT ( 'NONE',  ( -0.07405724077823318263, -0.7952755904974174728, -0.1787899950787401604 ) ) ;
#39092=CARTESIAN_POINT ( 'NONE',  ( 0.000000000000000000, -0.09842519685039370636, 0.000000000000000000 ) ) ;
#39095=CARTESIAN_POINT ( 'NONE',  ( 0.1264236179284866091, -0.03112790523711275736, -0.1264236179284866091 ) ) ;
#39096=CARTESIAN_POINT ( 'NONE',  ( 0.07405724077823318263, 0.1003937008411650705, -0.1787899950787401604 ) ) ;
#39101=CARTESIAN_POINT ( 'NONE',  ( 0.1574803149606300301, -0.9552165354330708347, 0.06523048226347956391 ) ) ;
#39103=CARTESIAN_POINT ( 'NONE',  ( 3.301370929368692659E-17, -1.762839085173596443, 0.1797182628040039365 ) ) ;
#39105=CARTESIAN_POINT ( 'NONE',  ( -0.1264236179284866091, -0.3499015747493862127, 0.1264236179284866091 ) ) ;
#39115=CARTESIAN_POINT ( 'NONE',  ( -0.1264236179284866091, -0.07923228341080333637, 0.1264236179284866091 ) ) ;
#39117=CARTESIAN_POINT ( 'NONE',  ( 0.07405724077823318263, -0.9970472440407247561, -0.1787899950787401604 ) ) ;
#39118=DIRECTION ( 'NONE',  ( 0.000000000000000000, 0.000000000000000000, 1.000000000000000000 ) ) ;
#39146=CARTESIAN_POINT ( 'NONE',  ( 0.1264236179284866091, -1.103962550906403495, 0.1264236179284866091 ) ) ;
#39148=CARTESIAN_POINT ( 'NONE',  ( 0.1264236179284866091, -0.05462598419820496182, -0.1264236179284866091 ) ) ;
#39158=EDGE_CURVE ( 'NONE', #35410, #35946, #13521, .T. ) ;
#39159=CARTESIAN_POINT ( 'NONE',  ( 0.07405724077823318263, -0.7263779527021420046, -0.1787899950787401604 ) ) ;
#39184=CARTESIAN_POINT ( 'NONE',  ( 0.1264236179284866091, -0.01525590545804753929, -0.1264236179284866091 ) ) ;
#39191=CARTESIAN_POINT ( 'NONE',  ( 0.07405724077823318263, -1.686023621993479882, 0.1787899950787401604 ) ) ;
#39200=CARTESIAN_POINT ( 'NONE',  ( 0.1264236179284866091, -0.6610491650796320728, -0.1264236179284866091 ) ) ;
#39202=CARTESIAN_POINT ( 'NONE',  ( -0.1663756747267724490, -0.08956132504751300460, 0.02463664667560858459 ) ) ;
#39208=CARTESIAN_POINT ( 'NONE',  ( 0.1113553986120547346, -0.002952755905511810983, -0.1113553986120547346 ) ) ;
#39219=CARTESIAN_POINT ( 'NONE',  ( 0.07444174185955065859, -0.7761264867484009011, 0.1797182628040039087 ) ) ;
#39220=CARTESIAN_POINT ( 'NONE',  ( 0.2471922904502826812, 0.07821434602336012343, 0.07684457919973788909 ) ) ;
#39223=CARTESIAN_POINT ( 'NONE',  ( -0.06523048226347956391, -0.6500984251968493499, 0.1574803149606297803 ) ) ;
#39237=CARTESIAN_POINT ( 'NONE',  ( 0.09009865225413171697, 0.1299212598425196763, 0.1562008126607098424 ) ) ;
#39241=CARTESIAN_POINT ( 'NONE',  ( 0.07444174185955065859, 0.09001524553506463910, 0.1797182628040039087 ) ) ;
#39242=CARTESIAN_POINT ( 'NONE',  ( 0.1264236179284866091, -1.004429133804503937, -0.1264236179284866091 ) ) ;
#39243=CARTESIAN_POINT ( 'NONE',  ( 2.892866454678787531E-17, -1.474409448818897461, 0.1574803149606299191 ) ) ;
#39257=CARTESIAN_POINT ( 'NONE',  ( -0.1350291203833209053, 0.09842519685039377575, -0.2074739718643930364 ) ) ;
#39261=CARTESIAN_POINT ( 'NONE',  ( 0.1264236179284866091, -0.3165609761032547875, 0.1264236179284866091 ) ) ;
#39269=VERTEX_POINT ( 'NONE', #16643 ) ;
#39272=CARTESIAN_POINT ( 'NONE',  ( 0.1264236179284866091, -1.122539370024976391, -0.1264236179284866091 ) ) ;
#39273=CARTESIAN_POINT ( 'NONE',  ( -0.1264236179284866091, -1.186515747977732183, -0.1264236179284866091 ) ) ;
#39274=DIRECTION ( 'NONE',  ( 0.000000000000000000, 1.000000000000000000, 0.000000000000000000 ) ) ;
#39275=CARTESIAN_POINT ( 'NONE',  ( 0.1797182628040039365, -0.5718942032838330025, -2.200913952912460540E-17 ) ) ;
#39279=CARTESIAN_POINT ( 'NONE',  ( 0.1574803149606300301, -0.1628937007874015908, -0.06523048226347956391 ) ) ;
#39293=CARTESIAN_POINT ( 'NONE',  ( -0.1264236179284866091, -0.5516732282926929409, 0.1264236179284866091 ) ) ;
#39294=CARTESIAN_POINT ( 'NONE',  ( 0.1113553986120547346, -1.105314960629921295, -0.1113553986120547346 ) ) ;
#39300=CARTESIAN_POINT ( 'NONE',  ( -0.1113553986120547346, -1.272637795168062746, 0.1113553986120547346 ) ) ;
#39309=CARTESIAN_POINT ( 'NONE',  ( -0.06523048226347956391, -0.2613188975302682127, -0.1574803149606300301 ) ) ;
#39315=CARTESIAN_POINT ( 'NONE',  ( 0.07328326258864251153, -0.09851384743134017352, 0.2080889956503677307 ) ) ;
#39316=EDGE_LOOP ( 'NONE', ( #44527, #36619, #37826 ) ) ;
#39318=EDGE_CURVE ( 'NONE', #4638, #19219, #5048, .T. ) ;
#39320=CARTESIAN_POINT ( 'NONE',  ( -0.1787899950787401604, -0.5935039369541101895, -0.07405724077823318263 ) ) ;
#39326=CARTESIAN_POINT ( 'NONE',  ( 0.1787899950787401882, -0.3006889763241893943, -2.189545951927503898E-17 ) ) ;
#39327=CARTESIAN_POINT ( 'NONE',  ( 0.1787899950787401882, -0.7682086613635590311, -2.189545951927503898E-17 ) ) ;
#39328=CARTESIAN_POINT ( 'NONE',  ( -0.2471908670705637023, -0.09572725253288329184, -0.02814577918614243404 ) ) ;
#39330=CARTESIAN_POINT ( 'NONE',  ( 0.07405724077823318263, -0.04343105484341201056, 0.1787899950787401604 ) ) ;
#39331=CARTESIAN_POINT ( 'NONE',  ( 0.1088466229509682248, -0.09842519685039366473, 0.1288475576157622204 ) ) ;
#39336=CARTESIAN_POINT ( 'NONE',  ( 2.892866454678787531E-17, -0.9232283464566929387, 0.1574803149606299191 ) ) ;
#39338=CARTESIAN_POINT ( 'NONE',  ( -0.1270800023317771588, -1.689020187535801076, 0.1270800023317771588 ) ) ;
#39344=CARTESIAN_POINT ( 'NONE',  ( -0.1607876024859741237, -0.09201407021827166799, -0.1926022046197118087 ) ) ;
#39347=CARTESIAN_POINT ( 'NONE',  ( -0.1787899950787401882, -0.1235236219934805202, 0.000000000000000000 ) ) ;
#39350=CARTESIAN_POINT ( 'NONE',  ( 0.1787899950787401882, -0.9650590550643465271, -2.189545951927503898E-17 ) ) ;
#39371=CARTESIAN_POINT ( 'NONE',  ( 0.1787899950787401882, 0.01427165359707061217, -2.189545951927503898E-17 ) ) ;
#39378=CARTESIAN_POINT ( 'NONE',  ( 0.1264236179284866091, -1.290970424922151638, -0.1264236179284866091 ) ) ;
#39380=CARTESIAN_POINT ( 'NONE',  ( 0.1787899950787401604, -0.1358267715997797664, -0.07405724077823318263 ) ) ;
#39388=CARTESIAN_POINT ( 'NONE',  ( 3.284318927891251994E-17, -1.452263779473795369, 0.1787899950787401882 ) ) ;
#39400=CARTESIAN_POINT ( 'NONE',  ( 0.06523048226347956391, -0.7928149605223941965, 0.1574803149606297803 ) ) ;
#39419=CARTESIAN_POINT ( 'NONE',  ( -0.1787899950787401882, 0.03887795280966901967, 0.000000000000000000 ) ) ;
#39426=CARTESIAN_POINT ( 'NONE',  ( 0.1850060400416835837, 0.08128102204193912717, 0.1786197838463692011 ) ) ;
#39431=CARTESIAN_POINT ( 'NONE',  ( -0.07405724077823318263, -1.666338582623402953, -0.1787899950787401604 ) ) ;
#39440=CARTESIAN_POINT ( 'NONE',  ( -0.1787899950787401604, -0.6881160942134909586, -0.07405724077823318263 ) ) ;
#39447=CARTESIAN_POINT ( 'NONE',  ( 0.06523048226347956391, 0.07824803149606308905, -0.1574803149606300301 ) ) ;
#39455=CARTESIAN_POINT ( 'NONE',  ( 0.07444174185955065859, -0.8942367229688730212, 0.1797182628040039087 ) ) ;
#39459=CARTESIAN_POINT ( 'NONE',  ( -0.1574803149606299191, -0.6181102362204724532, 0.000000000000000000 ) ) ;
#39478=CARTESIAN_POINT ( 'NONE',  ( -0.1797182628040039087, 0.1539916234878207224, -0.07444174185955065859 ) ) ;
#39479=CARTESIAN_POINT ( 'NONE',  ( 0.07405724077823318263, -1.056102362150961982, 0.1787899950787401604 ) ) ;
#39480=CARTESIAN_POINT ( 'NONE',  ( 0.1574803149606300301, -1.467027559055119168, 0.06523048226347956391 ) ) ;
#39481=ADVANCED_FACE ( 'NONE', ( #40971 ), #11425, .T. ) ;
#39487=CARTESIAN_POINT ( 'NONE',  ( 0.06523048226347956391, -1.447342519577512476, -0.1574803149606300301 ) ) ;
#39498=CARTESIAN_POINT ( 'NONE',  ( 3.284318927891251994E-17, -0.2427420784654590602, 0.1787899950787401882 ) ) ;
#39499=CARTESIAN_POINT ( 'NONE',  ( -0.1150168755148803235, -0.09842519685039370636, 0.1175860779051826899 ) ) ;
#39506=CARTESIAN_POINT ( 'NONE',  ( -0.1787899950787401882, -1.186515747977732183, 0.000000000000000000 ) ) ;
#39507=CARTESIAN_POINT ( 'NONE',  ( -0.07405724077823318263, -1.385826771599779184, -0.1787899950787401604 ) ) ;
#39509=( NAMED_UNIT ( * ) PLANE_ANGLE_UNIT ( ) SI_UNIT ( $, .RADIAN. ) ) ;
#39510=CARTESIAN_POINT ( 'NONE',  ( 0.1797182628040039087, -0.6088036521027303527, -0.07444174185955065859 ) ) ;
#39514=CARTESIAN_POINT ( 'NONE',  ( -9.642888182262618425E-18, -0.1555118110236220763, -0.1574803149606299191 ) ) ;
#39528=CARTESIAN_POINT ( 'NONE',  ( 0.06523048226347956391, -1.540846456585386548, 0.1574803149606297803 ) ) ;
#39529=CARTESIAN_POINT ( 'NONE',  ( -0.07405724077823318263, -0.5885826771115909573, 0.1787899950787401604 ) ) ;
#39530=CARTESIAN_POINT ( 'NONE',  ( 0.06523048226347956391, -0.9847440944881884484, -0.1574803149606300301 ) ) ;
#39539=ADVANCED_FACE ( 'NONE', ( #37173, #37401 ), #26173, .T. ) ;
#39548=CARTESIAN_POINT ( 'NONE',  ( 0.1910692666444111232, -0.07766248740297354569, 0.1751191768260063897 ) ) ;
#39550=CARTESIAN_POINT ( 'NONE',  ( 0.06523048226347956391, -0.2416338581601896740, 0.1574803149606297803 ) ) ;
#39555=CARTESIAN_POINT ( 'NONE',  ( 0.1312513784215866286, -0.09851384505487205401, -0.1483491369261773773 ) ) ;
#39562=CARTESIAN_POINT ( 'NONE',  ( -0.07405724077823318263, -0.3523622046706461619, 0.1787899950787401604 ) ) ;
#39563=CARTESIAN_POINT ( 'NONE',  ( 3.284318927891251994E-17, -0.9355314960092283583, 0.1787899950787401882 ) ) ;
#39565=FACE_OUTER_BOUND ( 'NONE', #26156, .T. ) ;
#39567=CARTESIAN_POINT ( 'NONE',  ( 0.1264236179284866091, -0.08034050366230964524, 0.1264236179284866091 ) ) ;
#39568=CARTESIAN_POINT ( 'NONE',  ( -0.1787899950787401604, -0.2736220471903310081, 0.07405724077823318263 ) ) ;
#39569=CARTESIAN_POINT ( 'NONE',  ( 0.07405724077823318263, 0.02165354336085014916, -0.1787899950787401604 ) ) ;
#39575=CARTESIAN_POINT ( 'NONE',  ( -0.07444174185955065859, -1.780063494622415865, -0.1797182628040039087 ) ) ;
#39576=CARTESIAN_POINT ( 'NONE',  ( -1.094772975963752103E-17, -0.4434055117572598959, -0.1787899950787401882 ) ) ;
#39583=CARTESIAN_POINT ( 'NONE',  ( -0.1986060025687029773, -0.07294156354251685181, -0.1707667409195914865 ) ) ;
#39586=CARTESIAN_POINT ( 'NONE',  ( -0.1264236179284866091, -0.08907480309584270284, -0.1264236179284866091 ) ) ;
#39588=CARTESIAN_POINT ( 'NONE',  ( -0.1787899950787401882, -1.142224409395055096, 0.000000000000000000 ) ) ;
#39590=EDGE_CURVE ( 'NONE', #26985, #3096, #16557, .T. ) ;
#39610=CARTESIAN_POINT ( 'NONE',  ( 0.1787899950787401882, -0.02509842514308689362, -2.189545951927503898E-17 ) ) ;
#39616=CARTESIAN_POINT ( 'NONE',  ( 0.07405724077823318263, -1.342643653268609460, 0.1787899950787401604 ) ) ;
#39618=CARTESIAN_POINT ( 'NONE',  ( 0.07405724077823318263, -0.2883858267178899260, -0.1787899950787401604 ) ) ;
#39624=CARTESIAN_POINT ( 'NONE',  ( 0.1264236179284866091, -1.594980314906866203, -0.1264236179284866091 ) ) ;
#39649=CARTESIAN_POINT ( 'NONE',  ( -0.1264236179284866091, -0.08415354325332302654, -0.1264236179284866091 ) ) ;
#39656=CARTESIAN_POINT ( 'NONE',  ( -0.1574803149606299191, 0.1397637796350860440, 0.000000000000000000 ) ) ;
#39664=CARTESIAN_POINT ( 'NONE',  ( -1.094772975963752103E-17, -0.8136082201977422601, -0.1787899950787401882 ) ) ;
#39667=CARTESIAN_POINT ( 'NONE',  ( 0.1264236179284866091, 0.1323818898175431191, 0.1264236179284866091 ) ) ;
#39679=CARTESIAN_POINT ( 'NONE',  ( -1.100456976456230270E-17, -0.7982721560397381122, -0.1797182628040039365 ) ) ;
#39684=CARTESIAN_POINT ( 'NONE',  ( -0.06523048226347956391, -0.5467519685039372579, -0.1574803149606300301 ) ) ;
#39691=CARTESIAN_POINT ( 'NONE',  ( 0.06523048226347956391, -0.6205708660342047489, -0.1574803149606300301 ) ) ;
#39697=DIRECTION ( 'NONE',  ( 0.000000000000000000, -1.000000000000000000, 0.000000000000000000 ) ) ;
#39701=CARTESIAN_POINT ( 'NONE',  ( -0.07444174185955065859, 0.08509398569254496281, 0.1797182628040039087 ) ) ;
#39702=CARTESIAN_POINT ( 'NONE',  ( -0.07405724077823318263, -1.179133858213953001, 0.1787899950787401604 ) ) ;
#39703=CARTESIAN_POINT ( 'NONE',  ( 0.06523048226347956391, -1.590059055118110187, 0.1574803149606297803 ) ) ;
#39721=CARTESIAN_POINT ( 'NONE',  ( -0.07405724077823318263, -0.4568168816150654510, -0.1787899950787401604 ) ) ;
#39722=CARTESIAN_POINT ( 'NONE',  ( -0.1264082094504824783, -0.09842519685039370636, 0.1067823974213112231 ) ) ;
#39732=CARTESIAN_POINT ( 'NONE',  ( -0.07405724077823318263, -1.218503936954111300, 0.1787899950787401604 ) ) ;
#39733=CARTESIAN_POINT ( 'NONE',  ( -0.1787899950787401604, -1.415354330654897019, 0.07405724077823318263 ) ) ;
#39741=CARTESIAN_POINT ( 'NONE',  ( 0.1574803149606300301, -0.1678149606299212671, 0.06523048226347956391 ) ) ;
#39751=CARTESIAN_POINT ( 'NONE',  ( -0.07405724077823318263, -0.07185039364702389131, 0.1787899950787401604 ) ) ;
#39753=CARTESIAN_POINT ( 'NONE',  ( 0.1113553986120547346, -1.528543306979086358, -0.1113553986120547346 ) ) ;
#39754=CARTESIAN_POINT ( 'NONE',  ( 3.284318927891251994E-17, -0.7436023621509606496, 0.1787899950787401882 ) ) ;
#39755=CARTESIAN_POINT ( 'NONE',  ( -0.06523048226347956391, -1.083169291338583529, 0.1574803149606297803 ) ) ;
#39765=CARTESIAN_POINT ( 'NONE',  ( 0.1574803149606300301, -1.260334645561765221, 0.06523048226347956391 ) ) ;
#39774=CARTESIAN_POINT ( 'NONE',  ( 0.06523048226347956391, -0.1628937006798744369, 0.1574803149606297803 ) ) ;
#39779=CARTESIAN_POINT ( 'NONE',  ( -0.08758009603785964214, -0.09851383865516692706, -0.1629933310116103984 ) ) ;
#39782=CARTESIAN_POINT ( 'NONE',  ( -0.07405724077823318263, -1.677289322559946116, -0.1787899950787401604 ) ) ;
#39788=CARTESIAN_POINT ( 'NONE',  ( 0.1787899950787401882, -0.8863188975840314843, -2.189545951927503898E-17 ) ) ;
#39790=CARTESIAN_POINT ( 'NONE',  ( -0.2471922899045395083, -0.07845124750587918749, -0.07638293795139619591 ) ) ;
#39794=CARTESIAN_POINT ( 'NONE',  ( -0.07444174185955065859, -0.2052603450161165910, -0.1797182628040039087 ) ) ;
#39796=CARTESIAN_POINT ( 'NONE',  ( -0.1264236179284866091, -0.1000255430323883782, -0.1264236179284866091 ) ) ;
#39797=CARTESIAN_POINT ( 'NONE',  ( -0.1264236179284866091, 0.06840551186478720236, -0.1264236179284866091 ) ) ;
#39798=CARTESIAN_POINT ( 'NONE',  ( 0.2471922026429001218, -0.09209855619650188230, -0.04265916557990739183 ) ) ;
#39806=CARTESIAN_POINT ( 'NONE',  ( 0.07444174185955046430, -1.706244596984621387, -0.1797182628040039087 ) ) ;
#39809=CARTESIAN_POINT ( 'NONE',  ( -0.1572356565282391760, -0.09317336072449060314, 0.1946530291195329998 ) ) ;
#39814=CARTESIAN_POINT ( 'NONE',  ( -0.07405724077823318263, -0.1555118109698585271, 0.1787899950787401604 ) ) ;
#39817=CARTESIAN_POINT ( 'NONE',  ( -0.07405724077823318263, -1.070866141678519456, -0.1787899950787401604 ) ) ;
#39827=CARTESIAN_POINT ( 'NONE',  ( 0.000000000000000000, -0.09842519685039370636, 0.1574803149606299191 ) ) ;
#39840=CARTESIAN_POINT ( 'NONE',  ( -0.07405724077823318263, 0.001968503990771401039, 0.1787899950787401604 ) ) ;
#39849=CARTESIAN_POINT ( 'NONE',  ( -0.07405724077823318263, -1.322958613898530533, -0.1787899950787401604 ) ) ;
#39851=CARTESIAN_POINT ( 'NONE',  ( 0.1787899950787401604, -0.2539370078202523584, -0.07405724077823318263 ) ) ;
#39855=CARTESIAN_POINT ( 'NONE',  ( -0.2471886260750748299, -0.05069887331258201429, 0.1203475566276436537 ) ) ;
#39858=CARTESIAN_POINT ( 'NONE',  ( 0.07405724077823318263, -1.567913385773008095, 0.1787899950787401604 ) ) ;
#39859=CARTESIAN_POINT ( 'NONE',  ( 0.07405724077823318263, -0.7411417322297018107, 0.1787899950787401604 ) ) ;
#39863=CARTESIAN_POINT ( 'NONE',  ( 0.1797182628040039087, -1.283016250527927893, 0.07444174185955046430 ) ) ;
#39875=CARTESIAN_POINT ( 'NONE',  ( -0.1787899950787401882, -0.0004921259304884630223, 0.000000000000000000 ) ) ;
#39894=CARTESIAN_POINT ( 'NONE',  ( 0.1787899950787401604, 0.01673228351833043817, 0.07405724077823318263 ) ) ;
#39901=CARTESIAN_POINT ( 'NONE',  ( -0.1787899950787401604, -1.813976377898992354, 0.07405724077823318263 ) ) ;
#39904=ORIENTED_EDGE ( 'NONE', *, *, #7679, .F. ) ;
#39909=CARTESIAN_POINT ( 'NONE',  ( -0.1787899950787401604, -0.8062263304339631897, -0.07405724077823318263 ) ) ;
#39911=CARTESIAN_POINT ( 'NONE',  ( -0.1694227370586289527, -0.08956103987234979857, 0.004342192889647520510 ) ) ;
#39927=CARTESIAN_POINT ( 'NONE',  ( 0.1270800023317771588, -0.8819335733625728313, -0.1270800023317771588 ) ) ;
#39931=CARTESIAN_POINT ( 'NONE',  ( -0.1113553986120547346, -0.5442913385826771977, -0.1113553986120547346 ) ) ;
#39932=CARTESIAN_POINT ( 'NONE',  ( -0.1635024568870425687, 0.1266995851085641056, 0.01633969686776765365 ) ) ;
#39948=CARTESIAN_POINT ( 'NONE',  ( -0.1264236179284866091, -1.142224409395055096, 0.1264236179284866091 ) ) ;
#39953=CARTESIAN_POINT ( 'NONE',  ( 0.1113553986120547346, -0.3179133857192444901, 0.1113553986120547346 ) ) ;
#39962=CARTESIAN_POINT ( 'NONE',  ( 0.1264236179284866091, -0.4740412910638843180, 0.1264236179284866091 ) ) ;
#39964=CARTESIAN_POINT ( 'NONE',  ( 0.02595745220638724302, -0.09842519685039370636, 0.1523733382129854319 ) ) ;
#39974=CARTESIAN_POINT ( 'NONE',  ( 0.07405724077823318263, -1.238188976324190005, -0.1787899950787401604 ) ) ;
#39975=CARTESIAN_POINT ( 'NONE',  ( -1.094772975963752103E-17, -1.309547244040724312, -0.1787899950787401882 ) ) ;
#39978=CARTESIAN_POINT ( 'NONE',  ( -0.07444174185955065859, -0.6235674316302897147, 0.1797182628040039087 ) ) ;
#39983=CARTESIAN_POINT ( 'NONE',  ( -0.1574803149606300301, -0.1875000000000000000, -0.06523048226347956391 ) ) ;
#39995=CARTESIAN_POINT ( 'NONE',  ( -0.1113553986120547346, -1.587598425089322696, 0.1113553986120547346 ) ) ;
#39996=CARTESIAN_POINT ( 'NONE',  ( 0.07405724077823318263, -0.7263779527021420046, -0.1787899950787401604 ) ) ;
#39998=CARTESIAN_POINT ( 'NONE',  ( -0.1574803149606300301, -1.132381889763780070, -0.06523048226347956391 ) ) ;
#40012=CARTESIAN_POINT ( 'NONE',  ( 0.06523048226347956391, -0.06938976367200050399, -0.1574803149606300301 ) ) ;
#40014=CARTESIAN_POINT ( 'NONE',  ( -0.1113553986120547346, -0.1309055117034966520, 0.1113553986120547346 ) ) ;
#40021=CARTESIAN_POINT ( 'NONE',  ( -0.1128178969825543304, -0.09851383988190079433, -0.1443091522045568953 ) ) ;
#40025=CARTESIAN_POINT ( 'NONE',  ( -0.07405724077823318263, -1.662525543032388420, 0.1787899950787401604 ) ) ;
#40029=CARTESIAN_POINT ( 'NONE',  ( -0.1264236179284866091, -0.3941929133320630219, 0.1264236179284866091 ) ) ;
#40030=CARTESIAN_POINT ( 'NONE',  ( 0.07405724077823318263, -0.9330708660879686311, 0.1787899950787401604 ) ) ;
#40031=CARTESIAN_POINT ( 'NONE',  ( -0.2471922963015220076, -0.09312803950196824054, -0.03901180619694211843 ) ) ;
#40035=CARTESIAN_POINT ( 'NONE',  ( 0.07444174185955046430, -0.1314414473783210302, -0.1797182628040039087 ) ) ;
#40037=CARTESIAN_POINT ( 'NONE',  ( -0.1264236179284866091, -0.09018302334734902559, 0.1264236179284866091 ) ) ;
#40038=CARTESIAN_POINT ( 'NONE',  ( 0.1787899950787401604, -0.2982283464029296116, 0.07405724077823318263 ) ) ;
#40048=FACE_OUTER_BOUND ( 'NONE', #45140, .T. ) ;
#40050=CARTESIAN_POINT ( 'NONE',  ( 0.1787899950787401882, -0.2219488188438744347, -2.189545951927503898E-17 ) ) ;
#40053=CARTESIAN_POINT ( 'NONE',  ( -0.07405724077823318263, -1.110236220418677533, -0.1787899950787401604 ) ) ;
#40063=CARTESIAN_POINT ( 'NONE',  ( -0.1574803149606300301, -1.122539369971214063, -0.06523048226347956391 ) ) ;
#40076=CARTESIAN_POINT ( 'NONE',  ( -0.07405724077823318263, -0.03740157474938609478, 0.1787899950787401604 ) ) ;
#40084=CARTESIAN_POINT ( 'NONE',  ( -0.1264236179284866091, -1.271285385552072933, 0.1264236179284866091 ) ) ;
#40087=CARTESIAN_POINT ( 'NONE',  ( -0.1787899950787401604, -0.3179133857730082058, -0.07405724077823318263 ) ) ;
#40096=CARTESIAN_POINT ( 'NONE',  ( 0.1787899950787401604, -1.681102362150960650, 0.07405724077823318263 ) ) ;
#40097=CARTESIAN_POINT ( 'NONE',  ( 0.07405724077823318263, -1.641732283410802573, 0.1787899950787401604 ) ) ;
#40100=CARTESIAN_POINT ( 'NONE',  ( -0.1730584022666810107, -0.09842519685039369248, -0.02721978519955341527 ) ) ;
#40101=CARTESIAN_POINT ( 'NONE',  ( -0.1797182628040039087, -1.302701289898007042, -0.07444174185955065859 ) ) ;
#40119=VECTOR ( 'NONE', #22879, 39.37007874015748143 ) ;
#40126=CARTESIAN_POINT ( 'NONE',  ( 3.284318927891251994E-17, -0.1087598424659214497, 0.1787899950787401882 ) ) ;
#40130=CARTESIAN_POINT ( 'NONE',  ( -0.1574803149606300301, 0.08809055118110237226, -0.06523048226347956391 ) ) ;
#40131=DIRECTION ( 'NONE',  ( 0.000000000000000000, 0.000000000000000000, 1.000000000000000000 ) ) ;
#40136=CARTESIAN_POINT ( 'NONE',  ( -0.1113553986120547346, 0.06594488199729076072, 0.1113553986120547346 ) ) ;
#40142=CARTESIAN_POINT ( 'NONE',  ( 0.1787899950787401604, -0.8997302674418365953, -0.07405724077823318263 ) ) ;
#40145=CARTESIAN_POINT ( 'NONE',  ( -0.1787899950787401882, 0.1569881890301415284, 0.000000000000000000 ) ) ;
#40158=CARTESIAN_POINT ( 'NONE',  ( 0.07444174185955046430, -0.8401028647011551387, -0.1797182628040039087 ) ) ;
#40162=CARTESIAN_POINT ( 'NONE',  ( 0.2471922904502826812, 0.08969147984773637172, -0.05033842647028097250 ) ) ;
#40171=CARTESIAN_POINT ( 'NONE',  ( 0.1787899950787401604, -0.8051181101824581576, -0.07405724077823318263 ) ) ;
#40180=CARTESIAN_POINT ( 'NONE',  ( 0.1574803149606299191, -1.543307086614173151, -1.928577636452523993E-17 ) ) ;
#40187=CARTESIAN_POINT ( 'NONE',  ( -0.1787899950787401604, -1.420275590497418250, 0.07405724077823318263 ) ) ;
#40190=EDGE_CURVE ( 'NONE', #37608, #33104, #14495, .T. ) ;
#40197=CARTESIAN_POINT ( 'NONE',  ( -0.1787899950787401604, -0.4518956217725454416, -0.07405724077823318263 ) ) ;
#40198=CARTESIAN_POINT ( 'NONE',  ( -0.08756112481127756308, -0.09842519685039370636, -0.1629625869553541495 ) ) ;
#40208=CARTESIAN_POINT ( 'NONE',  ( 0.1787899950787401604, -1.124999999946237228, -0.07405724077823318263 ) ) ;
#40210=CARTESIAN_POINT ( 'NONE',  ( -0.1787899950787401604, -1.380905511757260173, -0.07405724077823318263 ) ) ;
#40215=CARTESIAN_POINT ( 'NONE',  ( -0.1113553986120547346, -0.1899606299212598659, -0.1113553986120547346 ) ) ;
#40230=CARTESIAN_POINT ( 'NONE',  ( 3.284318927891251994E-17, -1.486712598371433103, 0.1787899950787401882 ) ) ;
#40231=CARTESIAN_POINT ( 'NONE',  ( 0.1574803149606300301, -1.570374015640505938, -0.06523048226347956391 ) ) ;
#40232=CARTESIAN_POINT ( 'NONE',  ( 0.07405724077823318263, -0.7805118109698575557, 0.1787899950787401604 ) ) ;
#40235=CARTESIAN_POINT ( 'NONE',  ( -0.1113553986120547346, -1.056102362204724532, -0.1113553986120547346 ) ) ;
#40244=TOROIDAL_SURFACE ( 'NONE', #18813, 0.2007874015748031815, 0.01968503937007873988 ) ;
#40254=VERTEX_POINT ( 'NONE', #17605 ) ;
#40257=CARTESIAN_POINT ( 'NONE',  ( 0.06244570574875708824, -0.09851384119049862165, -0.1836092180619330883 ) ) ;
#40259=ORIENTED_EDGE ( 'NONE', *, *, #21093, .F. ) ;
#40261=CARTESIAN_POINT ( 'NONE',  ( -1.094772975963752103E-17, -0.6796259841982046357, -0.1787899950787401882 ) ) ;
#40265=CARTESIAN_POINT ( 'NONE',  ( -0.1787899950787401882, -0.3991141731745826982, 0.000000000000000000 ) ) ;
#40266=CARTESIAN_POINT ( 'NONE',  ( 0.1264236179284866091, -0.8420275590013542866, -0.1264236179284866091 ) ) ;
#40268=CARTESIAN_POINT ( 'NONE',  ( -0.2471911001155968346, -0.08911307781785425541, -0.05219320342745862457 ) ) ;
#40271=CARTESIAN_POINT ( 'NONE',  ( -1.100456976456230270E-17, -0.2470910536775338395, -0.1797182628040039365 ) ) ;
#40272=CARTESIAN_POINT ( 'NONE',  ( 0.1264236179284866091, -0.1197105824024671250, 0.1264236179284866091 ) ) ;
#40273=CARTESIAN_POINT ( 'NONE',  ( -0.07405724077823318263, -0.05216535427694517224, -0.1787899950787401604 ) ) ;
#40281=CARTESIAN_POINT ( 'NONE',  ( -0.1898890638025484690, -0.07836638817766017340, 0.1758005714383346074 ) ) ;
#40286=CARTESIAN_POINT ( 'NONE',  ( 0.07405724077823318263, -0.2933070865604095467, -0.1787899950787401604 ) ) ;
#40289=CARTESIAN_POINT ( 'NONE',  ( -0.1787899950787401604, -1.139763779473794925, 0.07405724077823318263 ) ) ;
#40298=CARTESIAN_POINT ( 'NONE',  ( 0.06523048226347956391, -1.186515747923968300, 0.1574803149606297803 ) ) ;
#40311=CARTESIAN_POINT ( 'NONE',  ( -1.094772975963752103E-17, -0.01525590545804752021, -0.1787899950787401882 ) ) ;
#40317=CARTESIAN_POINT ( 'NONE',  ( 3.284318927891251994E-17, -1.345104283189868299, 0.1787899950787401882 ) ) ;
#40319=CARTESIAN_POINT ( 'NONE',  ( -0.1264236179284866091, -0.3203740156942680994, -0.1264236179284866091 ) ) ;
#40327=CARTESIAN_POINT ( 'NONE',  ( -0.1264236179284866091, -1.727854330654897685, 0.1264236179284866091 ) ) ;
#40330=CARTESIAN_POINT ( 'NONE',  ( 0.1797182628040039087, -1.479866644228716055, 0.07444174185955046430 ) ) ;
#40338=DIRECTION ( 'NONE',  ( 0.000000000000000000, 0.000000000000000000, 1.000000000000000000 ) ) ;
#40355=CARTESIAN_POINT ( 'NONE',  ( -9.642888182262618425E-18, 0.1200787401574803237, -0.1574803149606299191 ) ) ;
#40357=CARTESIAN_POINT ( 'NONE',  ( 0.1787899950787401882, -0.1776574802611972648, -2.189545951927503898E-17 ) ) ;
#40362=CARTESIAN_POINT ( 'NONE',  ( -0.03342428880116840584, -0.06208088008896742865, 0.2661310841544294870 ) ) ;
#40366=CARTESIAN_POINT ( 'NONE',  ( -0.1264236179284866091, -1.811515747977732405, 0.1264236179284866091 ) ) ;
#40376=CARTESIAN_POINT ( 'NONE',  ( -0.1787899950787401882, -0.7643956217725453861, 0.000000000000000000 ) ) ;
#40390=CARTESIAN_POINT ( 'NONE',  ( 0.1270800023317771588, -0.9311461717877698163, 0.1270800023317771588 ) ) ;
#40404=CARTESIAN_POINT ( 'NONE',  ( 0.07405724077823318263, -0.7362204723871804690, 0.1787899950787401604 ) ) ;
#40410=CARTESIAN_POINT ( 'NONE',  ( -0.06523048226347956391, -1.609744094488189337, -0.1574803149606300301 ) ) ;
#40419=CARTESIAN_POINT ( 'NONE',  ( -0.1574803149606299191, 0.06102362215477106361, 0.000000000000000000 ) ) ;
#40420=CARTESIAN_POINT ( 'NONE',  ( 0.1264236179284866091, -1.447342519631275692, 0.1264236179284866091 ) ) ;
#40430=CARTESIAN_POINT ( 'NONE',  ( -0.1264236179284866091, -0.4149861729536480914, -0.1264236179284866091 ) ) ;
#40431=CARTESIAN_POINT ( 'NONE',  ( -0.2387240754188476310, -0.08955950445031535256, -0.009354969050736969619 ) ) ;
#40439=CARTESIAN_POINT ( 'NONE',  ( 0.1264236179284866091, -1.407972440891118282, 0.1264236179284866091 ) ) ;
#40440=CARTESIAN_POINT ( 'NONE',  ( 3.284318927891251994E-17, -1.407972440891118282, 0.1787899950787401882 ) ) ;
#40449=CARTESIAN_POINT ( 'NONE',  ( 0.06523048226347956391, -0.3548228346456690496, -0.1574803149606300301 ) ) ;
#40454=CARTESIAN_POINT ( 'NONE',  ( -0.1264414976123398593, -0.09162967223036785902, -0.1264062623377731343 ) ) ;
#40458=CARTESIAN_POINT ( 'NONE',  ( -0.06523048226347956391, -0.5221456691838117781, 0.1574803149606297803 ) ) ;
#40460=CARTESIAN_POINT ( 'NONE',  ( -0.1908307771204775238, -0.07780576619187345999, -0.1752568734204362211 ) ) ;
#40464=CARTESIAN_POINT ( 'NONE',  ( -0.1787899950787401882, -1.496555118056472677, 0.000000000000000000 ) ) ;
#40465=CARTESIAN_POINT ( 'NONE',  ( -9.642888182262618425E-18, -1.602362204616881725, -0.1574803149606299191 ) ) ;
#40466=CARTESIAN_POINT ( 'NONE',  ( -1.094772975963752103E-17, -0.7239173227808818334, -0.1787899950787401882 ) ) ;
#40467=CARTESIAN_POINT ( 'NONE',  ( 2.892866454678787531E-17, -1.277559055118110187, 0.1574803149606299191 ) ) ;
#40471=ORIENTED_EDGE ( 'NONE', *, *, #21087, .T. ) ;
#40489=CARTESIAN_POINT ( 'NONE',  ( -0.2304022103396637655, -0.09842519685039370636, 0.06210465366844153401 ) ) ;
#40496=CARTESIAN_POINT ( 'NONE',  ( -0.1787899950787401882, -0.8321850393163149340, 0.000000000000000000 ) ) ;
#40497=CARTESIAN_POINT ( 'NONE',  ( 0.07405724077823318263, -0.4507874015210400209, -0.1787899950787401604 ) ) ;
#40499=CARTESIAN_POINT ( 'NONE',  ( -0.1787899950787401882, -0.9060039369541103005, 0.000000000000000000 ) ) ;
#40504=CARTESIAN_POINT ( 'NONE',  ( -1.100456976456230270E-17, -0.1683508961972187135, -0.1797182628040039365 ) ) ;
#40505=CARTESIAN_POINT ( 'NONE',  ( 2.892866454678787531E-17, 0.1397637795275590566, 0.1574803149606299191 ) ) ;
#40506=CARTESIAN_POINT ( 'NONE',  ( -0.1787899950787401882, -0.1235236219934805202, 0.000000000000000000 ) ) ;
#40507=CARTESIAN_POINT ( 'NONE',  ( 0.2471922711061203815, -0.07744971747249546068, -0.07831899213442956864 ) ) ;
#40518=CARTESIAN_POINT ( 'NONE',  ( 0.1787899950787401604, -0.2244094487651340231, 0.07405724077823318263 ) ) ;
#40520=CARTESIAN_POINT ( 'NONE',  ( 0.07405724077823318263, -1.154527559001354842, -0.1787899950787401604 ) ) ;
#40546=CARTESIAN_POINT ( 'NONE',  ( 0.1787899950787401882, -1.532112157205616221, -2.189545951927503898E-17 ) ) ;
#40549=CARTESIAN_POINT ( 'NONE',  ( 0.1787899950787401604, -0.3375984251430867999, 0.07405724077823318263 ) ) ;
#40559=CARTESIAN_POINT ( 'NONE',  ( -0.1787899950787401604, -1.661417322780881500, -0.07405724077823318263 ) ) ;
#40560=CARTESIAN_POINT ( 'NONE',  ( 0.07405724077823318263, -1.720472440891118726, 0.1787899950787401604 ) ) ;
#40565=CARTESIAN_POINT ( 'NONE',  ( -0.07444174185955065859, -1.346992628480683907, -0.1797182628040039087 ) ) ;
#40583=CARTESIAN_POINT ( 'NONE',  ( 0.1113553986120547346, -0.04232283464566929249, -0.1113553986120547346 ) ) ;
#40584=ORIENTED_EDGE ( 'NONE', *, *, #9712, .T. ) ;
#40585=CARTESIAN_POINT ( 'NONE',  ( 0.07444174185955065859, -0.1068351481657228014, 0.1797182628040039087 ) ) ;
#40592=CARTESIAN_POINT ( 'NONE',  ( -0.07405724077823318263, -0.1112204723871813017, 0.1787899950787401604 ) ) ;
#40596=CARTESIAN_POINT ( 'NONE',  ( 0.1895013542076671997, -0.07859528327911675938, -0.1760244123199382060 ) ) ;
#40598=CARTESIAN_POINT ( 'NONE',  ( 0.06523048226347956391, 0.03395669302091285091, 0.1574803149606297803 ) ) ;
#40604=CYLINDRICAL_SURFACE ( 'NONE', #18772, 0.1574803149606299191 ) ;
#40606=CARTESIAN_POINT ( 'NONE',  ( 0.1787899950787401882, -0.8234507398827816127, -2.189545951927503898E-17 ) ) ;
#40616=CARTESIAN_POINT ( 'NONE',  ( -0.07405724077823318263, -0.5246062991588343882, -0.1787899950787401604 ) ) ;
#40621=CARTESIAN_POINT ( 'NONE',  ( 3.301370929368692659E-17, -1.054177667850761946, 0.1797182628040039365 ) ) ;
#40630=CARTESIAN_POINT ( 'NONE',  ( 0.07405724077823318263, -0.7755905511273385455, 0.1787899950787401604 ) ) ;
#40635=CARTESIAN_POINT ( 'NONE',  ( -0.06523048226347956391, -1.688484251968503269, -0.1574803149606300301 ) ) ;
#40643=CARTESIAN_POINT ( 'NONE',  ( 0.06523048226347956391, -0.3056102361129455214, -0.1574803149606300301 ) ) ;
#40651=CARTESIAN_POINT ( 'NONE',  ( 0.1574803149606300301, -0.03494094477436274215, -0.06523048226347956391 ) ) ;
#40653=CARTESIAN_POINT ( 'NONE',  ( 0.1321676148590689159, 0.1299212598425196763, -0.1026092226670043267 ) ) ;
#40656=CARTESIAN_POINT ( 'NONE',  ( -0.1787899950787401882, -0.3313247556308138164, 0.000000000000000000 ) ) ;
#40657=CARTESIAN_POINT ( 'NONE',  ( -0.2269653392414791304, -0.08955981648012203977, 0.06100550293770786586 ) ) ;
#40659=CYLINDRICAL_SURFACE ( 'NONE', #46303, 0.1574803149606299191 ) ;
#40665=EDGE_LOOP ( 'NONE', ( #31666, #45560, #19236, #26178 ) ) ;
#40668=CARTESIAN_POINT ( 'NONE',  ( -1.094772975963752103E-17, -1.353838582623401621, -0.1787899950787401882 ) ) ;
#40669=CARTESIAN_POINT ( 'NONE',  ( 0.07405724077823318263, -1.469488188922614791, -0.1787899950787401604 ) ) ;
#40678=CARTESIAN_POINT ( 'NONE',  ( 0.1113553986120547346, -0.2785433070866141780, -0.1113553986120547346 ) ) ;
#40694=CARTESIAN_POINT ( 'NONE',  ( 0.1787899950787401604, -1.518700787347811554, 0.07405724077823318263 ) ) ;
#40695=CARTESIAN_POINT ( 'NONE',  ( -0.1264236179284866091, -0.7878937007336378473, 0.1264236179284866091 ) ) ;
#40696=CARTESIAN_POINT ( 'NONE',  ( 0.06523048226347956391, -1.260334645669290321, -0.1574803149606300301 ) ) ;
#40719=CARTESIAN_POINT ( 'NONE',  ( 0.07340243826527893811, -0.09851382364606299513, 0.1314582435714135855 ) ) ;
#40729=CARTESIAN_POINT ( 'NONE',  ( 0.1787899950787401604, -0.8543307086076546986, 0.07405724077823318263 ) ) ;
#40730=CARTESIAN_POINT ( 'NONE',  ( 0.07405724077823318263, -0.4655511810485986057, 0.1787899950787401604 ) ) ;
#40731=CARTESIAN_POINT ( 'NONE',  ( -0.1787899950787401604, -1.139763779473794925, 0.07405724077823318263 ) ) ;
#40735=CARTESIAN_POINT ( 'NONE',  ( 0.1797182628040039365, -0.3356737308428881517, -2.200913952912460540E-17 ) ) ;
#40737=CARTESIAN_POINT ( 'NONE',  ( -0.1787899950787401882, -0.04478346451316559534, 0.000000000000000000 ) ) ;
#40750=CARTESIAN_POINT ( 'NONE',  ( -0.1264236179284866091, -0.2367125983714334636, 0.1264236179284866091 ) ) ;
#40753=CARTESIAN_POINT ( 'NONE',  ( -0.1787899950787401882, -1.220964566875370139, 0.000000000000000000 ) ) ;
#40757=ORIENTED_EDGE ( 'NONE', *, *, #46039, .F. ) ;
#40761=CARTESIAN_POINT ( 'NONE',  ( 0.1113553986120547346, -1.174212598317669221, -0.1113553986120547346 ) ) ;
#40764=CARTESIAN_POINT ( 'NONE',  ( -0.09161186067205415173, -0.09842317194137423231, -0.1536306822207036404 ) ) ;
#40781=CARTESIAN_POINT ( 'NONE',  ( 0.1787899950787401882, -1.414001920985143768, -2.189545951927503898E-17 ) ) ;
#40783=CARTESIAN_POINT ( 'NONE',  ( 0.1787899950787401604, -0.4163385826234020093, 0.07405724077823318263 ) ) ;
#40791=CARTESIAN_POINT ( 'NONE',  ( 0.1787899950787401882, -1.796751968450173376, -2.189545951927503898E-17 ) ) ;
#40792=CARTESIAN_POINT ( 'NONE',  ( -0.1264236179284866091, -1.688484251914740275, 0.1264236179284866091 ) ) ;
#40798=CARTESIAN_POINT ( 'NONE',  ( -0.1574803149606297803, -0.7731299212598427006, 0.06523048226347956391 ) ) ;
#40799=CARTESIAN_POINT ( 'NONE',  ( 0.07444174185955046430, -1.430654045803517294, -0.1797182628040039087 ) ) ;
#40805=CARTESIAN_POINT ( 'NONE',  ( 0.07405724077823318263, 0.1397637795813224670, -0.1787899950787401604 ) ) ;
#40812=ORIENTED_EDGE ( 'NONE', *, *, #21029, .F. ) ;
#40815=CARTESIAN_POINT ( 'NONE',  ( 0.1270800023317771588, -0.05516191981926597820, -0.1270800023317771588 ) ) ;
#40818=CARTESIAN_POINT ( 'NONE',  ( -0.1787899950787401882, -1.265255905458047225, 0.000000000000000000 ) ) ;
#40826=CARTESIAN_POINT ( 'NONE',  ( -0.1264236179284866091, -0.1235236219934805202, -0.1264236179284866091 ) ) ;
#40835=CARTESIAN_POINT ( 'NONE',  ( -9.642888182262618425E-18, -0.1062992124908982289, -0.1574803149606299191 ) ) ;
#40841=CARTESIAN_POINT ( 'NONE',  ( -0.1787899950787401604, -0.9243365666544370862, -0.07405724077823318263 ) ) ;
#40843=CARTESIAN_POINT ( 'NONE',  ( 0.1264236179284866091, 0.06348425202226751218, -0.1264236179284866091 ) ) ;
#40853=CARTESIAN_POINT ( 'NONE',  ( 0.1797182628040039087, -0.9286855418665098671, 0.07444174185955046430 ) ) ;
#40866=CARTESIAN_POINT ( 'NONE',  ( 0.1787899950787401604, -0.7263779527021420046, -0.07405724077823318263 ) ) ;
#40869=CARTESIAN_POINT ( 'NONE',  ( 0.1574803149606299191, 0.1299212598425196763, 0.000000000000000000 ) ) ;
#40870=CARTESIAN_POINT ( 'NONE',  ( 0.000000000000000000, 0.09842519685039370636, -0.2204724409448818867 ) ) ;
#40873=CARTESIAN_POINT ( 'NONE',  ( -0.1574803149606297803, -1.718011811023622881, 0.06523048226347956391 ) ) ;
#40893=CARTESIAN_POINT ( 'NONE',  ( 0.009906661468957056113, 0.04209688371799798906, -0.2797134572002689112 ) ) ;
#40895=CARTESIAN_POINT ( 'NONE',  ( -0.1787899950787401604, -0.4863444406701833977, 0.07405724077823318263 ) ) ;
#40896=CARTESIAN_POINT ( 'NONE',  ( -0.2007511360401751932, -0.08955985698252086347, 0.1161810953340854241 ) ) ;
#40900=CARTESIAN_POINT ( 'NONE',  ( 0.1264236179284866091, -1.773253889489082580, 0.1264236179284866091 ) ) ;
#40902=CARTESIAN_POINT ( 'NONE',  ( 0.2471922332844968817, -0.07944658092491525825, 0.07441910580888103088 ) ) ;
#40904=CARTESIAN_POINT ( 'NONE',  ( 0.1787899950787401604, -1.361220472387181690, -0.07405724077823318263 ) ) ;
#40905=CARTESIAN_POINT ( 'NONE',  ( -0.07405724077823318263, -1.543307086560409713, -0.1787899950787401604 ) ) ;
#40912=CARTESIAN_POINT ( 'NONE',  ( -7.939671275311751530E-17, -0.03219022224904082713, -0.2854330708661417804 ) ) ;
#40918=CARTESIAN_POINT ( 'NONE',  ( -0.1219444983797640936, -0.09073875858372155989, -0.1307555171292179852 ) ) ;
#40922=CARTESIAN_POINT ( 'NONE',  ( -0.1674689075051689624, -0.08956125648410076523, 0.01721656813326377655 ) ) ;
#40929=CARTESIAN_POINT ( 'NONE',  ( -0.07405724077823318263, -1.543307086560409713, -0.1787899950787401604 ) ) ;
#40930=CARTESIAN_POINT ( 'NONE',  ( -0.1264236179284866091, -0.9158464566391496531, -0.1264236179284866091 ) ) ;
#40931=CARTESIAN_POINT ( 'NONE',  ( -0.1113553986120547346, -1.164370078740157632, 0.1113553986120547346 ) ) ;
#40939=CARTESIAN_POINT ( 'NONE',  ( 0.06523048226347956391, -1.343996062884598386, 0.1574803149606297803 ) ) ;
#40957=CARTESIAN_POINT ( 'NONE',  ( -0.1275616080144442999, -0.09842519685039370636, -0.2189039336074421471 ) ) ;
#40962=ORIENTED_EDGE ( 'NONE', *, *, #2794, .T. ) ;
#40964=CARTESIAN_POINT ( 'NONE',  ( 0.07405724077823318263, -0.8592519684501739308, 0.1787899950787401604 ) ) ;
#40965=CARTESIAN_POINT ( 'NONE',  ( 0.1787899950787401882, -1.043799212544661348, -2.189545951927503898E-17 ) ) ;
#40970=CARTESIAN_POINT ( 'NONE',  ( 0.1270800023317771588, -0.2913823922602110095, -0.1270800023317771588 ) ) ;
#40971=FACE_OUTER_BOUND ( 'NONE', #23248, .T. ) ;
#40973=CARTESIAN_POINT ( 'NONE',  ( 0.1264236179284866091, -0.1874999999462366451, 0.1264236179284866091 ) ) ;
#40977=ADVANCED_FACE ( 'NONE', ( #40048 ), #32530, .T. ) ;
#40979=FACE_OUTER_BOUND ( 'NONE', #24492, .T. ) ;
#40980=DIRECTION ( 'NONE',  ( 1.000000000000000000, 0.000000000000000000, 0.000000000000000000 ) ) ;
#40988=CARTESIAN_POINT ( 'NONE',  ( -0.07405724077823318263, -0.3277559054580475584, -0.1787899950787401604 ) ) ;
#40990=CARTESIAN_POINT ( 'NONE',  ( -0.07405724077823318263, -1.252952755851747924, 0.1787899950787401604 ) ) ;
#40999=CARTESIAN_POINT ( 'NONE',  ( -0.1188990808483700867, -0.09842519868841002884, -0.1335248378736948738 ) ) ;
#41014=CARTESIAN_POINT ( 'NONE',  ( 0.1264236179284866091, -1.458293259567820854, 0.1264236179284866091 ) ) ;
#41017=CARTESIAN_POINT ( 'NONE',  ( 0.1264236179284866091, -0.4089566928596221063, -0.1264236179284866091 ) ) ;
#41025=CARTESIAN_POINT ( 'NONE',  ( -0.1787899950787401604, 0.09928548058965885881, -0.07405724077823318263 ) ) ;
#41026=CARTESIAN_POINT ( 'NONE',  ( -0.1787899950787401882, -1.693405511757259951, 0.000000000000000000 ) ) ;
#41031=CARTESIAN_POINT ( 'NONE',  ( 0.1574803149606299191, -0.7165354330708662012, -1.928577636452523993E-17 ) ) ;
#41033=CARTESIAN_POINT ( 'NONE',  ( -1.100456976456230270E-17, -1.467563494622415421, -0.1797182628040039365 ) ) ;
#41053=CARTESIAN_POINT ( 'NONE',  ( -0.07444174185955065859, 0.006353828212230052709, 0.1797182628040039087 ) ) ;
#41054=CARTESIAN_POINT ( 'NONE',  ( -0.1264236179284866091, -1.220964566875370139, 0.1264236179284866091 ) ) ;
#41059=CARTESIAN_POINT ( 'NONE',  ( -0.1574803149606300301, 0.04872047244094490637, -0.06523048226347956391 ) ) ;
#41062=CARTESIAN_POINT ( 'NONE',  ( 0.1787899950787401882, -0.09891732278088229136, -2.189545951927503898E-17 ) ) ;
#41067=CARTESIAN_POINT ( 'NONE',  ( 0.06523048226347956391, 0.009350393808314452077, -0.1574803149606300301 ) ) ;
#41074=CARTESIAN_POINT ( 'NONE',  ( 0.07405724077823318263, -0.9095727871268751707, 0.1787899950787401604 ) ) ;
#41076=CARTESIAN_POINT ( 'NONE',  ( 0.1787899950787401604, 0.01673228351833043817, 0.07405724077823318263 ) ) ;
#41082=CARTESIAN_POINT ( 'NONE',  ( -0.07405724077823318263, -0.5098425196312756924, 0.1787899950787401604 ) ) ;
#41083=ADVANCED_FACE ( 'NONE', ( #9845 ), #25613, .T. ) ;
#41087=CARTESIAN_POINT ( 'NONE',  ( 0.1797182628040039087, -1.081244596984620499, -0.07444174185955065859 ) ) ;
#41102=CARTESIAN_POINT ( 'NONE',  ( -0.1787899950787401604, -0.7460629920722210429, 0.07405724077823318263 ) ) ;
#41105=DIRECTION ( 'NONE',  ( 1.000000000000000000, 0.000000000000000000, 0.000000000000000000 ) ) ;
#41110=CARTESIAN_POINT ( 'NONE',  ( -0.1113553986120547346, -1.636811023622047223, 0.1113553986120547346 ) ) ;
#41118=CARTESIAN_POINT ( 'NONE',  ( -0.1113553986120547346, 0.06594488199729076072, 0.1113553986120547346 ) ) ;
#41119=CARTESIAN_POINT ( 'NONE',  ( 0.07405724077823318263, -1.528543307032852239, 0.1787899950787401604 ) ) ;
#41124=CARTESIAN_POINT ( 'NONE',  ( 3.284318927891251994E-17, -0.5970727871268759479, 0.1787899950787401882 ) ) ;
#41125=CARTESIAN_POINT ( 'NONE',  ( -0.1827272056907964515, -0.08955978927791437283, 0.1407872760489078667 ) ) ;
#41130=CARTESIAN_POINT ( 'NONE',  ( -0.1787899950787401604, -1.790478298937899115, -0.07405724077823318263 ) ) ;
#41137=CARTESIAN_POINT ( 'NONE',  ( -0.07405724077823318263, -1.351377952702143004, -0.1787899950787401604 ) ) ;
#41138=CARTESIAN_POINT ( 'NONE',  ( 3.284318927891251994E-17, -1.526082677111590513, 0.1787899950787401882 ) ) ;
#41154=CARTESIAN_POINT ( 'NONE',  ( -0.1307509148717837799, -0.08955578701844334188, 0.09650363397519905184 ) ) ;
#41160=CARTESIAN_POINT ( 'NONE',  ( -0.1787899950787401882, -1.575295275536787276, 0.000000000000000000 ) ) ;
#41161=CARTESIAN_POINT ( 'NONE',  ( -0.07405724077823318263, -0.8395669290800948925, -0.1787899950787401604 ) ) ;
#41162=CARTESIAN_POINT ( 'NONE',  ( 0.1574803149606300301, -1.147145669291337766, -0.06523048226347956391 ) ) ;
#41170=CARTESIAN_POINT ( 'NONE',  ( 2.892866454678787531E-17, -1.307086614065700703, 0.1574803149606299191 ) ) ;
#41183=CARTESIAN_POINT ( 'NONE',  ( -0.1397729047152643789, -0.09842519685039370636, 0.1853948292088582472 ) ) ;
#41190=CARTESIAN_POINT ( 'NONE',  ( 0.07405724077823318263, -0.9379921259304876413, 0.1787899950787401604 ) ) ;
#41192=CARTESIAN_POINT ( 'NONE',  ( -1.094772975963752103E-17, -0.9945866141194644738, -0.1787899950787401882 ) ) ;
#41194=CARTESIAN_POINT ( 'NONE',  ( -0.1797182628040039087, -0.3971894788743842164, -0.07444174185955065859 ) ) ;
#41195=CARTESIAN_POINT ( 'NONE',  ( -0.1574803149606300301, 0.1274606299212597549, -0.06523048226347956391 ) ) ;
#41196=CARTESIAN_POINT ( 'NONE',  ( -0.1787899950787401882, -0.1628937007336379861, 0.000000000000000000 ) ) ;
#41206=CARTESIAN_POINT ( 'NONE',  ( -0.07405724077823318263, -0.4852362204186770889, -0.1787899950787401604 ) ) ;
#41208=CARTESIAN_POINT ( 'NONE',  ( 0.1787899950787401604, -1.159448818843874074, -0.07405724077823318263 ) ) ;
#41221=CARTESIAN_POINT ( 'NONE',  ( -0.1138125304461556353, -0.09842519813797928618, -0.1380434466211696298 ) ) ;
#41238=CARTESIAN_POINT ( 'NONE',  ( -0.07405724077823318263, -1.441068850119002542, -0.1787899950787401604 ) ) ;
#41240=CARTESIAN_POINT ( 'NONE',  ( 0.1787899950787401604, -0.4557086613635593086, 0.07405724077823318263 ) ) ;
#41252=CARTESIAN_POINT ( 'NONE',  ( 0.1787899950787401604, -1.794291338528913426, -0.07405724077823318263 ) ) ;
#41253=CARTESIAN_POINT ( 'NONE',  ( -0.1264236179284866091, -1.767224409395055318, 0.1264236179284866091 ) ) ;
#41259=CARTESIAN_POINT ( 'NONE',  ( 0.06523048226347956391, -0.6697834645669303866, -0.1574803149606300301 ) ) ;
#41261=CARTESIAN_POINT ( 'NONE',  ( 0.1270800023317771588, -1.482327274149974450, 0.1270800023317771588 ) ) ;
#41263=CARTESIAN_POINT ( 'NONE',  ( -0.1574803149606300301, -0.4532480313885357548, -0.06523048226347956391 ) ) ;
#41272=CARTESIAN_POINT ( 'NONE',  ( 0.07405724077823318263, 0.04625984257344856188, 0.1787899950787401604 ) ) ;
#41284=CARTESIAN_POINT ( 'NONE',  ( -0.1797182628040039087, 0.001432568369710361233, 0.07444174185955065859 ) ) ;
#41285=CARTESIAN_POINT ( 'NONE',  ( 0.1787899950787401882, -1.245570866087968520, -2.189545951927503898E-17 ) ) ;
#41300=CARTESIAN_POINT ( 'NONE',  ( 0.1113553986120547346, -0.08169291327829980576, 0.1113553986120547346 ) ) ;
#41307=CARTESIAN_POINT ( 'NONE',  ( 0.07405724077823318263, -1.012919243819789594, -0.1787899950787401604 ) ) ;
#41309=CARTESIAN_POINT ( 'NONE',  ( 0.1264236179284866091, 0.05364173233722803469, 0.1264236179284866091 ) ) ;
#41316=CARTESIAN_POINT ( 'NONE',  ( 0.1787899950787401604, -0.6919291338045056028, -0.07405724077823318263 ) ) ;
#41321=CARTESIAN_POINT ( 'NONE',  ( 0.07444174185955046430, -0.9582131009216291462, -0.1797182628040039087 ) ) ;
#41325=CONICAL_SURFACE ( 'NONE', #25298, 0.1673228346456692994, 0.7853981633974532750 ) ;
#41331=CARTESIAN_POINT ( 'NONE',  ( -0.1787899950787401882, 0.07824803154982658271, 0.000000000000000000 ) ) ;
#41337=CARTESIAN_POINT ( 'NONE',  ( -0.1264236179284866091, -0.9502952755367874982, -0.1264236179284866091 ) ) ;
#41340=CARTESIAN_POINT ( 'NONE',  ( 0.1574803149606299191, -1.730314960522393752, -1.928577636452523993E-17 ) ) ;
#41343=CARTESIAN_POINT ( 'NONE',  ( 0.1753418932787807749, 0.1299212598425196763, 0.07262899196590184847 ) ) ;
#41344=CARTESIAN_POINT ( 'NONE',  ( 0.1574803149606300301, -1.742618110236221041, 0.06523048226347956391 ) ) ;
#41348=ORIENTED_EDGE ( 'NONE', *, *, #5999, .T. ) ;
#41349=CARTESIAN_POINT ( 'NONE',  ( -0.1787899950787401604, -1.464566929080096225, -0.07405724077823318263 ) ) ;
#41358=CARTESIAN_POINT ( 'NONE',  ( -1.094772975963752103E-17, -0.6167578264969547641, -0.1787899950787401882 ) ) ;
#41359=CARTESIAN_POINT ( 'NONE',  ( 0.1048138276931706719, -0.09842519685039370636, 0.1042338764169748050 ) ) ;
#41367=CARTESIAN_POINT ( 'NONE',  ( -0.1264236179284866091, -1.792938928859161507, -0.1264236179284866091 ) ) ;
#41371=CARTESIAN_POINT ( 'NONE',  ( 0.1787899950787401604, -1.366141732229700478, 0.07405724077823318263 ) ) ;
#41372=CARTESIAN_POINT ( 'NONE',  ( 0.07405724077823318263, -1.484251968450174930, 0.1787899950787401604 ) ) ;
#41379=CARTESIAN_POINT ( 'NONE',  ( -0.1574803149606299191, -0.3425196850393700809, 0.000000000000000000 ) ) ;
#41387=CARTESIAN_POINT ( 'NONE',  ( 0.1574803149606300301, -0.5516732282389297248, 0.06523048226347956391 ) ) ;
#41391=CARTESIAN_POINT ( 'NONE',  ( -0.1406443466276429688, -0.08955922997629965632, 0.08377781526596418671 ) ) ;
#41400=CARTESIAN_POINT ( 'NONE',  ( -0.1113553986120547346, -0.02263779527559055260, 0.1113553986120547346 ) ) ;
#41401=CARTESIAN_POINT ( 'NONE',  ( 0.1264236179284866091, -1.678641732229700922, 0.1264236179284866091 ) ) ;
#41402=CARTESIAN_POINT ( 'NONE',  ( 0.1787899950787401882, -0.8912401574265511606, -2.189545951927503898E-17 ) ) ;
#41404=CARTESIAN_POINT ( 'NONE',  ( -0.1574803149606297803, -1.166830708661416693, 0.06523048226347956391 ) ) ;
#41412=CARTESIAN_POINT ( 'NONE',  ( 0.1113553986120547346, -1.380905511703496069, 0.1113553986120547346 ) ) ;
#41428=CARTESIAN_POINT ( 'NONE',  ( -0.2379070121699287110, -0.09842519685039370636, 0.03196672700780228693 ) ) ;
#41436=CARTESIAN_POINT ( 'NONE',  ( 0.1264236179284866091, -0.8961614172690708369, 0.1264236179284866091 ) ) ;
#41437=CARTESIAN_POINT ( 'NONE',  ( 0.1787899950787401604, -1.124999999946237228, 0.07405724077823318263 ) ) ;
#41440=CARTESIAN_POINT ( 'NONE',  ( 0.1797182628040039087, -0.2938430221814707366, -0.07444174185955065859 ) ) ;
#41441=CARTESIAN_POINT ( 'NONE',  ( 0.06523048226347956391, 0.1028543307086613318, 0.1574803149606297803 ) ) ;
#41444=EDGE_CURVE ( 'NONE', #43211, #47206, #11717, .T. ) ;
#41446=DIRECTION ( 'NONE',  ( 0.000000000000000000, 1.000000000000000000, 0.000000000000000000 ) ) ;
#41447=CARTESIAN_POINT ( 'NONE',  ( 2.892866454678787531E-17, -0.9921259841444409755, 0.1574803149606299191 ) ) ;
#41448=CARTESIAN_POINT ( 'NONE',  ( 0.1264236179284866091, -0.4630905511273386010, 0.1264236179284866091 ) ) ;
#41450=CARTESIAN_POINT ( 'NONE',  ( -0.1787899950787401604, -1.257874015694269376, 0.07405724077823318263 ) ) ;
#41454=EDGE_LOOP ( 'NONE', ( #41833, #38364, #22455, #18167, #23412, #29995 ) ) ;
#41458=CARTESIAN_POINT ( 'NONE',  ( -0.06523048226347956391, -1.245570866034205304, -0.1574803149606300301 ) ) ;
#41463=CARTESIAN_POINT ( 'NONE',  ( 0.06474555581190044595, -0.09842519435343592693, -0.1666564064369808196 ) ) ;
#41475=CARTESIAN_POINT ( 'NONE',  ( 3.284318927891251994E-17, -1.463214519410340531, 0.1787899950787401882 ) ) ;
#41478=CARTESIAN_POINT ( 'NONE',  ( 0.1787899950787401882, -0.4926181101824567143, -2.189545951927503898E-17 ) ) ;
#41488=CARTESIAN_POINT ( 'NONE',  ( -0.1264236179284866091, -1.772145669237574994, 0.1264236179284866091 ) ) ;
#41489=CARTESIAN_POINT ( 'NONE',  ( 0.07405724077823318263, -1.759842519631276581, 0.1787899950787401604 ) ) ;
#41494=CARTESIAN_POINT ( 'NONE',  ( -0.1574803149606300301, -0.7780511811023617108, -0.06523048226347956391 ) ) ;
#41496=CARTESIAN_POINT ( 'NONE',  ( -0.1797182628040039365, -1.497091053677533479, 0.000000000000000000 ) ) ;
#41497=DIRECTION ( 'NONE',  ( 0.000000000000000000, 0.000000000000000000, 1.000000000000000000 ) ) ;
#41498=CARTESIAN_POINT ( 'NONE',  ( 0.1574803149606299191, -0.4704724408373543443, -1.928577636452523993E-17 ) ) ;
#41503=ORIENTED_EDGE ( 'NONE', *, *, #16935, .F. ) ;
#41505=EDGE_CURVE ( 'NONE', #35894, #2394, #5355, .T. ) ;
#41508=CARTESIAN_POINT ( 'NONE',  ( 0.1787899950787401604, 0.09547244099864542199, -0.07405724077823318263 ) ) ;
#41520=CARTESIAN_POINT ( 'NONE',  ( -9.642888182262618425E-18, -1.051181102254677313, -0.1574803149606299191 ) ) ;
#41521=CARTESIAN_POINT ( 'NONE',  ( -0.1787899950787401882, -1.304625984198204636, 0.000000000000000000 ) ) ;
#41534=CARTESIAN_POINT ( 'NONE',  ( -0.1574803149606299191, 0.02165354341461366364, 0.000000000000000000 ) ) ;
#41543=CARTESIAN_POINT ( 'NONE',  ( 0.1264236179284866091, -0.9366397162607342786, -0.1264236179284866091 ) ) ;
#41544=CARTESIAN_POINT ( 'NONE',  ( 0.1787899950787401604, -0.02263779522182702078, 0.07405724077823318263 ) ) ;
#41546=ORIENTED_EDGE ( 'NONE', *, *, #42772, .F. ) ;
#41547=CARTESIAN_POINT ( 'NONE',  ( 3.624546087963248077E-17, -0.09842519685039370636, 0.2854330708661417804 ) ) ;
#41549=CARTESIAN_POINT ( 'NONE',  ( -0.07405724077823318263, -0.6033464566391496531, -0.1787899950787401604 ) ) ;
#41552=CARTESIAN_POINT ( 'NONE',  ( -0.1797182628040039087, -1.100929636354699426, 0.07444174185955065859 ) ) ;
#41553=CARTESIAN_POINT ( 'NONE',  ( 0.1747918830520822919, 0.1299212598425196763, 0.01616506989262271946 ) ) ;
#41564=CARTESIAN_POINT ( 'NONE',  ( 0.06523048226347956391, -0.6747047243019220764, 0.1574803149606297803 ) ) ;
#41566=CARTESIAN_POINT ( 'NONE',  ( -0.07405724077823318263, 0.1250000000537635492, 0.1787899950787401604 ) ) ;
#41577=CARTESIAN_POINT ( 'NONE',  ( 0.06523048226347956391, -1.737696850286174266, 0.1574803149606297803 ) ) ;
#41579=ORIENTED_EDGE ( 'NONE', *, *, #30083, .T. ) ;
#41584=CARTESIAN_POINT ( 'NONE',  ( -0.1113553986120547346, -1.794291338582677087, 0.1113553986120547346 ) ) ;
#41589=CARTESIAN_POINT ( 'NONE',  ( -0.1264236179284866091, -1.575295275536787276, 0.1264236179284866091 ) ) ;
#41594=CARTESIAN_POINT ( 'NONE',  ( -0.1264236179284866091, -0.5330964091741204891, -0.1264236179284866091 ) ) ;
#41595=CARTESIAN_POINT ( 'NONE',  ( -0.1699750452893318831, -0.08956104039312501319, -0.005819416704781811035 ) ) ;
#41596=CARTESIAN_POINT ( 'NONE',  ( 0.1113553986120547346, 0.04625984262721204859, -0.1113553986120547346 ) ) ;
#41598=CARTESIAN_POINT ( 'NONE',  ( -0.04259491748599998628, -0.09487271926367001063, 0.1523944991998174292 ) ) ;
#41608=CARTESIAN_POINT ( 'NONE',  ( 3.284318927891251994E-17, -1.531003936954110189, 0.1787899950787401882 ) ) ;
#41609=CARTESIAN_POINT ( 'NONE',  ( 0.1787899950787401604, -1.597440944828127485, 0.07405724077823318263 ) ) ;
#41616=CARTESIAN_POINT ( 'NONE',  ( 0.1574803149606299191, -0.4803149606299212948, -1.928577636452523993E-17 ) ) ;
#41623=DIRECTION ( 'NONE',  ( 0.000000000000000000, -1.000000000000000000, 0.000000000000000000 ) ) ;
#41629=CARTESIAN_POINT ( 'NONE',  ( -0.1598598147400959735, -0.08956144258305162587, 0.04681090282771781935 ) ) ;
#41630=CARTESIAN_POINT ( 'NONE',  ( -0.1264236179284866091, -0.5565944881352126172, -0.1264236179284866091 ) ) ;
#41640=CARTESIAN_POINT ( 'NONE',  ( -0.1787899950787401604, -1.690944881836001334, 0.07405724077823318263 ) ) ;
#41641=CARTESIAN_POINT ( 'NONE',  ( 0.07405724077823318263, -0.9625984251430860228, -0.1787899950787401604 ) ) ;
#41642=CARTESIAN_POINT ( 'NONE',  ( -0.06523048226347956391, -1.319389763779527769, 0.1574803149606297803 ) ) ;
#41661=CARTESIAN_POINT ( 'NONE',  ( 0.009745153983727742816, -0.04193537623276881454, -0.2798067035903422095 ) ) ;
#41665=CARTESIAN_POINT ( 'NONE',  ( 0.1188451152720541443, -0.09842519685039231858, -0.1576307852885025784 ) ) ;
#41673=CARTESIAN_POINT ( 'NONE',  ( 3.284318927891251994E-17, -1.058562992072220377, 0.1787899950787401882 ) ) ;
#41674=CARTESIAN_POINT ( 'NONE',  ( -0.1787899950787401604, -1.021653543253323138, 0.07405724077823318263 ) ) ;
#41677=CARTESIAN_POINT ( 'NONE',  ( -0.1797182628040039365, -0.2766186127326519251, 0.000000000000000000 ) ) ;
#41679=CARTESIAN_POINT ( 'NONE',  ( 0.06523048226347956391, 0.02411417322834644855, 0.1574803149606297803 ) ) ;
#41692=CARTESIAN_POINT ( 'NONE',  ( -0.06523048226347956391, -0.9699803148531034314, -0.1574803149606300301 ) ) ;
#41693=CARTESIAN_POINT ( 'NONE',  ( -0.1787899950787401604, -0.4753937007336378473, 0.07405724077823318263 ) ) ;
#41695=CARTESIAN_POINT ( 'NONE',  ( 0.07405724077823318263, -1.272637795221826629, -0.1787899950787401604 ) ) ;
#41716=CARTESIAN_POINT ( 'NONE',  ( -0.1098090583144935017, -0.09851385237441358245, -0.2293689557742909502 ) ) ;
#41722=CARTESIAN_POINT ( 'NONE',  ( 0.07405724077823318263, -1.603470424922151416, -0.1787899950787401604 ) ) ;
#41725=CARTESIAN_POINT ( 'NONE',  ( -0.1787899950787401604, -0.4704724408911186706, 0.07405724077823318263 ) ) ;
#41730=CARTESIAN_POINT ( 'NONE',  ( -0.1787899950787401604, -0.2391732282926934683, 0.07405724077823318263 ) ) ;
#41735=CARTESIAN_POINT ( 'NONE',  ( 0.07405724077823318263, -1.804133858213953889, 0.1787899950787401604 ) ) ;
#41736=CARTESIAN_POINT ( 'NONE',  ( 0.1787899950787401882, -1.791830708607653699, -2.189545951927503898E-17 ) ) ;
#41741=CARTESIAN_POINT ( 'NONE',  ( 0.1574803149606299191, -0.6771653543307086798, -1.928577636452523993E-17 ) ) ;
#41743=CARTESIAN_POINT ( 'NONE',  ( -1.100456976456230270E-17, -1.585673730842887652, -0.1797182628040039365 ) ) ;
#41753=CARTESIAN_POINT ( 'NONE',  ( -0.1264236179284866091, -0.0004921259304884456750, 0.1264236179284866091 ) ) ;
#41764=CARTESIAN_POINT ( 'NONE',  ( -0.07405724077823318263, -1.297244094434425010, 0.1787899950787401604 ) ) ;
#41776=CARTESIAN_POINT ( 'NONE',  ( -0.09072478486328348912, -0.09340956239926175020, -0.2330530577653659730 ) ) ;
#41780=CARTESIAN_POINT ( 'NONE',  ( -0.1574803149606300301, -0.02017716524680367163, -0.06523048226347956391 ) ) ;
#41788=CARTESIAN_POINT ( 'NONE',  ( 0.1787899950787401604, -1.101501920985143990, 0.07405724077823318263 ) ) ;
#41790=CARTESIAN_POINT ( 'NONE',  ( 0.1264236179284866091, 0.02411417328210995956, -0.1264236179284866091 ) ) ;
#41794=DIRECTION ( 'NONE',  ( 0.4999999999999998890, 0.000000000000000000, 0.8660254037844388186 ) ) ;
#41798=CARTESIAN_POINT ( 'NONE',  ( -0.1264236179284866091, -0.5615157479777322935, -0.1264236179284866091 ) ) ;
#41801=CARTESIAN_POINT ( 'NONE',  ( 0.1270800023317771588, -1.206736722968872133, 0.1270800023317771588 ) ) ;
#41815=ORIENTED_EDGE ( 'NONE', *, *, #38837, .T. ) ;
#41817=CARTESIAN_POINT ( 'NONE',  ( 2.892866454678787531E-17, -1.740157480207433105, 0.1574803149606299191 ) ) ;
#41822=CARTESIAN_POINT ( 'NONE',  ( 0.07405724077823318263, 0.09055118115612580121, 0.1787899950787401604 ) ) ;
#41829=CARTESIAN_POINT ( 'NONE',  ( -0.1574803149606300301, -0.3745078739082211006, -0.06523048226347956391 ) ) ;
#41830=CARTESIAN_POINT ( 'NONE',  ( 0.1787899950787401604, -1.562992125930488196, 0.07405724077823318263 ) ) ;
#41833=ORIENTED_EDGE ( 'NONE', *, *, #5865, .F. ) ;
#41837=CARTESIAN_POINT ( 'NONE',  ( 0.1580704331077708857, 0.1206688581849416769, -0.006611858888777481270 ) ) ;
#41839=CARTESIAN_POINT ( 'NONE',  ( -1.094772975963752103E-17, -0.5380176690166401654, -0.1787899950787401882 ) ) ;
#41840=CARTESIAN_POINT ( 'NONE',  ( 0.1442972407897856468, -0.08956032687278150939, -0.1319430747994370101 ) ) ;
#41851=CARTESIAN_POINT ( 'NONE',  ( 0.1264236179284866091, -1.516240157426551161, -0.1264236179284866091 ) ) ;
#41856=CARTESIAN_POINT ( 'NONE',  ( 0.1797182628040039087, -0.6875438095830463947, -0.07444174185955065859 ) ) ;
#41861=CARTESIAN_POINT ( 'NONE',  ( 0.1113553986120547346, -0.4852362204724409156, 0.1113553986120547346 ) ) ;
#41873=CARTESIAN_POINT ( 'NONE',  ( -0.1787899950787401604, -0.4704724408911186706, 0.07405724077823318263 ) ) ;
#41874=EDGE_LOOP ( 'NONE', ( #37044, #26977, #10766 ) ) ;
#41879=CARTESIAN_POINT ( 'NONE',  ( 3.284318927891251994E-17, -1.722933070812378009, 0.1787899950787401882 ) ) ;
#41880=CARTESIAN_POINT ( 'NONE',  ( 0.1264236179284866091, -0.8469488188438739629, -0.1264236179284866091 ) ) ;
#41881=CARTESIAN_POINT ( 'NONE',  ( -0.06523048226347956391, -1.334153543307087242, -0.1574803149606300301 ) ) ;
#41888=CARTESIAN_POINT ( 'NONE',  ( 0.06523048226347956391, 0.009350393808314453811, -0.1574803149606300301 ) ) ;
#41898=CARTESIAN_POINT ( 'NONE',  ( -0.1894960330211026833, 0.07859832706092077792, 0.1760274851910419436 ) ) ;
#41902=CARTESIAN_POINT ( 'NONE',  ( 0.09176752663691399581, -0.09842519685039370636, -0.1728335834645769731 ) ) ;
#41904=EDGE_CURVE ( 'NONE', #3164, #2574, #713, .T. ) ;
#41908=CARTESIAN_POINT ( 'NONE',  ( 0.1787899950787401604, -1.011811023568284451, 0.07405724077823318263 ) ) ;
#41909=CARTESIAN_POINT ( 'NONE',  ( 0.1787899950787401882, -1.161909448765133801, -2.189545951927503898E-17 ) ) ;
#41912=CARTESIAN_POINT ( 'NONE',  ( 0.1797182628040039365, -0.4931540458035180707, -2.200913952912460540E-17 ) ) ;
#41913=CARTESIAN_POINT ( 'NONE',  ( -0.1574803149606297803, -1.826279527451528661, 0.06523048226347956391 ) ) ;
#41915=CARTESIAN_POINT ( 'NONE',  ( 0.06523048226347956391, 0.03887795275590551908, -0.1574803149606300301 ) ) ;
#41925=CARTESIAN_POINT ( 'NONE',  ( 0.1264236179284866091, -0.3745078739619845942, -0.1264236179284866091 ) ) ;
#41928=CARTESIAN_POINT ( 'NONE',  ( 0.1787899950787401604, -1.356299212544662014, -0.07405724077823318263 ) ) ;
#41942=CARTESIAN_POINT ( 'NONE',  ( -0.05554372828378579402, -0.07731288306167675983, 0.2533648624690310047 ) ) ;
#41949=CARTESIAN_POINT ( 'NONE',  ( -0.2118463275878102459, -0.09851385012822971854, 0.1047257731708598344 ) ) ;
#41958=CARTESIAN_POINT ( 'NONE',  ( -0.1264236179284866091, -0.5172244093950552069, -0.1264236179284866091 ) ) ;
#41964=CARTESIAN_POINT ( 'NONE',  ( 0.1787899950787401882, -0.7288385826234015097, -2.189545951927503898E-17 ) ) ;
#41967=CARTESIAN_POINT ( 'NONE',  ( -0.07405724077823318263, -0.008982235945774144636, 0.1787899950787401604 ) ) ;
#41968=CARTESIAN_POINT ( 'NONE',  ( -1.094772975963752103E-17, 0.1422244095025824717, -0.1787899950787401882 ) ) ;
#41972=CARTESIAN_POINT ( 'NONE',  ( 0.06523048226347956391, -0.9207677165354321014, 0.1574803149606297803 ) ) ;
#41974=CARTESIAN_POINT ( 'NONE',  ( 0.07444174185955065859, -1.642268219031864707, 0.1797182628040039087 ) ) ;
#41977=CARTESIAN_POINT ( 'NONE',  ( 0.1787899950787401604, -0.3375984251430867999, 0.07405724077823318263 ) ) ;
#41986=CARTESIAN_POINT ( 'NONE',  ( -0.1574803149606300301, -0.8469488187901119680, -0.06523048226347956391 ) ) ;
#41987=CARTESIAN_POINT ( 'NONE',  ( 0.1787899950787401882, 0.09301181107738563936, -2.189545951927503898E-17 ) ) ;
#41998=CARTESIAN_POINT ( 'NONE',  ( 0.07405724077823318263, -1.395669291284819868, -0.1787899950787401604 ) ) ;
#42012=PLANE ( 'NONE',  #22178 ) ;
#42016=CARTESIAN_POINT ( 'NONE',  ( -0.06523048226347956391, -0.1825787400499532531, -0.1574803149606300301 ) ) ;
#42023=CARTESIAN_POINT ( 'NONE',  ( -0.07405724077823318263, -1.150714519410340753, 0.1787899950787401604 ) ) ;
#42025=CARTESIAN_POINT ( 'NONE',  ( 0.1264236179284866091, -0.1038385826234017734, 0.1264236179284866091 ) ) ;
#42035=CARTESIAN_POINT ( 'NONE',  ( 0.1787899950787401882, -0.6550196849856062542, -2.189545951927503898E-17 ) ) ;
#42040=CARTESIAN_POINT ( 'NONE',  ( 0.1797182628040039365, -1.162445384386194824, -2.200913952912460540E-17 ) ) ;
#42047=CARTESIAN_POINT ( 'NONE',  ( -0.01380083870287700763, -0.09697728935039548470, 0.1574803149606300023 ) ) ;
#42048=CARTESIAN_POINT ( 'NONE',  ( 0.1574803149606299191, -0.7460629920184567165, -1.928577636452523993E-17 ) ) ;
#42049=CARTESIAN_POINT ( 'NONE',  ( 0.1787899950787401882, 0.05856299217974772486, -2.189545951927503898E-17 ) ) ;
#42058=CARTESIAN_POINT ( 'NONE',  ( 0.06523048226347956391, -1.644192913278300860, -0.1574803149606300301 ) ) ;
#42063=CARTESIAN_POINT ( 'NONE',  ( -0.07405724077823318263, 0.08562992131360593062, 0.1787899950787401604 ) ) ;
#42071=CARTESIAN_POINT ( 'NONE',  ( 0.1113553986120547346, -0.3868110235145200693, -0.1113553986120547346 ) ) ;
#42072=CARTESIAN_POINT ( 'NONE',  ( -0.07405724077823318263, -1.690944881836001334, 0.1787899950787401604 ) ) ;
#42080=CARTESIAN_POINT ( 'NONE',  ( 0.1787899950787401882, -0.7447105824024665699, -2.189545951927503898E-17 ) ) ;
#42082=CARTESIAN_POINT ( 'NONE',  ( -0.1484669515004454765, -0.08956113575196811283, -0.09387933231569273174 ) ) ;
#42084=ORIENTED_EDGE ( 'NONE', *, *, #7679, .T. ) ;
#42092=CARTESIAN_POINT ( 'NONE',  ( 0.1264236179284866091, -1.437499999946236340, -0.1264236179284866091 ) ) ;
#42096=CARTESIAN_POINT ( 'NONE',  ( 3.301370929368692659E-17, -0.7392170379295019966, 0.1797182628040039365 ) ) ;
#42098=CARTESIAN_POINT ( 'NONE',  ( -0.1574803149606299191, -0.5000000000000000000, 0.000000000000000000 ) ) ;
#42111=CARTESIAN_POINT ( 'NONE',  ( 3.284318927891251994E-17, -0.5812007873478111097, 0.1787899950787401882 ) ) ;
#42117=CARTESIAN_POINT ( 'NONE',  ( 3.284318927891251994E-17, -1.762303149552535642, 0.1787899950787401882 ) ) ;
#42118=CARTESIAN_POINT ( 'NONE',  ( 0.1787899950787401604, -1.090551181048598606, 0.07405724077823318263 ) ) ;
#42119=CARTESIAN_POINT ( 'NONE',  ( -0.1113553986120547346, -1.371062992125984259, -0.1113553986120547346 ) ) ;
#42139=CARTESIAN_POINT ( 'NONE',  ( -0.1711856790334027878, 0.08819060268785008927, 0.1865989729947978293 ) ) ;
#42142=CARTESIAN_POINT ( 'NONE',  ( -1.094772975963752103E-17, -0.3017971965756956476, -0.1787899950787401882 ) ) ;
#42145=CARTESIAN_POINT ( 'NONE',  ( -0.03864956553883512613, -0.09842519685039370636, 0.2227303740875846427 ) ) ;
#42148=ORIENTED_EDGE ( 'NONE', *, *, #44773, .T. ) ;
#42151=CARTESIAN_POINT ( 'NONE',  ( 0.1787899950787401604, -1.051181102308440529, 0.07405724077823318263 ) ) ;
#42152=CARTESIAN_POINT ( 'NONE',  ( 0.1787899950787401604, -1.203740157426551383, 0.07405724077823318263 ) ) ;
#42156=CARTESIAN_POINT ( 'NONE',  ( 0.1270800023317771588, -0.4488627072208409285, -0.1270800023317771588 ) ) ;
#42157=CARTESIAN_POINT ( 'NONE',  ( -0.1574803149606299191, -1.789370078632629868, 0.000000000000000000 ) ) ;
#42159=CARTESIAN_POINT ( 'NONE',  ( 2.892866454678787531E-17, 0.06102362204724409711, 0.1574803149606299191 ) ) ;
#42161=CIRCLE ( 'NONE', #835, 0.1673228346456692994 ) ;
#42170=CARTESIAN_POINT ( 'NONE',  ( 3.284318927891251994E-17, -0.5073818897100158543, 0.1787899950787401882 ) ) ;
#42172=CARTESIAN_POINT ( 'NONE',  ( -0.1264236179284866091, -1.452263779473795369, 0.1264236179284866091 ) ) ;
#42181=CARTESIAN_POINT ( 'NONE',  ( -0.1574803149606300301, -1.240649606191686072, -0.06523048226347956391 ) ) ;
#42185=CARTESIAN_POINT ( 'NONE',  ( 0.1767609453248275564, -0.09842768728010117818, -0.02846602293845313172 ) ) ;
#42197=CARTESIAN_POINT ( 'NONE',  ( -0.2233098565426767657, -0.09851385024739447993, 0.08145678030718524198 ) ) ;
#42204=CARTESIAN_POINT ( 'NONE',  ( 0.1264236179284866091, -1.605931054843411587, -0.1264236179284866091 ) ) ;
#42207=CARTESIAN_POINT ( 'NONE',  ( 0.1787899950787401882, -0.6107283464029291675, -2.189545951927503898E-17 ) ) ;
#42213=CARTESIAN_POINT ( 'NONE',  ( 0.1264236179284866091, -0.2957677164816697180, -0.1264236179284866091 ) ) ;
#42214=CARTESIAN_POINT ( 'NONE',  ( -0.07405724077823318263, -0.7411417322297018107, 0.1787899950787401604 ) ) ;
#42218=CARTESIAN_POINT ( 'NONE',  ( 0.1787899950787401882, 0.04269099240068251894, -2.189545951927503898E-17 ) ) ;
#42219=CARTESIAN_POINT ( 'NONE',  ( 3.284318927891251994E-17, 0.1225393701325037388, 0.1787899950787401882 ) ) ;
#42222=VECTOR ( 'NONE', #46479, 39.37007874015748143 ) ;
#42226=CARTESIAN_POINT ( 'NONE',  ( -0.1574803149606300301, -0.9749015748031498729, -0.06523048226347956391 ) ) ;
#42228=CARTESIAN_POINT ( 'NONE',  ( 0.1797182628040039087, -1.632425699346824466, -0.07444174185955065859 ) ) ;
#42229=CARTESIAN_POINT ( 'NONE',  ( 0.1787899950787401604, -0.3326771653005671237, -0.07405724077823318263 ) ) ;
#42232=CARTESIAN_POINT ( 'NONE',  ( 0.1806410355270341994, 0.08353766247254058863, -0.1811399203779157918 ) ) ;
#42240=CARTESIAN_POINT ( 'NONE',  ( -1.094772975963752103E-17, -0.01525590545804752021, -0.1787899950787401882 ) ) ;
#42241=CARTESIAN_POINT ( 'NONE',  ( 3.284318927891251994E-17, -0.03001968498560657339, 0.1787899950787401882 ) ) ;
#42243=CARTESIAN_POINT ( 'NONE',  ( -1.094772975963752103E-17, -0.9945866141194644738, -0.1787899950787401882 ) ) ;
#42252=CARTESIAN_POINT ( 'NONE',  ( 2.892866454678787531E-17, -1.070866141624756018, 0.1574803149606299191 ) ) ;
#42253=CARTESIAN_POINT ( 'NONE',  ( 0.1787899950787401882, -1.403051181048598384, -2.189545951927503898E-17 ) ) ;
#42261=LINE ( 'NONE', #17101, #28555 ) ;
#42267=CARTESIAN_POINT ( 'NONE',  ( -0.02739131347899105909, -0.09752745740044843625, 0.1550798682808147422 ) ) ;
#42274=CARTESIAN_POINT ( 'NONE',  ( 0.07405724077823318263, -1.067053102087507366, 0.1787899950787401604 ) ) ;
#42276=CARTESIAN_POINT ( 'NONE',  ( 0.1264236179284866091, -0.1825787401037169411, 0.1264236179284866091 ) ) ;
#42277=ORIENTED_EDGE ( 'NONE', *, *, #35776, .F. ) ;
#42278=ORIENTED_EDGE ( 'NONE', *, *, #29231, .F. ) ;
#42285=CARTESIAN_POINT ( 'NONE',  ( -1.094772975963752103E-17, -0.5664370078202519698, -0.1787899950787401882 ) ) ;
#42288=CARTESIAN_POINT ( 'NONE',  ( -0.1270800023317771588, -1.177209163913754075, 0.1270800023317771588 ) ) ;
#42296=EDGE_CURVE ( 'NONE', #47458, #22666, #30124, .T. ) ;
#42300=CARTESIAN_POINT ( 'NONE',  ( -0.1787899950787401604, 0.1151574803687242243, -0.07405724077823318263 ) ) ;
#42311=CARTESIAN_POINT ( 'NONE',  ( -0.1113553986120547346, -1.705708661309795149, 0.1113553986120547346 ) ) ;
#42315=CARTESIAN_POINT ( 'NONE',  ( 0.03837864586585212900, -0.06712557525767723354, 0.2632749781601034789 ) ) ;
#42317=CARTESIAN_POINT ( 'NONE',  ( 0.06523048226347956391, -1.786909448818898571, 0.1574803149606297803 ) ) ;
#42321=CARTESIAN_POINT ( 'NONE',  ( -0.08643384275325982635, 0.09202339627320535453, 0.2355304684854533370 ) ) ;
#42323=CARTESIAN_POINT ( 'NONE',  ( 0.1787899950787401604, -1.681102362150960650, 0.07405724077823318263 ) ) ;
#42328=CARTESIAN_POINT ( 'NONE',  ( 0.1583756834309467398, 0.1213737535021009450, -0.01438113282651966134 ) ) ;
#42330=CARTESIAN_POINT ( 'NONE',  ( 0.07405724077823318263, -0.6733523146859311526, 0.1787899950787401604 ) ) ;
#42332=CARTESIAN_POINT ( 'NONE',  ( -0.1377866315803517872, -0.08956094045033681506, -0.1113219018184753994 ) ) ;
#42346=CARTESIAN_POINT ( 'NONE',  ( 0.1270800023317771588, -0.7638233371421003781, -0.1270800023317771588 ) ) ;
#42347=CARTESIAN_POINT ( 'NONE',  ( 0.2471922904502826812, 0.08811029028641703675, 0.05516800237527588052 ) ) ;
#42351=CARTESIAN_POINT ( 'NONE',  ( 2.892866454678787531E-17, -0.3720472440944881942, 0.1574803149606299191 ) ) ;
#42352=CARTESIAN_POINT ( 'NONE',  ( -0.1439004954719960427, -0.09842519685039366473, 0.08538203236020840137 ) ) ;
#42360=CARTESIAN_POINT ( 'NONE',  ( -0.1574803149606299191, -0.6082677164279055582, 0.000000000000000000 ) ) ;
#42365=CARTESIAN_POINT ( 'NONE',  ( -0.1264236179284866091, -0.5861220471903307860, 0.1264236179284866091 ) ) ;
#42371=CARTESIAN_POINT ( 'NONE',  ( 0.1797182628040039087, 0.09493650537758448194, 0.07444174185955046430 ) ) ;
#42372=CARTESIAN_POINT ( 'NONE',  ( 0.1787899950787401882, -1.127460629867496067, -2.189545951927503898E-17 ) ) ;
#42373=CARTESIAN_POINT ( 'NONE',  ( -0.1113553986120547346, -1.292322834645669438, -0.1113553986120547346 ) ) ;
#42379=CARTESIAN_POINT ( 'NONE',  ( -0.06523048226347956391, -1.348917322727117174, 0.1574803149606297803 ) ) ;
#42382=DIRECTION ( 'NONE',  ( 0.000000000000000000, 0.000000000000000000, 1.000000000000000000 ) ) ;
#42389=CARTESIAN_POINT ( 'NONE',  ( -0.07405724077823318263, -0.2205964091741206001, -0.1787899950787401604 ) ) ;
#42391=CARTESIAN_POINT ( 'NONE',  ( 0.1098058327898338432, -0.09842519685039370636, 0.1888946959883346655 ) ) ;
#42399=CARTESIAN_POINT ( 'NONE',  ( -0.1787899950787401604, -1.297244094434425010, 0.07405724077823318263 ) ) ;
#42401=CARTESIAN_POINT ( 'NONE',  ( -0.1797182628040039087, -0.4316382977720212843, 0.07444174185955065859 ) ) ;
#42402=CARTESIAN_POINT ( 'NONE',  ( 0.1113553986120547346, -1.774606299105070839, 0.1113553986120547346 ) ) ;
#42406=CARTESIAN_POINT ( 'NONE',  ( 0.06523048226347956391, -0.05462598425196847629, 0.1574803149606297803 ) ) ;
#42412=CARTESIAN_POINT ( 'NONE',  ( -0.1787899950787401882, -0.5565944881352126172, 0.000000000000000000 ) ) ;
#42413=CARTESIAN_POINT ( 'NONE',  ( 3.284318927891251994E-17, -1.368602362150960650, 0.1787899950787401882 ) ) ;
#42430=CARTESIAN_POINT ( 'NONE',  ( 0.2074133033502960355, -0.09851384765663445675, 0.004766324057523401575 ) ) ;
#42437=CARTESIAN_POINT ( 'NONE',  ( -1.094772975963752103E-17, -1.640379873741049321, -0.1787899950787401882 ) ) ;
#42439=CARTESIAN_POINT ( 'NONE',  ( -0.1787899950787401882, -0.5123031495525355306, 0.000000000000000000 ) ) ;
#42443=CARTESIAN_POINT ( 'NONE',  ( -0.07405724077823318263, -0.2736220471903310081, 0.1787899950787401604 ) ) ;
#42445=CARTESIAN_POINT ( 'NONE',  ( 0.07405724077823318263, -0.7755905511273385455, 0.1787899950787401604 ) ) ;
#42450=CARTESIAN_POINT ( 'NONE',  ( -0.07405724077823318263, 0.05499414200698173744, -0.1787899950787401604 ) ) ;
#42451=CARTESIAN_POINT ( 'NONE',  ( -0.1264236179284866091, 0.07824803154982658271, 0.1264236179284866091 ) ) ;
#42453=CARTESIAN_POINT ( 'NONE',  ( -0.02321135729119747776, -0.09842519685039372024, 0.1582298369811388494 ) ) ;
#42455=ADVANCED_FACE ( 'NONE', ( #30650 ), #35589, .T. ) ;
#42458=CARTESIAN_POINT ( 'NONE',  ( -0.06523048226347956391, -0.8617125984251972071, -0.1574803149606300301 ) ) ;
#42460=CARTESIAN_POINT ( 'NONE',  ( 0.1270800023317771588, -1.639807589110604313, 0.1270800023317771588 ) ) ;
#42463=CARTESIAN_POINT ( 'NONE',  ( -0.1787899950787401604, -0.3966535432533230265, -0.07405724077823318263 ) ) ;
#42472=CARTESIAN_POINT ( 'NONE',  ( 0.1787899950787401882, -0.06446850388324429360, -2.189545951927503898E-17 ) ) ;
#42474=CARTESIAN_POINT ( 'NONE',  ( -0.1264236179284866091, -0.8715551180564724554, -0.1264236179284866091 ) ) ;
#42500=CARTESIAN_POINT ( 'NONE',  ( -0.07405724077823318263, -1.190084598150498607, 0.1787899950787401604 ) ) ;
#42502=CARTESIAN_POINT ( 'NONE',  ( 0.1787899950787401882, -0.09891732278088229136, -2.189545951927503898E-17 ) ) ;
#42511=CARTESIAN_POINT ( 'NONE',  ( -0.07405724077823318263, -0.7214566928596228834, -0.1787899950787401604 ) ) ;
#42516=CARTESIAN_POINT ( 'NONE',  ( -0.1797182628040039087, -1.223961132417690889, -0.07444174185955065859 ) ) ;
#42537=CARTESIAN_POINT ( 'NONE',  ( 0.1787899950787401604, 0.05610236225848785896, 0.07405724077823318263 ) ) ;
#42546=CARTESIAN_POINT ( 'NONE',  ( 2.892866454678787531E-17, -0.4015748030420787651, 0.1574803149606299191 ) ) ;
#42547=CARTESIAN_POINT ( 'NONE',  ( -0.07405724077823318263, -1.626968503883244876, -0.1787899950787401604 ) ) ;
#42554=CARTESIAN_POINT ( 'NONE',  ( 0.1787899950787401604, -0.7028798737410506536, -0.07405724077823318263 ) ) ;
#42556=CARTESIAN_POINT ( 'NONE',  ( 0.09025693572801693487, -0.08956069895912480150, -0.1695530491970364262 ) ) ;
#42559=CARTESIAN_POINT ( 'NONE',  ( 0.06523048226347956391, 0.06348425196850393526, 0.1574803149606297803 ) ) ;
#42568=CARTESIAN_POINT ( 'NONE',  ( -0.1797182628040039365, -0.6703194001342264174, 0.000000000000000000 ) ) ;
#42571=CARTESIAN_POINT ( 'NONE',  ( 0.1113553986120547346, -0.3572834645669291098, -0.1113553986120547346 ) ) ;
#42579=CARTESIAN_POINT ( 'NONE',  ( 0.1113553986120547346, -0.5836614172153071767, -0.1113553986120547346 ) ) ;
#42581=CARTESIAN_POINT ( 'NONE',  ( 0.07405724077823318263, -0.5246062991588343882, -0.1787899950787401604 ) ) ;
#42587=CARTESIAN_POINT ( 'NONE',  ( -8.354793841626791791E-17, 0.03219022224904082713, -0.2854330708661417804 ) ) ;
#42589=CARTESIAN_POINT ( 'NONE',  ( -0.1797182628040039087, 0.04080264710986784837, 0.07444174185955065859 ) ) ;
#42590=CARTESIAN_POINT ( 'NONE',  ( -0.1787899950787401604, -1.031496062938363822, -0.07405724077823318263 ) ) ;
#42591=CARTESIAN_POINT ( 'NONE',  ( -0.1574803149606300301, -1.329232283464566011, -0.06523048226347956391 ) ) ;
#42599=CARTESIAN_POINT ( 'NONE',  ( 0.1574803149606300301, -1.452263779420031709, -0.06523048226347956391 ) ) ;
#42610=CARTESIAN_POINT ( 'NONE',  ( 0.1787899950787401882, -0.2328995587804200962, -2.189545951927503898E-17 ) ) ;
#42612=CARTESIAN_POINT ( 'NONE',  ( 0.1762049892238537474, -0.09842519685039370636, -0.09843609369557973499 ) ) ;
#42620=CARTESIAN_POINT ( 'NONE',  ( 0.1264236179284866091, -1.083169291284818980, -0.1264236179284866091 ) ) ;
#42621=CARTESIAN_POINT ( 'NONE',  ( 0.1264236179284866091, -1.196358267662771757, -0.1264236179284866091 ) ) ;
#42625=CARTESIAN_POINT ( 'NONE',  ( 3.301370929368692659E-17, -0.5029965654885574233, 0.1797182628040039365 ) ) ;
#42629=CARTESIAN_POINT ( 'NONE',  ( -0.1113553986120547346, 0.05610236220472441387, 0.1113553986120547346 ) ) ;
#42636=CARTESIAN_POINT ( 'NONE',  ( -0.07405724077823318263, -0.6673228345919050009, 0.1787899950787401604 ) ) ;
#42637=CARTESIAN_POINT ( 'NONE',  ( -0.1787899950787401604, -1.336614173174582865, 0.07405724077823318263 ) ) ;
#42648=CARTESIAN_POINT ( 'NONE',  ( 0.1306058198804243842, -0.09842711666118027225, -0.1221223300366590520 ) ) ;
#42651=CARTESIAN_POINT ( 'NONE',  ( 0.1916485431825860897, -0.07731288306172690028, 0.1747847109491888207 ) ) ;
#42658=CARTESIAN_POINT ( 'NONE',  ( 0.1954853181098232251, -0.09851384548657264595, 0.08125050196056771146 ) ) ;
#42661=CARTESIAN_POINT ( 'NONE',  ( -0.1787899950787401604, -1.549336566654435865, 0.07405724077823318263 ) ) ;
#42663=CARTESIAN_POINT ( 'NONE',  ( 0.07405724077823318263, -0.5393700786863945273, 0.1787899950787401604 ) ) ;
#42670=CARTESIAN_POINT ( 'NONE',  ( -0.1264236179284866091, -0.3154527558517483676, 0.1264236179284866091 ) ) ;
#42671=CARTESIAN_POINT ( 'NONE',  ( 3.284318927891251994E-17, -0.7386811023084409733, 0.1787899950787401882 ) ) ;
#42675=CARTESIAN_POINT ( 'NONE',  ( 0.1787899950787401604, 0.005781543581784898134, -0.07405724077823318263 ) ) ;
#42676=CARTESIAN_POINT ( 'NONE',  ( 0.1787899950787401604, 0.01673228351833045899, -0.07405724077823318263 ) ) ;
#42680=CARTESIAN_POINT ( 'NONE',  ( 0.1574803149606300301, -0.8764763779527571241, 0.06523048226347956391 ) ) ;
#42682=CARTESIAN_POINT ( 'NONE',  ( 0.1797182628040039087, -1.716087116669659629, 0.07444174185955046430 ) ) ;
#42684=CARTESIAN_POINT ( 'NONE',  ( 0.1898978525284559515, 0.07836113345104910033, -0.1757954945903058008 ) ) ;
#42687=DIRECTION ( 'NONE',  ( 0.000000000000000000, 0.000000000000000000, 1.000000000000000000 ) ) ;
#42689=CARTESIAN_POINT ( 'NONE',  ( 2.892866454678787531E-17, -0.9133858266641260437, 0.1574803149606299191 ) ) ;
#42690=CARTESIAN_POINT ( 'NONE',  ( -0.1787899950787401882, -0.1628937007336379861, 0.000000000000000000 ) ) ;
#42692=CARTESIAN_POINT ( 'NONE',  ( 0.1787899950787401604, -0.9625984251430860228, -0.07405724077823318263 ) ) ;
#42715=CARTESIAN_POINT ( 'NONE',  ( -0.1264236179284866091, 0.1176181102899840625, 0.1264236179284866091 ) ) ;
#42721=CARTESIAN_POINT ( 'NONE',  ( -0.07405724077823318263, -1.086738141457586515, -0.1787899950787401604 ) ) ;
#42723=CARTESIAN_POINT ( 'NONE',  ( 0.1787899950787401882, -0.05954724404072461036, -2.189545951927503898E-17 ) ) ;
#42730=CARTESIAN_POINT ( 'NONE',  ( 0.1797182628040039365, -0.1781934158822582603, -2.200913952912460540E-17 ) ) ;
#42733=CARTESIAN_POINT ( 'NONE',  ( 0.1797182628040039087, -1.278094990685408439, -0.07444174185955065859 ) ) ;
#42742=CARTESIAN_POINT ( 'NONE',  ( 0.1574803149606300301, -0.7829724408373558431, -0.06523048226347956391 ) ) ;
#42752=ORIENTED_EDGE ( 'NONE', *, *, #37764, .F. ) ;
#42755=CARTESIAN_POINT ( 'NONE',  ( -0.1787899950787401604, 0.04133858273092887170, 0.07405724077823318263 ) ) ;
#42761=CARTESIAN_POINT ( 'NONE',  ( 0.1627568843983490665, 0.09133345722617872142, 0.1914653398462901890 ) ) ;
#42766=CARTESIAN_POINT ( 'NONE',  ( -0.1574803149606300301, -0.4138779526483781224, -0.06523048226347956391 ) ) ;
#42767=CARTESIAN_POINT ( 'NONE',  ( 3.284318927891251994E-17, -1.767224409395055318, 0.1787899950787401882 ) ) ;
#42772=EDGE_CURVE ( 'NONE', #30178, #6678, #26091, .T. ) ;
#42775=CARTESIAN_POINT ( 'NONE',  ( 0.1787899950787401604, -0.7078011335835699969, 0.07405724077823318263 ) ) ;
#42779=CARTESIAN_POINT ( 'NONE',  ( -0.07117121207836790697, -0.08956324299011318713, 0.1404802767937309016 ) ) ;
#42780=ORIENTED_EDGE ( 'NONE', *, *, #5999, .F. ) ;
#42794=CARTESIAN_POINT ( 'NONE',  ( -0.1574803149606300301, -0.6599409448818898127, -0.06523048226347956391 ) ) ;
#42795=CARTESIAN_POINT ( 'NONE',  ( -0.1639265925754282704, 0.1264995129648254779, 0.007850818260147569144 ) ) ;
#42806=CARTESIAN_POINT ( 'NONE',  ( -0.1636338509590271328, -0.08956016023378124413, -0.05621478700804145856 ) ) ;
#42807=CARTESIAN_POINT ( 'NONE',  ( -0.1787899950787401604, -0.6328740156942683770, -0.07405724077823318263 ) ) ;
#42815=CARTESIAN_POINT ( 'NONE',  ( 0.1797182628040039087, 0.06048768647994660214, -0.07444174185955065859 ) ) ;
#42816=CARTESIAN_POINT ( 'NONE',  ( -1.094772975963752103E-17, -1.117618110182456714, -0.1787899950787401882 ) ) ;
#42817=CARTESIAN_POINT ( 'NONE',  ( -0.06523048226347956391, -1.555610236220473785, 0.1574803149606297803 ) ) ;
#42824=CARTESIAN_POINT ( 'NONE',  ( -0.06523048226347956391, -1.442421259734993244, -0.1574803149606300301 ) ) ;
#42832=CARTESIAN_POINT ( 'NONE',  ( -0.2471922904502827090, 0.09275221067063772751, 0.04038095640780218348 ) ) ;
#42835=CARTESIAN_POINT ( 'NONE',  ( 0.07968303789223217526, -0.08956740676322874628, -0.2394271090157727711 ) ) ;
#42838=CARTESIAN_POINT ( 'NONE',  ( 0.1787899950787401604, -0.3141003461819947828, 0.07405724077823318263 ) ) ;
#42845=ORIENTED_EDGE ( 'NONE', *, *, #21093, .T. ) ;
#42847=CARTESIAN_POINT ( 'NONE',  ( -0.1787899950787401604, -1.105314960576158301, 0.07405724077823318263 ) ) ;
#42848=B_SPLINE_CURVE_WITH_KNOTS ( 'NONE', 3,
 ( #28691, #36084, #3243, #17871, #32514, #47098, #28933, #43496, #10704, #25310, #44430, #9149, #22406, #37031, #27157, #11402, #40596, #16356, #26268, #15009, #22161 ),
 .UNSPECIFIED., .F., .F.,
 ( 4, 2, 1, 1, 2, 2, 2, 1, 1, 1, 2, 2, 4 ),
 ( 0.000000000000000000, 0.1249999999999968359, 0.1874999999999953648, 0.2187499999999947264, 0.2343749999999944766, 0.2499999999999942268, 0.3749999999999941713, 0.4374999999999943379, 0.4687499999999944489, 0.4843749999999945044, 0.4921874999999945599, 0.4999999999999945599, 1.000000000000000000 ),
 .UNSPECIFIED. ) ;
#42849=CARTESIAN_POINT ( 'NONE',  ( -0.1787899950787401882, -1.299704724355684959, 0.000000000000000000 ) ) ;
#42854=CARTESIAN_POINT ( 'NONE',  ( 2.892866454678787531E-17, -0.1751968503937007815, 0.1574803149606299191 ) ) ;
#42857=CARTESIAN_POINT ( 'NONE',  ( -0.1113553986120547346, -0.06200787401574803237, 0.1113553986120547346 ) ) ;
#42866=CARTESIAN_POINT ( 'NONE',  ( 3.284318927891251994E-17, -0.5861220471903307860, 0.1787899950787401882 ) ) ;
#42869=CARTESIAN_POINT ( 'NONE',  ( 0.07405724077823318263, -1.405511810969858999, 0.1787899950787401604 ) ) ;
#42876=EDGE_LOOP ( 'NONE', ( #38512, #24672, #29314, #39904 ) ) ;
#42880=CARTESIAN_POINT ( 'NONE',  ( 0.1727868965068283524, -0.09842808818411986904, -0.04689813055546866727 ) ) ;
#42887=CARTESIAN_POINT ( 'NONE',  ( 0.1113553986120547346, -0.1604330707586147375, 0.1113553986120547346 ) ) ;
#42893=CARTESIAN_POINT ( 'NONE',  ( 0.1908917291238539371, -0.09851384365687540501, -0.07079149662741023030 ) ) ;
#42899=CARTESIAN_POINT ( 'NONE',  ( 0.1787899950787401882, -1.689592472166246306, -2.189545951927503898E-17 ) ) ;
#42901=CARTESIAN_POINT ( 'NONE',  ( -0.1787899950787401882, -0.5516732282926929409, 0.000000000000000000 ) ) ;
#42907=CARTESIAN_POINT ( 'NONE',  ( -0.1787899950787401882, -0.2810039369541106336, 0.000000000000000000 ) ) ;
#42908=CARTESIAN_POINT ( 'NONE',  ( 3.284318927891251994E-17, -0.7780511810485984947, 0.1787899950787401882 ) ) ;
#42914=CARTESIAN_POINT ( 'NONE',  ( -0.1787899950787401882, -0.01636412570955368337, 0.000000000000000000 ) ) ;
#42919=CARTESIAN_POINT ( 'NONE',  ( 0.1113553986120547346, -0.9183070866141731514, 0.1113553986120547346 ) ) ;
#42921=CARTESIAN_POINT ( 'NONE',  ( 0.1797182628040039087, -1.794827274149976004, 0.07444174185955046430 ) ) ;
#42930=CARTESIAN_POINT ( 'NONE',  ( -0.2090839795233657428, -0.06563552548624972116, -0.1647146447860223517 ) ) ;
#42933=CARTESIAN_POINT ( 'NONE',  ( -0.07405724077823318263, -0.09153543301710270752, -0.1787899950787401604 ) ) ;
#42935=CARTESIAN_POINT ( 'NONE',  ( 0.1787899950787401882, -0.8863188975840314843, -2.189545951927503898E-17 ) ) ;
#42958=CARTESIAN_POINT ( 'NONE',  ( -0.1264236179284866091, -0.04970472435568527164, -0.1264236179284866091 ) ) ;
#42964=CARTESIAN_POINT ( 'NONE',  ( -0.07405724077823318263, -1.244218456418216601, -0.1787899950787401604 ) ) ;
#42966=CARTESIAN_POINT ( 'NONE',  ( 0.1264236179284866091, -0.1333661416785200671, -0.1264236179284866091 ) ) ;
#42975=CARTESIAN_POINT ( 'NONE',  ( 0.07405724077823318263, -1.410433070812377565, 0.1787899950787401604 ) ) ;
#42979=CARTESIAN_POINT ( 'NONE',  ( -0.1797182628040039087, -1.258409951315329289, 0.07444174185955065859 ) ) ;
#43002=MECHANICAL_DESIGN_GEOMETRIC_PRESENTATION_REPRESENTATION('',(#22360),#33854);
#43005=CARTESIAN_POINT ( 'NONE',  ( -0.07405724077823318263, -0.04724409443442544737, -0.1787899950787401604 ) ) ;
#43009=CARTESIAN_POINT ( 'NONE',  ( 0.1465299180647062771, 0.09658349877441903264, 0.2008339832271497927 ) ) ;
#43015=CARTESIAN_POINT ( 'NONE',  ( 0.1574803149606300301, -0.3892716534357800184, -0.06523048226347956391 ) ) ;
#43016=CARTESIAN_POINT ( 'NONE',  ( 3.284318927891251994E-17, -1.649114173174582643, 0.1787899950787401882 ) ) ;
#43025=CARTESIAN_POINT ( 'NONE',  ( -0.07405724077823318263, -0.6389034957882946397, 0.1787899950787401604 ) ) ;
#43028=CARTESIAN_POINT ( 'NONE',  ( -0.1528862059369570925, -0.08956163382569545806, 0.06277908432128326277 ) ) ;
#43043=CARTESIAN_POINT ( 'NONE',  ( 0.07444174185955065859, -0.8154965654885567572, 0.1797182628040039087 ) ) ;
#43047=CARTESIAN_POINT ( 'NONE',  ( 0.1113553986120547346, -0.6427165354330708347, 0.1113553986120547346 ) ) ;
#43058=CARTESIAN_POINT ( 'NONE',  ( -0.1264236179284866091, -0.6254921259304881964, 0.1264236179284866091 ) ) ;
#43067=CARTESIAN_POINT ( 'NONE',  ( 0.1264236179284866091, -1.796751968450173376, 0.1264236179284866091 ) ) ;
#43068=CARTESIAN_POINT ( 'NONE',  ( 0.1264236179284866091, -1.093011810969858333, 0.1264236179284866091 ) ) ;
#43069=CARTESIAN_POINT ( 'NONE',  ( -0.06523048226347956391, -1.594980314960629419, 0.1574803149606297803 ) ) ;
#43076=CARTESIAN_POINT ( 'NONE',  ( 2.892866454678787531E-17, -1.425196850286173156, 0.1574803149606299191 ) ) ;
#43089=CARTESIAN_POINT ( 'NONE',  ( 0.07405724077823318263, -0.2009113698040420337, 0.1787899950787401604 ) ) ;
#43097=CARTESIAN_POINT ( 'NONE',  ( -0.1264236179284866091, -1.142224409395055096, 0.1264236179284866091 ) ) ;
#43098=CARTESIAN_POINT ( 'NONE',  ( 0.1787899950787401604, -1.316929133804503937, -0.07405724077823318263 ) ) ;
#43103=CARTESIAN_POINT ( 'NONE',  ( 0.06523048226347956391, -0.2121062992125984648, 0.1574803149606297803 ) ) ;
#43119=CARTESIAN_POINT ( 'NONE',  ( -0.1113553986120547346, -1.508858267609007653, 0.1113553986120547346 ) ) ;
#43120=CARTESIAN_POINT ( 'NONE',  ( -1.094772975963752103E-17, -0.5664370078202519698, -0.1787899950787401882 ) ) ;
#43121=CARTESIAN_POINT ( 'NONE',  ( 2.892866454678787531E-17, -1.041338582677165503, 0.1574803149606299191 ) ) ;
#43126=VECTOR ( 'NONE', #46759, 39.37007874015748143 ) ;
#43137=CARTESIAN_POINT ( 'NONE',  ( 2.892866454678787531E-17, -0.2047244093412921295, 0.1574803149606299191 ) ) ;
#43151=CARTESIAN_POINT ( 'NONE',  ( -0.1787899950787401604, -0.2834645668753703052, -0.07405724077823318263 ) ) ;
#43152=CARTESIAN_POINT ( 'NONE',  ( 0.1787899950787401882, -0.9256889763241890057, -2.189545951927503898E-17 ) ) ;
#43154=CARTESIAN_POINT ( 'NONE',  ( -0.2471922904502826812, -0.03219022224904098672, -0.1427165354330708902 ) ) ;
#43157=CIRCLE ( 'NONE', #43928, 0.01968503937007875723 ) ;
#43158=CARTESIAN_POINT ( 'NONE',  ( 0.1787899950787401604, -0.07295861389853010304, -0.07405724077823318263 ) ) ;
#43159=CARTESIAN_POINT ( 'NONE',  ( 0.1787899950787401604, -0.2588582676627719792, 0.07405724077823318263 ) ) ;
#43160=CARTESIAN_POINT ( 'NONE',  ( -0.07405724077823318263, 0.06594488194352733645, -0.1787899950787401604 ) ) ;
#43161=CARTESIAN_POINT ( 'NONE',  ( 0.01656181348484438501, -0.09842519685039362309, 0.1616518427886418363 ) ) ;
#43169=CARTESIAN_POINT ( 'NONE',  ( -1.100456976456230270E-17, -1.743154045803517738, -0.1797182628040039365 ) ) ;
#43177=CARTESIAN_POINT ( 'NONE',  ( 0.07405724077823318263, -0.1899606298674962612, 0.1787899950787401604 ) ) ;
#43179=CARTESIAN_POINT ( 'NONE',  ( 0.1264236179284866091, -1.156988188922614125, -0.1264236179284866091 ) ) ;
#43199=CARTESIAN_POINT ( 'NONE',  ( -0.1787899950787401604, -0.007874015694267974541, -0.07405724077823318263 ) ) ;
#43202=CARTESIAN_POINT ( 'NONE',  ( -0.2471922904502826812, 0.09842519685039370636, 5.914624404477007554E-17 ) ) ;
#43204=CARTESIAN_POINT ( 'NONE',  ( -0.1787899950787401604, -1.352486172953647925, 0.07405724077823318263 ) ) ;
#43206=CARTESIAN_POINT ( 'NONE',  ( 0.1787899950787401604, -0.2194881889226144023, 0.07405724077823318263 ) ) ;
#43211=VERTEX_POINT ( 'NONE', #20306 ) ;
#43214=CARTESIAN_POINT ( 'NONE',  ( -0.2471922466704931376, -0.08138981793828348188, 0.07067796049273157577 ) ) ;
#43220=CARTESIAN_POINT ( 'NONE',  ( 0.1787899950787401882, -1.442421259788756016, -2.189545951927503898E-17 ) ) ;
#43221=CARTESIAN_POINT ( 'NONE',  ( -0.1787899950787401882, -0.7928149605761574126, 0.000000000000000000 ) ) ;
#43225=CARTESIAN_POINT ( 'NONE',  ( 3.301370929368692659E-17, -1.290398140291706630, 0.1797182628040039365 ) ) ;
#43237=CARTESIAN_POINT ( 'NONE',  ( 0.1264236179284866091, -0.01525590545804753929, -0.1264236179284866091 ) ) ;
#43255=CARTESIAN_POINT ( 'NONE',  ( 0.1264236179284866091, -0.02509842514308689362, 0.1264236179284866091 ) ) ;
#43256=VERTEX_POINT ( 'NONE', #8811 ) ;
#43263=CARTESIAN_POINT ( 'NONE',  ( 0.07405724077823318263, -1.789370078686394194, -0.1787899950787401604 ) ) ;
#43275=CARTESIAN_POINT ( 'NONE',  ( 0.1264236179284866091, -0.7791594013001044150, -0.1264236179284866091 ) ) ;
#43277=CARTESIAN_POINT ( 'NONE',  ( 0.05390907504427756153, -0.08956249738940257055, 0.1385839714854027738 ) ) ;
#43278=CARTESIAN_POINT ( 'NONE',  ( -0.02421810057410377776, -0.08754923116810497952, 0.1560975693771988193 ) ) ;
#43291=CARTESIAN_POINT ( 'NONE',  ( -0.1797182628040039087, -0.7908902662759585978, -0.07444174185955065859 ) ) ;
#43295=CARTESIAN_POINT ( 'NONE',  ( 0.06523048226347956391, -0.5664370078740157410, 0.1574803149606297803 ) ) ;
#43296=CARTESIAN_POINT ( 'NONE',  ( -0.08791145637253013068, 0.1224054518956866344, -0.1337190540265945915 ) ) ;
#43305=CARTESIAN_POINT ( 'NONE',  ( 0.2471922904502826812, -0.09842519685039370636, -0.1427165354330708902 ) ) ;
#43310=CARTESIAN_POINT ( 'NONE',  ( 0.1270800023317771588, 0.1023183951413639964, -0.1270800023317771588 ) ) ;
#43311=CARTESIAN_POINT ( 'NONE',  ( 0.1787899950787401882, -1.166830708607653477, -2.189545951927503898E-17 ) ) ;
#43312=CARTESIAN_POINT ( 'NONE',  ( 2.892866454678787531E-17, -1.513779527559055094, 0.1574803149606299191 ) ) ;
#43319=CARTESIAN_POINT ( 'NONE',  ( -0.1113553986120547346, -1.400590551073574774, -0.1113553986120547346 ) ) ;
#43328=CARTESIAN_POINT ( 'NONE',  ( -0.2471922904502827090, 0.09255273792768342611, 0.04108768875596389286 ) ) ;
#43332=CARTESIAN_POINT ( 'NONE',  ( 3.284318927891251994E-17, -0.4395924721662464729, 0.1787899950787401882 ) ) ;
#43333=CARTESIAN_POINT ( 'NONE',  ( -0.09634625429846278843, -0.09842519685039370636, -0.1571995980677732274 ) ) ;
#43335=DIRECTION ( 'NONE',  ( 0.000000000000000000, 0.000000000000000000, 1.000000000000000000 ) ) ;
#43342=CARTESIAN_POINT ( 'NONE',  ( -0.1787899950787401604, -1.228346456639149542, -0.07405724077823318263 ) ) ;
#43343=CARTESIAN_POINT ( 'NONE',  ( 0.1264236179284866091, -1.393208661363559031, -0.1264236179284866091 ) ) ;
#43348=CARTESIAN_POINT ( 'NONE',  ( 2.892866454678787531E-17, -0.09645669291338582196, 0.1574803149606299191 ) ) ;
#43360=CARTESIAN_POINT ( 'NONE',  ( 0.1574803149606300301, -1.491633858160189785, -0.06523048226347956391 ) ) ;
#43361=CARTESIAN_POINT ( 'NONE',  ( -0.1787899950787401604, -0.5147637794737950356, 0.07405724077823318263 ) ) ;
#43362=CARTESIAN_POINT ( 'NONE',  ( 0.1574803149606300301, -1.029035433070865535, -0.06523048226347956391 ) ) ;
#43377=CARTESIAN_POINT ( 'NONE',  ( 0.06523048226347956391, -0.08415354319955967166, 0.1574803149606297803 ) ) ;
#43380=CARTESIAN_POINT ( 'NONE',  ( -0.1113553986120547346, -0.1702755904436539236, 0.1113553986120547346 ) ) ;
#43387=CARTESIAN_POINT ( 'NONE',  ( -1.094772975963752103E-17, -1.758490109961521775, -0.1787899950787401882 ) ) ;
#43392=CARTESIAN_POINT ( 'NONE',  ( 0.1264236179284866091, -0.9699803149068660924, 0.1264236179284866091 ) ) ;
#43397=CARTESIAN_POINT ( 'NONE',  ( -0.1787899950787401882, -0.1344743619300261817, 0.000000000000000000 ) ) ;
#43398=CARTESIAN_POINT ( 'NONE',  ( -0.07405724077823318263, -0.3080708660879689087, 0.1787899950787401604 ) ) ;
#43399=CARTESIAN_POINT ( 'NONE',  ( -0.1787899950787401882, -0.005413385773008132923, 0.000000000000000000 ) ) ;
#43400=CARTESIAN_POINT ( 'NONE',  ( 0.2471920410536352364, -0.09140649424452929050, -0.04498895533762308635 ) ) ;
#43406=CARTESIAN_POINT ( 'NONE',  ( 0.1270800023317771588, -1.679177667850761724, 0.1270800023317771588 ) ) ;
#43415=CARTESIAN_POINT ( 'NONE',  ( -0.1574803149606300301, -0.9256889762704257896, -0.06523048226347956391 ) ) ;
#43418=CARTESIAN_POINT ( 'NONE',  ( -0.1787899950787401882, -1.024114173174582643, 0.000000000000000000 ) ) ;
#43439=CARTESIAN_POINT ( 'NONE',  ( -0.1787899950787401882, -0.005413385773008132923, 0.000000000000000000 ) ) ;
#43449=CARTESIAN_POINT ( 'NONE',  ( 0.1787899950787401604, -1.254060976103255065, -0.07405724077823318263 ) ) ;
#43451=CARTESIAN_POINT ( 'NONE',  ( -0.1787899950787401882, -0.2760826771115909573, 0.000000000000000000 ) ) ;
#43457=CARTESIAN_POINT ( 'NONE',  ( -0.1264236179284866091, -1.575295275536787276, 0.1264236179284866091 ) ) ;
#43458=CARTESIAN_POINT ( 'NONE',  ( -0.1787899950787401604, -0.7509842519147402751, 0.07405724077823318263 ) ) ;
#43462=CARTESIAN_POINT ( 'NONE',  ( -0.1270800023317771588, -1.255949321394068674, 0.1270800023317771588 ) ) ;
#43490=CARTESIAN_POINT ( 'NONE',  ( -1.094772975963752103E-17, -0.01033464561552785432, -0.1787899950787401882 ) ) ;
#43495=CARTESIAN_POINT ( 'NONE',  ( 0.2064293380533964994, 0.06762482675899135487, 0.1662510369723770864 ) ) ;
#43496=CARTESIAN_POINT ( 'NONE',  ( 0.1564674760228476069, -0.09340956239926176408, -0.1950964973271320235 ) ) ;
#43499=CARTESIAN_POINT ( 'NONE',  ( 0.06523048226347956391, 0.1126968505012277688, 0.1574803149606297803 ) ) ;
#43508=CARTESIAN_POINT ( 'NONE',  ( -0.1787899950787401882, -0.8431357792528602069, 0.000000000000000000 ) ) ;
#43510=CARTESIAN_POINT ( 'NONE',  ( 0.06711304729538268565, -0.08956252386023248746, 0.1311275629080100313 ) ) ;
#43516=AXIS2_PLACEMENT_3D ( 'NONE', #18866, #44491, #29716 ) ;
#43521=CARTESIAN_POINT ( 'NONE',  ( -0.1797182628040039087, -0.8647091639137531871, 0.07444174185955065859 ) ) ;
#43525=CARTESIAN_POINT ( 'NONE',  ( 0.1574803149606300301, -0.5172244094488184230, -0.06523048226347956391 ) ) ;
#43526=CARTESIAN_POINT ( 'NONE',  ( -0.1634885253152291440, 0.1261140749709542819, -0.008880672301011263703 ) ) ;
#43527=ORIENTED_EDGE ( 'NONE', *, *, #32939, .T. ) ;
#43536=CARTESIAN_POINT ( 'NONE',  ( 0.1264236179284866091, -0.6451771653005667906, -0.1264236179284866091 ) ) ;
#43545=CARTESIAN_POINT ( 'NONE',  ( 0.1787899950787401604, -1.164370078686393306, -0.07405724077823318263 ) ) ;
#43546=CARTESIAN_POINT ( 'NONE',  ( -0.06523048226347956391, -1.531003937007875182, -0.1574803149606300301 ) ) ;
#43554=CARTESIAN_POINT ( 'NONE',  ( 0.1787899950787401604, -1.405511810969858999, 0.07405724077823318263 ) ) ;
#43563=CARTESIAN_POINT ( 'NONE',  ( 0.1787899950787401882, -0.4691200312213645862, -2.189545951927503898E-17 ) ) ;
#43564=CARTESIAN_POINT ( 'NONE',  ( -0.09424215950663268615, -0.09842519685039370636, 0.1330654084077543264 ) ) ;
#43572=CARTESIAN_POINT ( 'NONE',  ( -0.1264236179284866091, -1.230807086560409269, -0.1264236179284866091 ) ) ;
#43574=CARTESIAN_POINT ( 'NONE',  ( 0.1787899950787401604, -1.395669291284819868, -0.07405724077823318263 ) ) ;
#43577=CARTESIAN_POINT ( 'NONE',  ( -1.100456976456230270E-17, -0.6014217623389507272, -0.1797182628040039365 ) ) ;
#43581=CARTESIAN_POINT ( 'NONE',  ( 0.1113553986120547346, -0.1702755905511811052, 0.1113553986120547346 ) ) ;
#43597=CARTESIAN_POINT ( 'NONE',  ( -0.1113553986120547346, -1.558070866034206858, -0.1113553986120547346 ) ) ;
#43598=CARTESIAN_POINT ( 'NONE',  ( 0.1787899950787401604, -0.7362204723871804690, 0.07405724077823318263 ) ) ;
#43600=CARTESIAN_POINT ( 'NONE',  ( -0.1574803149606297803, -1.127460629921260837, 0.06523048226347956391 ) ) ;
#43615=CARTESIAN_POINT ( 'NONE',  ( 2.892866454678787531E-17, -0.08661417312081949593, 0.1574803149606299191 ) ) ;
#43617=CARTESIAN_POINT ( 'NONE',  ( -9.642888182262618425E-18, -0.2637795274515279398, -0.1574803149606299191 ) ) ;
#43624=CARTESIAN_POINT ( 'NONE',  ( 0.1101484706250415307, -0.09851384295070100827, -0.1631889973867482468 ) ) ;
#43627=CARTESIAN_POINT ( 'NONE',  ( 0.1787899950787401604, -1.692053102087505811, 0.07405724077823318263 ) ) ;
#43632=CARTESIAN_POINT ( 'NONE',  ( 3.284318927891251994E-17, -0.3892716534895436786, 0.1787899950787401882 ) ) ;
#43633=CARTESIAN_POINT ( 'NONE',  ( 0.1264236179284866091, -0.9306102361667086820, 0.1264236179284866091 ) ) ;
#43638=CARTESIAN_POINT ( 'NONE',  ( -1.100456976456230270E-17, -0.1289808174570614141, -0.1797182628040039365 ) ) ;
#43639=CARTESIAN_POINT ( 'NONE',  ( -0.1264236179284866091, -0.1295531020875065054, 0.1264236179284866091 ) ) ;
#43640=CARTESIAN_POINT ( 'NONE',  ( 0.07405724077823318263, -0.2490157479777327099, -0.1787899950787401604 ) ) ;
#43642=CARTESIAN_POINT ( 'NONE',  ( -0.1787899950787401604, -0.08169291333206318839, 0.07405724077823318263 ) ) ;
#43644=CARTESIAN_POINT ( 'NONE',  ( 0.2471886260749917852, -0.05069887331343050224, -0.1203475566266943436 ) ) ;
#43649=CARTESIAN_POINT ( 'NONE',  ( 0.07444174185955065859, -1.681638297772022783, 0.1797182628040039087 ) ) ;
#43657=CARTESIAN_POINT ( 'NONE',  ( -0.1264236179284866091, -0.3154527558517483676, 0.1264236179284866091 ) ) ;
#43659=CARTESIAN_POINT ( 'NONE',  ( -0.1264236179284866091, -1.058562992072220377, 0.1264236179284866091 ) ) ;
#43678=CARTESIAN_POINT ( 'NONE',  ( -0.07405724077823318263, -0.05216535427694517224, -0.1787899950787401604 ) ) ;
#43688=CARTESIAN_POINT ( 'NONE',  ( 0.1787899950787401604, -1.377092472166246084, 0.07405724077823318263 ) ) ;
#43689=ORIENTED_EDGE ( 'NONE', *, *, #582, .F. ) ;
#43690=CARTESIAN_POINT ( 'NONE',  ( 0.07405724077823318263, -0.3031496062454492879, 0.1787899950787401604 ) ) ;
#43698=CARTESIAN_POINT ( 'NONE',  ( -0.1264236179284866091, -1.585137795221826629, -0.1264236179284866091 ) ) ;
#43699=CARTESIAN_POINT ( 'NONE',  ( 0.1264236179284866091, -1.639271653489543290, 0.1264236179284866091 ) ) ;
#43704=CARTESIAN_POINT ( 'NONE',  ( -0.07444174185955065859, -1.307622549740526052, -0.1797182628040039087 ) ) ;
#43706=B_SPLINE_CURVE_WITH_KNOTS ( 'NONE', 3,
 ( #20273, #2066, #5183, #13341, #19804, #27970, #9507, #34436, #31098, #45658, #12876, #30867, #27510, #45902, #13118, #24354, #1582, #34680, #42315, #23646, #9739 ),
 .UNSPECIFIED., .F., .F.,
 ( 4, 2, 1, 1, 2, 2, 2, 1, 1, 1, 2, 2, 4 ),
 ( 0.000000000000000000, 0.1249999999999996669, 0.1874999999999995004, 0.2187499999999994171, 0.2343749999999993894, 0.2499999999999993339, 0.3749999999999966693, 0.4374999999999952816, 0.4687499999999946709, 0.4843749999999945044, 0.4921874999999945044, 0.4999999999999945599, 1.000000000000000000 ),
 .UNSPECIFIED. ) ;
#43725=CARTESIAN_POINT ( 'NONE',  ( -0.1574803149606297803, -1.038877952648378900, 0.06523048226347956391 ) ) ;
#43732=CARTESIAN_POINT ( 'NONE',  ( -0.1264236179284866091, 0.004429133912031228346, 0.1264236179284866091 ) ) ;
#43740=CARTESIAN_POINT ( 'NONE',  ( 0.06523048226347956391, 0.08809055128862934569, -0.1574803149606300301 ) ) ;
#43751=CARTESIAN_POINT ( 'NONE',  ( 0.1264236179284866091, -0.8972696375205767572, -0.1264236179284866091 ) ) ;
#43753=CARTESIAN_POINT ( 'NONE',  ( -0.1574803149606299191, -0.01771653532554381960, 0.000000000000000000 ) ) ;
#43765=CARTESIAN_POINT ( 'NONE',  ( -0.1797182628040039087, -0.7859690064334394766, 0.07444174185955065859 ) ) ;
#43769=CARTESIAN_POINT ( 'NONE',  ( -0.1258674519624516375, 0.1236212482586854927, -0.1007786101663682155 ) ) ;
#43772=EDGE_CURVE ( 'NONE', #1072, #13671, #19703, .T. ) ;
#43781=CARTESIAN_POINT ( 'NONE',  ( -0.1787899950787401604, -0.7116141731745821986, -0.07405724077823318263 ) ) ;
#43791=CARTESIAN_POINT ( 'NONE',  ( -0.1113553986120547346, -1.528543307086614123, -0.1113553986120547346 ) ) ;
#43795=CARTESIAN_POINT ( 'NONE',  ( 2.892866454678787531E-17, 0.1003937007874015908, 0.1574803149606299191 ) ) ;
#43804=CARTESIAN_POINT ( 'NONE',  ( 3.284318927891251994E-17, -0.3608523146859319297, 0.1787899950787401882 ) ) ;
#43815=CARTESIAN_POINT ( 'NONE',  ( 0.1787899950787401882, -1.245570866087968520, -2.189545951927503898E-17 ) ) ;
#43816=CARTESIAN_POINT ( 'NONE',  ( 3.284318927891251994E-17, -1.447342519631275692, 0.1787899950787401882 ) ) ;
#43823=CARTESIAN_POINT ( 'NONE',  ( -0.1113553986120547346, -0.1112204724409448786, -0.1113553986120547346 ) ) ;
#43834=CARTESIAN_POINT ( 'NONE',  ( -0.1787899950787401604, -0.03740157474938609478, 0.07405724077823318263 ) ) ;
#43838=CARTESIAN_POINT ( 'NONE',  ( 0.1264236179284866091, -1.639271653489543290, 0.1264236179284866091 ) ) ;
#43839=CARTESIAN_POINT ( 'NONE',  ( 0.1574803149606299191, -1.494094488081448846, -1.928577636452523993E-17 ) ) ;
#43840=CARTESIAN_POINT ( 'NONE',  ( 0.1787899950787401604, -0.7755905511273385455, 0.07405724077823318263 ) ) ;
#43842=CARTESIAN_POINT ( 'NONE',  ( 0.1113553986120547346, -0.9872047244094488416, -0.1113553986120547346 ) ) ;
#43844=AXIS2_PLACEMENT_3D ( 'NONE', #5931, #20548, #24391 ) ;
#43849=ORIENTED_EDGE ( 'NONE', *, *, #39590, .T. ) ;
#43856=CARTESIAN_POINT ( 'NONE',  ( 0.1574803149606300301, -0.07431102351452013866, -0.06523048226347956391 ) ) ;
#43865=CARTESIAN_POINT ( 'NONE',  ( -0.1205236854640061028, -0.09851384067577953485, -0.1371198999545033548 ) ) ;
#43873=CARTESIAN_POINT ( 'NONE',  ( 0.1787899950787401604, -0.8444881889226140137, -0.07405724077823318263 ) ) ;
#43878=CARTESIAN_POINT ( 'NONE',  ( 0.1270800023317771588, -0.1831146757247779644, 0.1270800023317771588 ) ) ;
#43879=CARTESIAN_POINT ( 'NONE',  ( -0.1787899950787401604, -0.1713838107489239204, 0.07405724077823318263 ) ) ;
#43880=CARTESIAN_POINT ( 'NONE',  ( -0.1787899950787401604, -0.3179133857730082058, -0.07405724077823318263 ) ) ;
#43881=CARTESIAN_POINT ( 'NONE',  ( 0.07405724077823318263, -0.1112204723871813017, 0.1787899950787401604 ) ) ;
#43883=CARTESIAN_POINT ( 'NONE',  ( 0.2471922967771570667, -0.09275221067063771363, -0.04038134086897739172 ) ) ;
#43887=DIRECTION ( 'NONE',  ( -0.000000000000000000, 1.000000000000000000, 0.000000000000000000 ) ) ;
#43889=DIRECTION ( 'NONE',  ( 0.000000000000000000, 0.000000000000000000, 1.000000000000000000 ) ) ;
#43891=DIRECTION ( 'NONE',  ( 0.000000000000000000, -1.000000000000000000, 0.000000000000000000 ) ) ;
#43896=CARTESIAN_POINT ( 'NONE',  ( 0.07405724077823318263, -0.3474409448281265411, 0.1787899950787401604 ) ) ;
#43898=CARTESIAN_POINT ( 'NONE',  ( -1.094772975963752103E-17, -1.112696850339937038, -0.1787899950787401882 ) ) ;
#43905=CARTESIAN_POINT ( 'NONE',  ( 0.06523048226347956391, -1.147145669183812222, 0.1574803149606297803 ) ) ;
#43916=CARTESIAN_POINT ( 'NONE',  ( 0.07405724077823318263, 0.04625984257344856188, 0.1787899950787401604 ) ) ;
#43927=CARTESIAN_POINT ( 'NONE',  ( -0.07405724077823318263, -1.283588535158372457, -0.1787899950787401604 ) ) ;
#43928=AXIS2_PLACEMENT_3D ( 'NONE', #6921, #24440, #21301 ) ;
#43929=EDGE_LOOP ( 'NONE', ( #35116, #41579, #8815, #13802 ) ) ;
#43930=CARTESIAN_POINT ( 'NONE',  ( -0.1264236179284866091, -0.2317913385289138151, 0.1264236179284866091 ) ) ;
#43939=CARTESIAN_POINT ( 'NONE',  ( -0.07405724077823318263, -1.705708661363559253, -0.1787899950787401604 ) ) ;
#43940=CARTESIAN_POINT ( 'NONE',  ( 0.07405724077823318263, -1.626968503883244876, -0.1787899950787401604 ) ) ;
#43943=CARTESIAN_POINT ( 'NONE',  ( 3.301370929368692659E-17, -1.487248533992494126, 0.1797182628040039365 ) ) ;
#43969=CARTESIAN_POINT ( 'NONE',  ( -0.1264236179284866091, -0.1530511810485988278, 0.1264236179284866091 ) ) ;
#43977=CARTESIAN_POINT ( 'NONE',  ( 0.1574803149606300301, 0.03887795286343254109, 0.06523048226347956391 ) ) ;
#43986=CYLINDRICAL_SURFACE ( 'NONE', #16012, 0.2204724409448818867 ) ;
#43987=CARTESIAN_POINT ( 'NONE',  ( -0.1787899950787401604, -0.8849664879142767893, -0.07405724077823318263 ) ) ;
#43989=CARTESIAN_POINT ( 'NONE',  ( -0.1264236179284866091, 0.1225393701325037388, 0.1264236179284866091 ) ) ;
#43994=ADVANCED_FACE ( 'NONE', ( #7235 ), #21855, .F. ) ;
#43999=CARTESIAN_POINT ( 'NONE',  ( 0.1270800023317771588, -0.8524060143074547735, 0.1270800023317771588 ) ) ;
#44006=CARTESIAN_POINT ( 'NONE',  ( 0.06523048226347977208, 0.1126968505012277827, 0.1574803149606297803 ) ) ;
#44010=CARTESIAN_POINT ( 'NONE',  ( -0.1787899950787401604, -0.7903543306548983516, -0.07405724077823318263 ) ) ;
#44017=CARTESIAN_POINT ( 'NONE',  ( -0.1113553986120547346, -1.725393700787401841, -0.1113553986120547346 ) ) ;
#44019=( BOUNDED_CURVE ( )  B_SPLINE_CURVE ( 2, ( #16390, #19956, #26472, #4863, #45109, #34596, #31010, #12084, #1746 ),
 .UNSPECIFIED., .F., .T. ) 
 B_SPLINE_CURVE_WITH_KNOTS ( ( 3, 2, 2, 2, 3 ),
 ( 0.09500000000000000111, 0.09750000000000000333, 0.1000000000000000056, 0.1024999999999999939, 0.1049999999999999961 ),
 .UNSPECIFIED. ) 
 CURVE ( )  GEOMETRIC_REPRESENTATION_ITEM ( )  RATIONAL_B_SPLINE_CURVE ( ( 1.000000000000000000, 0.9238795325112869605, 1.000000000000000000, 0.9238795325112869605, 1.000000000000000000, 0.9238795325112869605, 1.000000000000000000, 0.9238795325112869605, 1.000000000000000000 ) ) 
 REPRESENTATION_ITEM ( '' )  ) ;
#44024=CARTESIAN_POINT ( 'NONE',  ( 0.1264236179284866091, -1.437499999946236340, -0.1264236179284866091 ) ) ;
#44036=CARTESIAN_POINT ( 'NONE',  ( 0.1787899950787401604, -0.3534704249221524153, 0.07405724077823318263 ) ) ;
#44037=CARTESIAN_POINT ( 'NONE',  ( -0.2305915495022031469, -0.08955974388200925451, -0.07008671854853071315 ) ) ;
#44041=EDGE_CURVE ( 'NONE', #3128, #47458, #6554, .T. ) ;
#44049=CARTESIAN_POINT ( 'NONE',  ( 3.284318927891251994E-17, -1.294783464513165283, 0.1787899950787401882 ) ) ;
#44050=CARTESIAN_POINT ( 'NONE',  ( 0.1787899950787401882, -1.358759842465921297, -2.189545951927503898E-17 ) ) ;
#44059=CARTESIAN_POINT ( 'NONE',  ( -9.642888182262618425E-18, -0.3523622047244094335, -0.1574803149606299191 ) ) ;
#44070=VERTEX_POINT ( 'NONE', #32100 ) ;
#44073=CARTESIAN_POINT ( 'NONE',  ( 0.07405724077823318263, -1.587598425143086800, -0.1787899950787401604 ) ) ;
#44074=CARTESIAN_POINT ( 'NONE',  ( 0.1574803149606299191, -1.572834645561763667, -1.928577636452523993E-17 ) ) ;
#44075=CARTESIAN_POINT ( 'NONE',  ( -0.07405724077823318263, -0.8001968503399367050, -0.1787899950787401604 ) ) ;
#44076=CARTESIAN_POINT ( 'NONE',  ( -9.642888182262618425E-18, -1.100393700787401619, -0.1574803149606299191 ) ) ;
#44098=CARTESIAN_POINT ( 'NONE',  ( 0.000000000000000000, 0.1102362204724409434, 0.000000000000000000 ) ) ;
#44102=CARTESIAN_POINT ( 'NONE',  ( -0.009589690922603031839, -0.09851384308256634637, -0.1896418766835074876 ) ) ;
#44106=CARTESIAN_POINT ( 'NONE',  ( -0.2471922904502826535, 0.05203836715090711523, -0.1197978718290576422 ) ) ;
#44110=CARTESIAN_POINT ( 'NONE',  ( -0.1787899950787401882, -0.8715551180564724554, 0.000000000000000000 ) ) ;
#44111=CARTESIAN_POINT ( 'NONE',  ( -0.1264236179284866091, -0.4335629920722205433, 0.1264236179284866091 ) ) ;
#44112=CARTESIAN_POINT ( 'NONE',  ( -0.1787899950787401604, -0.9429133857730090940, 0.07405724077823318263 ) ) ;
#44114=CARTESIAN_POINT ( 'NONE',  ( 0.1797182628040039365, -0.1388233371421006002, -2.200913952912460540E-17 ) ) ;
#44115=CARTESIAN_POINT ( 'NONE',  ( 0.1264236179284866091, -0.02017716530056720692, -0.1264236179284866091 ) ) ;
#44116=CARTESIAN_POINT ( 'NONE',  ( 0.000000000000000000, -0.09842519685039370636, 0.000000000000000000 ) ) ;
#44126=CARTESIAN_POINT ( 'NONE',  ( 4.681852760415787419E-17, -0.03219022224904102836, 0.2854330708661417804 ) ) ;
#44127=CARTESIAN_POINT ( 'NONE',  ( 0.1264236179284866091, -0.2662401574265516047, 0.1264236179284866091 ) ) ;
#44130=CARTESIAN_POINT ( 'NONE',  ( 0.1787899950787401604, -1.001968503883243988, -0.07405724077823318263 ) ) ;
#44137=ADVANCED_FACE ( 'NONE', ( #21292 ), #40244, .T. ) ;
#44139=CARTESIAN_POINT ( 'NONE',  ( 2.892866454678787531E-17, -1.188976377845228471, 0.1574803149606299191 ) ) ;
#44156=CARTESIAN_POINT ( 'NONE',  ( 0.1787899950787401604, -1.411541291063884929, -0.07405724077823318263 ) ) ;
#44158=CARTESIAN_POINT ( 'NONE',  ( -1.094772975963752103E-17, -0.2859251967966303098, -0.1787899950787401882 ) ) ;
#44169=CARTESIAN_POINT ( 'NONE',  ( -0.1270800023317771588, -1.413429636354698760, 0.1270800023317771588 ) ) ;
#44190=CARTESIAN_POINT ( 'NONE',  ( 0.1797182628040039087, -0.1019138883232029447, 0.07444174185955046430 ) ) ;
#44192=CARTESIAN_POINT ( 'NONE',  ( 0.1113553986120547346, -1.065944881782236342, 0.1113553986120547346 ) ) ;
#44198=CARTESIAN_POINT ( 'NONE',  ( 3.284318927891251994E-17, -0.1481299212060791237, 0.1787899950787401882 ) ) ;
#44206=CARTESIAN_POINT ( 'NONE',  ( -0.06523048226347956391, 0.1323818898713065573, -0.1574803149606300301 ) ) ;
#44212=DIRECTION ( 'NONE',  ( 0.000000000000000000, 0.000000000000000000, -1.000000000000000000 ) ) ;
#44213=CARTESIAN_POINT ( 'NONE',  ( 0.1787899950787401604, -0.7816200312213649193, -0.07405724077823318263 ) ) ;
#44222=CARTESIAN_POINT ( 'NONE',  ( -0.1787899950787401882, -0.5172244093950552069, 0.000000000000000000 ) ) ;
#44226=CARTESIAN_POINT ( 'NONE',  ( -0.1270800023317771588, -1.068941447378320975, -0.1270800023317771588 ) ) ;
#44238=CARTESIAN_POINT ( 'NONE',  ( -0.1787899950787401882, -0.7485236219934803259, 0.000000000000000000 ) ) ;
#44246=CARTESIAN_POINT ( 'NONE',  ( 0.06523048226347956391, -1.747539370078740717, 0.1574803149606297803 ) ) ;
#44254=B_SPLINE_CURVE_WITH_KNOTS ( 'NONE', 3,
 ( #46214, #45979, #16540, #30700, #45265, #27588, #7150, #21285, #28758, #46926, #14354, #20818, #10045, #47170, #6902, #35457, #9820, #32092, #39257, #31868 ),
 .UNSPECIFIED., .F., .F.,
 ( 4, 1, 1, 1, 1, 1, 2, 2, 1, 1, 1, 2, 2, 4 ),
 ( 0.000000000000000000, 0.2499999999999940048, 0.3749999999999910072, 0.4374999999999891753, 0.4687499999999880096, 0.4843749999999875655, 0.4921874999999874545, 0.4999999999999873990, 0.6249999999999876765, 0.6874999999999874545, 0.7187499999999875655, 0.7343749999999877875, 0.7499999999999881206, 1.000000000000000000 ),
 .UNSPECIFIED. ) ;
#44262=CARTESIAN_POINT ( 'NONE',  ( -8.354793841626791791E-17, 0.03219022224904082713, -0.2854330708661417804 ) ) ;
#44264=CARTESIAN_POINT ( 'NONE',  ( -0.08276828494985000173, -0.08956000829960196474, 0.2091008467216779743 ) ) ;
#44265=CARTESIAN_POINT ( 'NONE',  ( -0.2471922904502826812, -0.09842519685039370636, 0.1427165354330708902 ) ) ;
#44266=DIRECTION ( 'NONE',  ( 0.000000000000000000, 1.000000000000000000, 0.000000000000000000 ) ) ;
#44271=CARTESIAN_POINT ( 'NONE',  ( -0.1264236179284866091, -1.339074803095842592, 0.1264236179284866091 ) ) ;
#44272=CARTESIAN_POINT ( 'NONE',  ( 0.1787899950787401604, -1.553149606245448178, -0.07405724077823318263 ) ) ;
#44280=CARTESIAN_POINT ( 'NONE',  ( 0.1113553986120547346, -0.2490157480314960647, 0.1113553986120547346 ) ) ;
#44288=CARTESIAN_POINT ( 'NONE',  ( -0.1113553986120547346, -0.5639763778452283605, 0.1113553986120547346 ) ) ;
#44291=CARTESIAN_POINT ( 'NONE',  ( -0.1694883852340978991, -0.08955000340450794405, 0.001402097216817517434 ) ) ;
#44299=CARTESIAN_POINT ( 'NONE',  ( 3.284318927891251994E-17, -1.604822834591905556, 0.1787899950787401882 ) ) ;
#44300=CARTESIAN_POINT ( 'NONE',  ( 0.1787899950787401604, -0.7312992125446612368, -0.07405724077823318263 ) ) ;
#44301=CARTESIAN_POINT ( 'NONE',  ( 0.1113553986120547346, -1.184055118110236338, -0.1113553986120547346 ) ) ;
#44310=CARTESIAN_POINT ( 'NONE',  ( -0.1574803149606297803, -1.314468503829480550, 0.06523048226347956391 ) ) ;
#44316=CARTESIAN_POINT ( 'NONE',  ( 0.1113553986120547346, -0.07185039359326043928, -0.1113553986120547346 ) ) ;
#44319=CARTESIAN_POINT ( 'NONE',  ( 0.05729443792182561251, 0.07836113345104780969, 0.2523541117089074803 ) ) ;
#44326=CARTESIAN_POINT ( 'NONE',  ( 0.09778643531992912974, -0.09851382616417500571, 0.1118397558297255928 ) ) ;
#44333=CARTESIAN_POINT ( 'NONE',  ( 0.07405724077823318263, -0.8838582676627719792, -0.1787899950787401604 ) ) ;
#44334=CARTESIAN_POINT ( 'NONE',  ( 0.1787899950787401882, -1.122539370024976391, -2.189545951927503898E-17 ) ) ;
#44337=CARTESIAN_POINT ( 'NONE',  ( -0.1270800023317771588, -0.1240595576145415435, -0.1270800023317771588 ) ) ;
#44351=CARTESIAN_POINT ( 'NONE',  ( 0.1787899950787401604, -0.2194881889226144023, -0.07405724077823318263 ) ) ;
#44353=CARTESIAN_POINT ( 'NONE',  ( 0.07405724077823318263, -1.233267716481668774, -0.1787899950787401604 ) ) ;
#44361=CARTESIAN_POINT ( 'NONE',  ( 0.1574803149606300301, -1.176673228238929614, -0.06523048226347956391 ) ) ;
#44364=CARTESIAN_POINT ( 'NONE',  ( -0.1519198807041087229, -0.09842519685039373412, -0.09441072998970326258 ) ) ;
#44379=CARTESIAN_POINT ( 'NONE',  ( -0.1787899950787401604, -1.514887747756799019, -0.07405724077823318263 ) ) ;
#44381=CARTESIAN_POINT ( 'NONE',  ( 0.07405724077823318263, -0.4999999999462365619, 0.1787899950787401604 ) ) ;
#44390=CARTESIAN_POINT ( 'NONE',  ( -0.1787899950787401882, -1.580216535379306952, 0.000000000000000000 ) ) ;
#44391=CARTESIAN_POINT ( 'NONE',  ( 0.1787899950787401604, -1.671259842465922407, -0.07405724077823318263 ) ) ;
#44395=CARTESIAN_POINT ( 'NONE',  ( -0.06523048226347956391, -0.5713582677165348622, 0.1574803149606297803 ) ) ;
#44396=CARTESIAN_POINT ( 'NONE',  ( -0.07444174185955065859, -1.386362707220842205, -0.1797182628040039087 ) ) ;
#44402=ADVANCED_FACE ( 'NONE', ( #29949 ), #421, .T. ) ;
#44406=CARTESIAN_POINT ( 'NONE',  ( 0.1787899950787401604, 0.1348425197388028463, -0.07405724077823318263 ) ) ;
#44416=CARTESIAN_POINT ( 'NONE',  ( -0.1270800023317771588, -0.04531940013422661173, -0.1270800023317771588 ) ) ;
#44418=CARTESIAN_POINT ( 'NONE',  ( -0.1264236179284866091, -1.230807086560409269, -0.1264236179284866091 ) ) ;
#44427=CARTESIAN_POINT ( 'NONE',  ( 0.07405724077823318263, -0.1850393700249766959, 0.1787899950787401604 ) ) ;
#44430=CARTESIAN_POINT ( 'NONE',  ( 0.1686160743796767669, -0.08918665060135554101, -0.1880811715460162514 ) ) ;
#44434=CARTESIAN_POINT ( 'NONE',  ( -0.1574803149606299191, -0.09645669280585884853, 0.000000000000000000 ) ) ;
#44436=VERTEX_POINT ( 'NONE', #18638 ) ;
#44440=CARTESIAN_POINT ( 'NONE',  ( -1.094772975963752103E-17, -0.9710885351583720126, -0.1787899950787401882 ) ) ;
#44450=ADVANCED_FACE ( 'NONE', ( #11465 ), #40659, .F. ) ;
#44453=CARTESIAN_POINT ( 'NONE',  ( -0.1264236179284866091, -0.5123031495525355306, 0.1264236179284866091 ) ) ;
#44459=CARTESIAN_POINT ( 'NONE',  ( -0.1797182628040039087, -0.9434493213940695622, 0.07444174185955065859 ) ) ;
#44470=CARTESIAN_POINT ( 'NONE',  ( 0.1787899950787401604, -0.8444881889226140137, -0.07405724077823318263 ) ) ;
#44476=CARTESIAN_POINT ( 'NONE',  ( 0.06523048226347956391, -1.693405511811024944, -0.1574803149606300301 ) ) ;
#44481=CARTESIAN_POINT ( 'NONE',  ( -0.1574803149606300301, -0.2957677164279057802, -0.06523048226347956391 ) ) ;
#44490=CARTESIAN_POINT ( 'NONE',  ( 0.1006623723854972452, 0.09658349877441904652, -0.2273156230721085636 ) ) ;
#44491=DIRECTION ( 'NONE',  ( 0.000000000000000000, 1.000000000000000000, 0.000000000000000000 ) ) ;
#44492=CARTESIAN_POINT ( 'NONE',  ( -0.1264236179284866091, -0.4838838107489236706, 0.1264236179284866091 ) ) ;
#44493=CARTESIAN_POINT ( 'NONE',  ( 0.09776075193326634605, -0.09842519685039370636, 0.1118142777513527475 ) ) ;
#44498=CARTESIAN_POINT ( 'NONE',  ( -0.1264236179284866091, -1.704356251693805335, 0.1264236179284866091 ) ) ;
#44507=CARTESIAN_POINT ( 'NONE',  ( 0.1787899950787401604, -1.321850393647023392, -0.07405724077823318263 ) ) ;
#44508=CARTESIAN_POINT ( 'NONE',  ( 0.1787899950787401882, -1.594980314906866203, -2.189545951927503898E-17 ) ) ;
#44517=CARTESIAN_POINT ( 'NONE',  ( 0.1574803149606299191, -0.2834645669291338543, -1.928577636452523993E-17 ) ) ;
#44521=ORIENTED_EDGE ( 'NONE', *, *, #11592, .F. ) ;
#44522=CARTESIAN_POINT ( 'NONE',  ( -0.1363753864968494101, -0.09373322739561565364, -0.1156200648374353240 ) ) ;
#44526=CARTESIAN_POINT ( 'NONE',  ( -0.1064406243220434034, -0.08956136075716661371, 0.1198387747093381250 ) ) ;
#44527=ORIENTED_EDGE ( 'NONE', *, *, #38095, .F. ) ;
#44533=CARTESIAN_POINT ( 'NONE',  ( -0.1787899950787401882, -1.535925196796629866, 0.000000000000000000 ) ) ;
#44534=CARTESIAN_POINT ( 'NONE',  ( 0.07405724077823318263, -0.7411417322297018107, 0.1787899950787401604 ) ) ;
#44535=CARTESIAN_POINT ( 'NONE',  ( 2.892866454678787531E-17, -1.159448818897637956, 0.1574803149606299191 ) ) ;
#44558=CARTESIAN_POINT ( 'NONE',  ( -0.06612450700486259547, -0.09851382860064350488, 0.1467596715283011888 ) ) ;
#44568=CARTESIAN_POINT ( 'NONE',  ( -0.07405724077823318263, -0.9183070865604088251, -0.1787899950787401604 ) ) ;
#44569=CARTESIAN_POINT ( 'NONE',  ( 0.07405724077823318263, -1.051181102308440529, 0.1787899950787401604 ) ) ;
#44570=CARTESIAN_POINT ( 'NONE',  ( -0.1270800023317771588, -0.3209099513153291783, -0.1270800023317771588 ) ) ;
#44571=CARTESIAN_POINT ( 'NONE',  ( -0.06523048226347956391, 0.1619094488188975167, -0.1574803149606300301 ) ) ;
#44572=CARTESIAN_POINT ( 'NONE',  ( 0.07405724077823318263, -0.05708661411946481384, -0.1787899950787401604 ) ) ;
#44575=( CONVERSION_BASED_UNIT ( 'INCH', #33142 ) LENGTH_UNIT ( ) NAMED_UNIT ( #28348 ) ) ;
#44582=CARTESIAN_POINT ( 'NONE',  ( 3.284318927891251994E-17, -0.2711614172690712810, 0.1787899950787401882 ) ) ;
#44585=CARTESIAN_POINT ( 'NONE',  ( 0.07405724077823318263, -1.193897637741512696, -0.1787899950787401604 ) ) ;
#44596=CARTESIAN_POINT ( 'NONE',  ( -0.1187775451116823144, -0.09842519684033429472, -0.1336329292046753159 ) ) ;
#44604=CARTESIAN_POINT ( 'NONE',  ( -0.2112885751001251922, -0.09851385201003405589, -0.1284757149005590626 ) ) ;
#44610=CARTESIAN_POINT ( 'NONE',  ( -0.1264236179284866091, -1.438608220197742149, -0.1264236179284866091 ) ) ;
#44612=CARTESIAN_POINT ( 'NONE',  ( 0.1787899950787401604, -0.3769685038832444324, 0.07405724077823318263 ) ) ;
#44613=CARTESIAN_POINT ( 'NONE',  ( -0.06523048226347956391, 0.01427165365083412490, -0.1574803149606300301 ) ) ;
#44619=LINE ( 'NONE', #37215, #29476 ) ;
#44623=CARTESIAN_POINT ( 'NONE',  ( -0.1787899950787401604, -1.779527559001355952, -0.07405724077823318263 ) ) ;
#44627=CARTESIAN_POINT ( 'NONE',  ( -0.06523048226347956391, -0.7682086614173235795, 0.1574803149606297803 ) ) ;
#44629=CARTESIAN_POINT ( 'NONE',  ( -0.1797182628040039087, -1.460181604858636906, -0.07444174185955065859 ) ) ;
#44631=CARTESIAN_POINT ( 'NONE',  ( 0.2471922904502825424, 0.07319706521782758102, -0.08615678709746438235 ) ) ;
#44638=CARTESIAN_POINT ( 'NONE',  ( 2.892866454678787531E-17, -0.8346456691838110009, 0.1574803149606299191 ) ) ;
#44648=CARTESIAN_POINT ( 'NONE',  ( -0.1797182628040039087, -0.04285877021296678052, -0.07444174185955065859 ) ) ;
#44650=CARTESIAN_POINT ( 'NONE',  ( -0.1787899950787401882, -1.147145669237574772, 0.000000000000000000 ) ) ;
#44655=CARTESIAN_POINT ( 'NONE',  ( -0.1574803149606297803, 0.05364173228346463818, 0.06523048226347956391 ) ) ;
#44659=CARTESIAN_POINT ( 'NONE',  ( 0.07405724077823318263, -0.1702755904974175283, -0.1787899950787401604 ) ) ;
#44661=CARTESIAN_POINT ( 'NONE',  ( -0.06523048226347956391, 0.08316929133858273759, -0.1574803149606300301 ) ) ;
#44666=CARTESIAN_POINT ( 'NONE',  ( 0.1574803149606299191, -0.1161417321759375954, -1.928577636452523993E-17 ) ) ;
#44669=ORIENTED_EDGE ( 'NONE', *, *, #152, .T. ) ;
#44674=CARTESIAN_POINT ( 'NONE',  ( 0.1787899950787401604, -1.057210582402466903, -0.07405724077823318263 ) ) ;
#44676=CARTESIAN_POINT ( 'NONE',  ( 0.1787899950787401604, 0.02165354336085011100, -0.07405724077823318263 ) ) ;
#44687=CARTESIAN_POINT ( 'NONE',  ( -0.1797182628040039087, -1.066480817457060581, -0.07444174185955065859 ) ) ;
#44701=CARTESIAN_POINT ( 'NONE',  ( 0.07405724077823318263, -0.7608267715997808489, -0.1787899950787401604 ) ) ;
#44707=ADVANCED_FACE ( 'NONE', ( #34938 ), #46166, .T. ) ;
#44709=CARTESIAN_POINT ( 'NONE',  ( 0.1574803149606300301, -1.737696850393700032, -0.06523048226347956391 ) ) ;
#44719=CARTESIAN_POINT ( 'NONE',  ( -0.1574803149606297803, -0.2908464565853862149, 0.06523048226347956391 ) ) ;
#44720=CARTESIAN_POINT ( 'NONE',  ( 0.1787899950787401604, -1.602362204670647161, 0.07405724077823318263 ) ) ;
#44722=CIRCLE ( 'NONE', #15692, 0.2007874015748031815 ) ;
#44732=CARTESIAN_POINT ( 'NONE',  ( -0.1787899950787401604, -0.5257145194103405306, 0.07405724077823318263 ) ) ;
#44733=CARTESIAN_POINT ( 'NONE',  ( -0.2055635559985952709, -0.08955966668076850712, -0.1312247587652915493 ) ) ;
#44735=DIRECTION ( 'NONE',  ( 0.000000000000000000, 0.000000000000000000, 1.000000000000000000 ) ) ;
#44737=CARTESIAN_POINT ( 'NONE',  ( -0.1264236179284866091, -1.822466487914279565, 0.1264236179284866091 ) ) ;
#44743=CARTESIAN_POINT ( 'NONE',  ( -0.1787899950787401604, -1.267716535379307619, -0.07405724077823318263 ) ) ;
#44744=CARTESIAN_POINT ( 'NONE',  ( 0.07405724077823318263, -1.548228346402928723, -0.1787899950787401604 ) ) ;
#44752=CARTESIAN_POINT ( 'NONE',  ( 0.06523048226347956391, -0.3302165354330710012, 0.1574803149606297803 ) ) ;
#44757=CARTESIAN_POINT ( 'NONE',  ( -0.1331022545968926496, -0.09301241491031153608, -0.1193785939374830685 ) ) ;
#44762=CARTESIAN_POINT ( 'NONE',  ( -0.1692806188707426940, -0.08955568274170122578, -0.02334579719831987241 ) ) ;
#44769=CARTESIAN_POINT ( 'NONE',  ( -1.094772975963752103E-17, -1.624507873961984261, -0.1787899950787401882 ) ) ;
#44770=CARTESIAN_POINT ( 'NONE',  ( -0.1264236179284866091, -0.9060039369541103005, 0.1264236179284866091 ) ) ;
#44771=CARTESIAN_POINT ( 'NONE',  ( -9.642888182262618425E-18, -1.179133858267716661, -0.1574803149606299191 ) ) ;
#44773=EDGE_CURVE ( 'NONE', #30751, #2574, #22595, .T. ) ;
#44781=CARTESIAN_POINT ( 'NONE',  ( 0.06523048226347956391, -1.304625984144440309, 0.1574803149606297803 ) ) ;
#44797=CARTESIAN_POINT ( 'NONE',  ( -0.01524196446234527512, -0.09851383026906693208, 0.1563901584214165141 ) ) ;
#44805=CARTESIAN_POINT ( 'NONE',  ( -1.094772975963752103E-17, -0.8813976377415118080, -0.1787899950787401882 ) ) ;
#44806=CARTESIAN_POINT ( 'NONE',  ( 0.1264236179284866091, -1.009350393647023614, 0.1264236179284866091 ) ) ;
#44809=CARTESIAN_POINT ( 'NONE',  ( -0.1797182628040039087, -0.3135280615515493308, 0.07444174185955065859 ) ) ;
#44810=CARTESIAN_POINT ( 'NONE',  ( 0.1574803149606299191, 0.1496062992125984370, -1.928577636452523993E-17 ) ) ;
#44812=CARTESIAN_POINT ( 'NONE',  ( -0.07405724077823318263, -0.1555118109698585271, 0.1787899950787401604 ) ) ;
#44824=CARTESIAN_POINT ( 'NONE',  ( -0.1787899950787401604, -0.4803149605761579677, -0.07405724077823318263 ) ) ;
#44826=CARTESIAN_POINT ( 'NONE',  ( -0.07405724077823318263, -1.267716535379307619, -0.1787899950787401604 ) ) ;
#44839=CARTESIAN_POINT ( 'NONE',  ( 0.03891730292714078859, -0.09842393336832859496, -0.1745031462337006123 ) ) ;
#44853=CARTESIAN_POINT ( 'NONE',  ( -0.1787899950787401882, -1.394316881615065284, 0.000000000000000000 ) ) ;
#44855=CARTESIAN_POINT ( 'NONE',  ( -0.1264236179284866091, -0.4384842519147402196, -0.1264236179284866091 ) ) ;
#44864=CARTESIAN_POINT ( 'NONE',  ( 3.284318927891251994E-17, -1.767224409395055318, 0.1787899950787401882 ) ) ;
#44865=CARTESIAN_POINT ( 'NONE',  ( -0.1787899950787401604, 0.1151574803687242243, 0.07405724077823318263 ) ) ;
#44869=CARTESIAN_POINT ( 'NONE',  ( 0.06523048226347956391, -0.7485236220472446522, -0.1574803149606300301 ) ) ;
#44871=CARTESIAN_POINT ( 'NONE',  ( 0.1270800023317771588, -1.393744596984620054, -0.1270800023317771588 ) ) ;
#44872=CARTESIAN_POINT ( 'NONE',  ( 0.2471922904502826257, 0.07780974138651140792, -0.07762775726530279918 ) ) ;
#44880=CARTESIAN_POINT ( 'NONE',  ( -9.642888182262618425E-18, -0.8149606298137322957, -0.1574803149606299191 ) ) ;
#44893=CARTESIAN_POINT ( 'NONE',  ( 3.301370929368692659E-17, -0.1092957780869824730, 0.1797182628040039365 ) ) ;
#44894=CARTESIAN_POINT ( 'NONE',  ( -0.07405724077823318263, -1.139763779473794925, 0.1787899950787401604 ) ) ;
#44907=CARTESIAN_POINT ( 'NONE',  ( 0.1574803149606300301, 0.004429133965794757564, -0.06523048226347956391 ) ) ;
#44915=CARTESIAN_POINT ( 'NONE',  ( -0.07405724077823318263, -1.032604283189868521, 0.1787899950787401604 ) ) ;
#44917=CARTESIAN_POINT ( 'NONE',  ( 0.1787899950787401604, 0.09547244099864542199, 0.07405724077823318263 ) ) ;
#44925=CARTESIAN_POINT ( 'NONE',  ( -0.1270800023317771588, -0.9803587702129665793, 0.1270800023317771588 ) ) ;
#44926=CARTESIAN_POINT ( 'NONE',  ( 0.1748756820900291831, 0.1299212598425196763, 0.008513987618672504490 ) ) ;
#44936=CARTESIAN_POINT ( 'NONE',  ( 0.1264236179284866091, 0.09301181107738563936, 0.1264236179284866091 ) ) ;
#44938=ADVANCED_FACE ( 'NONE', ( #11661 ), #32301, .T. ) ;
#44942=CARTESIAN_POINT ( 'NONE',  ( 0.1787899950787401604, -0.9281496062454495100, 0.07405724077823318263 ) ) ;
#44946=CARTESIAN_POINT ( 'NONE',  ( -0.1113553986120547346, -1.745078740049952781, 0.1113553986120547346 ) ) ;
#44951=CARTESIAN_POINT ( 'NONE',  ( 0.1113553986120547346, -1.656496062992126150, -0.1113553986120547346 ) ) ;
#44956=CARTESIAN_POINT ( 'NONE',  ( 0.1787899950787401604, -1.558070866087969630, -0.07405724077823318263 ) ) ;
#44965=CARTESIAN_POINT ( 'NONE',  ( 0.1787899950787401882, -0.5084901099615219966, -2.189545951927503898E-17 ) ) ;
#44966=CARTESIAN_POINT ( 'NONE',  ( -0.1080892699026834713, -0.08955964444840118499, -0.2261462449159996335 ) ) ;
#44974=CARTESIAN_POINT ( 'NONE',  ( -0.1264236179284866091, -1.378444881836000002, 0.1264236179284866091 ) ) ;
#44975=CARTESIAN_POINT ( 'NONE',  ( -0.1264236179284866091, -1.570374015694267600, 0.1264236179284866091 ) ) ;
#44986=CARTESIAN_POINT ( 'NONE',  ( -0.1574803149606300301, -0.2268700787401574381, -0.06523048226347956391 ) ) ;
#44996=CARTESIAN_POINT ( 'NONE',  ( -0.1688682454601131422, -0.08956111721935616776, 0.008132950095326338738 ) ) ;
#45005=CARTESIAN_POINT ( 'NONE',  ( -0.1787899950787401604, -1.730314960576156968, 0.07405724077823318263 ) ) ;
#45006=CARTESIAN_POINT ( 'NONE',  ( 3.284318927891251994E-17, -0.8223425196312754704, 0.1787899950787401882 ) ) ;
#45007=CARTESIAN_POINT ( 'NONE',  ( 0.06523048226347956391, -1.181594488188976610, -0.1574803149606300301 ) ) ;
#45029=CARTESIAN_POINT ( 'NONE',  ( 0.08605959628751140567, -0.09851382450317322514, 0.1221410806743637861 ) ) ;
#45034=VERTEX_POINT ( 'NONE', #22959 ) ;
#45036=CARTESIAN_POINT ( 'NONE',  ( 0.1787899950787401604, -0.8149606298674965110, 0.07405724077823318263 ) ) ;
#45039=CARTESIAN_POINT ( 'NONE',  ( 3.284318927891251994E-17, -1.093011810969858333, 0.1787899950787401882 ) ) ;
#45042=CARTESIAN_POINT ( 'NONE',  ( -0.07444174185955065859, -0.3873469591893448083, 0.1797182628040039087 ) ) ;
#45043=EDGE_CURVE ( 'NONE', #28863, #6112, #37569, .T. ) ;
#45047=B_SPLINE_CURVE_WITH_KNOTS ( 'NONE', 3,
 ( #30845, #26528, #27009, #15746, #1559, #38236, #20017, #12625, #45412, #1806, #44926, #41553, #27248, #844, #8761, #9002 ),
 .UNSPECIFIED., .F., .F.,
 ( 4, 1, 2, 2, 2, 1, 2, 2, 4 ),
 ( 0.000000000000000000, 0.1250000000000000000, 0.1874999999999999445, 0.2499999999999999167, 0.5000000000000000000, 0.6250000000000000000, 0.6875000000000000000, 0.7500000000000000000, 1.000000000000000000 ),
 .UNSPECIFIED. ) ;
#45055=CARTESIAN_POINT ( 'NONE',  ( 0.1574803149606300301, -0.9847440943806630154, 0.06523048226347956391 ) ) ;
#45056=CARTESIAN_POINT ( 'NONE',  ( 0.1787899950787401882, -0.4187992125446614589, -2.189545951927503898E-17 ) ) ;
#45058=CARTESIAN_POINT ( 'NONE',  ( 0.07405724077823318263, -1.312007873961984705, -0.1787899950787401604 ) ) ;
#45069=CARTESIAN_POINT ( 'NONE',  ( 0.05727803307417802386, -0.09842527607325883554, -0.1693749438220764070 ) ) ;
#45076=ORIENTED_EDGE ( 'NONE', *, *, #152, .F. ) ;
#45085=CARTESIAN_POINT ( 'NONE',  ( 0.07405724077823318263, -1.460753889489081692, 0.1787899950787401604 ) ) ;
#45088=CARTESIAN_POINT ( 'NONE',  ( 0.1787899950787401604, -0.4114173227808823330, -0.07405724077823318263 ) ) ;
#45100=CARTESIAN_POINT ( 'NONE',  ( -0.1787899950787401604, 0.1386555593298164635, -0.07405724077823318263 ) ) ;
#45101=CARTESIAN_POINT ( 'NONE',  ( 0.1787899950787401882, 0.1323818898175431191, -2.189545951927503898E-17 ) ) ;
#45103=EDGE_CURVE ( 'NONE', #46609, #35410, #47241, .T. ) ;
#45106=CARTESIAN_POINT ( 'NONE',  ( 0.1113553986120547346, -0.6722440944881890035, -0.1113553986120547346 ) ) ;
#45108=CARTESIAN_POINT ( 'NONE',  ( 0.07444174185955065859, -1.602898140291707074, 0.1797182628040039087 ) ) ;
#45109=CARTESIAN_POINT ( 'NONE',  ( -0.1574803149606299191, -0.05708661406570126468, 0.000000000000000000 ) ) ;
#45120=CARTESIAN_POINT ( 'NONE',  ( 3.284318927891251994E-17, 0.08316929139234625901, 0.1787899950787401882 ) ) ;
#45130=CARTESIAN_POINT ( 'NONE',  ( -1.100456976456230270E-17, -0.05024065997674630191, -0.1797182628040039365 ) ) ;
#45140=EDGE_LOOP ( 'NONE', ( #17588, #13394, #24722 ) ) ;
#45145=CARTESIAN_POINT ( 'NONE',  ( -0.1113553986120547346, -0.1013779526483785387, -0.1113553986120547346 ) ) ;
#45153=CARTESIAN_POINT ( 'NONE',  ( 3.284318927891251994E-17, -0.9907735745284508289, 0.1787899950787401882 ) ) ;
#45155=CARTESIAN_POINT ( 'NONE',  ( 0.1787899950787401604, -0.01771653537930737918, -0.07405724077823318263 ) ) ;
#45160=CARTESIAN_POINT ( 'NONE',  ( -0.1787899950787401604, -0.6328740156942683770, 0.07405724077823318263 ) ) ;
#45161=EDGE_CURVE ( 'NONE', #23021, #4670, #30478, .T. ) ;
#45165=CARTESIAN_POINT ( 'NONE',  ( 0.07444174185955065859, -0.9336068017090288773, 0.1797182628040039087 ) ) ;
#45177=CARTESIAN_POINT ( 'NONE',  ( 0.07405724077823318263, 0.09055118115612578733, 0.1787899950787401604 ) ) ;
#45180=CARTESIAN_POINT ( 'NONE',  ( -0.1787899950787401882, -0.9847440944344251212, 0.000000000000000000 ) ) ;
#45185=CARTESIAN_POINT ( 'NONE',  ( -0.06523048226347956391, -1.624507873908221489, 0.1574803149606297803 ) ) ;
#45187=LINE ( 'NONE', #37792, #29072 ) ;
#45196=CARTESIAN_POINT ( 'NONE',  ( 0.1574803149606299191, -0.3523622046168823352, -1.928577636452523993E-17 ) ) ;
#45197=CARTESIAN_POINT ( 'NONE',  ( 0.1264236179284866091, -1.516240157426551161, -0.1264236179284866091 ) ) ;
#45202=CARTESIAN_POINT ( 'NONE',  ( 0.07405724077823318263, -0.5158719997253020662, 0.1787899950787401604 ) ) ;
#45203=CARTESIAN_POINT ( 'NONE',  ( 0.0008909177745428464943, -0.08956047734530078741, -0.1867918148680964563 ) ) ;
#45215=CARTESIAN_POINT ( 'NONE',  ( -0.1787899950787401882, -1.462106299158834721, 0.000000000000000000 ) ) ;
#45216=CARTESIAN_POINT ( 'NONE',  ( 0.07405724077823318263, -1.602362204670647161, 0.1787899950787401604 ) ) ;
#45224=CARTESIAN_POINT ( 'NONE',  ( -9.642888182262618425E-18, -0.4311023622047244208, -0.1574803149606299191 ) ) ;
#45228=CARTESIAN_POINT ( 'NONE',  ( -0.1259245010770292383, -0.09152579912861666389, -0.1269212964996754567 ) ) ;
#45237=CARTESIAN_POINT ( 'NONE',  ( -0.1057326532622849119, -0.08956134917853916799, 0.1203865889276477807 ) ) ;
#45238=CARTESIAN_POINT ( 'NONE',  ( -0.07405724077823318263, -0.4803149605761579677, -0.1787899950787401604 ) ) ;
#45247=CARTESIAN_POINT ( 'NONE',  ( -0.1787899950787401604, -1.769685039316315267, 0.07405724077823318263 ) ) ;
#45248=CARTESIAN_POINT ( 'NONE',  ( -0.1787899950787401882, -0.9109251967966299768, 0.000000000000000000 ) ) ;
#45249=VECTOR ( 'NONE', #35366, 39.37007874015748143 ) ;
#45250=CARTESIAN_POINT ( 'NONE',  ( -0.1574803149606299191, -1.326771653543307172, 0.000000000000000000 ) ) ;
#45265=CARTESIAN_POINT ( 'NONE',  ( -0.1984097999861051398, 0.07306521771079745042, -0.1708811194343041739 ) ) ;
#45272=CARTESIAN_POINT ( 'NONE',  ( -0.2112569658035661491, -0.09842519685039370636, -0.1284583705656232311 ) ) ;
#45282=CARTESIAN_POINT ( 'NONE',  ( 0.07405724077823318263, -1.056102362150961982, 0.1787899950787401604 ) ) ;
#45283=CARTESIAN_POINT ( 'NONE',  ( -0.1787899950787401604, -1.061023621993481214, 0.07405724077823318263 ) ) ;
#45288=CARTESIAN_POINT ( 'NONE',  ( -1.100456976456230270E-17, -0.4045713686381637308, -0.1797182628040039365 ) ) ;
#45290=CARTESIAN_POINT ( 'NONE',  ( 0.1574803149606300301, 0.03395669291338582890, -0.06523048226347956391 ) ) ;
#45300=CARTESIAN_POINT ( 'NONE',  ( -1.094772975963752103E-17, -0.3695866141194649179, -0.1787899950787401882 ) ) ;
#45302=CARTESIAN_POINT ( 'NONE',  ( 0.07405724077823318263, -1.248031496009228913, 0.1787899950787401604 ) ) ;
#45314=CARTESIAN_POINT ( 'NONE',  ( -0.07153359775988563096, -0.09842519684882801434, -0.1638561172960870671 ) ) ;
#45330=CARTESIAN_POINT ( 'NONE',  ( -0.1787899950787401604, -1.588706645394593719, 0.07405724077823318263 ) ) ;
#45333=CARTESIAN_POINT ( 'NONE',  ( -0.1787899950787401604, -0.3572834645131658382, -0.07405724077823318263 ) ) ;
#45337=CARTESIAN_POINT ( 'NONE',  ( 0.000000000000000000, -0.09842519685039370636, 0.1574803149606299191 ) ) ;
#45339=CARTESIAN_POINT ( 'NONE',  ( 3.284318927891251994E-17, -0.2317913385289138151, 0.1787899950787401882 ) ) ;
#45343=CARTESIAN_POINT ( 'NONE',  ( 0.1264236179284866091, -1.791830708607653699, -0.1264236179284866091 ) ) ;
#45344=CARTESIAN_POINT ( 'NONE',  ( -0.1264236179284866091, -1.777066929080094670, -0.1264236179284866091 ) ) ;
#45346=CARTESIAN_POINT ( 'NONE',  ( 0.1457398918270421118, -0.09842519685039370636, 0.09125884461778420442 ) ) ;
#45349=CARTESIAN_POINT ( 'NONE',  ( -0.1574803149606299191, -0.7755905511811023167, 0.000000000000000000 ) ) ;
#45351=CARTESIAN_POINT ( 'NONE',  ( 0.07444174185955046430, -1.509394203283832780, -0.1797182628040039087 ) ) ;
#45352=CARTESIAN_POINT ( 'NONE',  ( 0.000000000000000000, -0.09842519685039370636, 0.000000000000000000 ) ) ;
#45354=CARTESIAN_POINT ( 'NONE',  ( 0.2471922904502826257, 0.08140987345727848656, -0.07064030526713212244 ) ) ;
#45361=CARTESIAN_POINT ( 'NONE',  ( 0.06523048226347956391, -0.8715551180027079070, 0.1574803149606297803 ) ) ;
#45362=CARTESIAN_POINT ( 'NONE',  ( -0.1787899950787401882, 0.07332677170730689253, 0.000000000000000000 ) ) ;
#45375=CARTESIAN_POINT ( 'NONE',  ( -0.1787899950787401604, -1.385826771599779184, -0.07405724077823318263 ) ) ;
#45385=EDGE_LOOP ( 'NONE', ( #8306, #8838, #12105, #27363 ) ) ;
#45391=CARTESIAN_POINT ( 'NONE',  ( -9.642888182262618425E-18, -0.06692913375074074911, -0.1574803149606299191 ) ) ;
#45399=CARTESIAN_POINT ( 'NONE',  ( -0.1787899950787401604, -1.003076724134751130, -0.07405724077823318263 ) ) ;
#45401=CARTESIAN_POINT ( 'NONE',  ( -0.1787899950787401604, 0.001968503990771383692, 0.07405724077823318263 ) ) ;
#45407=CARTESIAN_POINT ( 'NONE',  ( 0.1787899950787401604, -0.6131889763241887836, -0.07405724077823318263 ) ) ;
#45408=SHAPE_REPRESENTATION ( 'Threaded Bushing', ( #20860 ), #22411 ) ;
#45411=CARTESIAN_POINT ( 'NONE',  ( -0.1270800023317771588, -1.108311526118478385, -0.1270800023317771588 ) ) ;
#45412=CARTESIAN_POINT ( 'NONE',  ( 0.1732685356795573284, 0.1299212598425196763, -0.01414958902434325198 ) ) ;
#45425=CARTESIAN_POINT ( 'NONE',  ( 0.1574803149606300301, -1.727854330601133581, -0.06523048226347956391 ) ) ;
#45429=CARTESIAN_POINT ( 'NONE',  ( 0.1113553986120547346, -1.774606299212598381, -0.1113553986120547346 ) ) ;
#45436=CARTESIAN_POINT ( 'NONE',  ( -0.1264236179284866091, -1.535925196796629866, 0.1264236179284866091 ) ) ;
#45441=CARTESIAN_POINT ( 'NONE',  ( 0.06523048226347956391, -0.04478346445940203924, 0.1574803149606297803 ) ) ;
#45443=CARTESIAN_POINT ( 'NONE',  ( 0.1264236179284866091, -0.5823090075993173631, -0.1264236179284866091 ) ) ;
#45444=CARTESIAN_POINT ( 'NONE',  ( 0.06147065055149940338, -0.08956076283990217768, -0.1800941195595248401 ) ) ;
#45452=CARTESIAN_POINT ( 'NONE',  ( -0.07405724077823318263, -1.430118110182456714, -0.1787899950787401604 ) ) ;
#45456=CARTESIAN_POINT ( 'NONE',  ( 0.07444174185955065859, -0.6973863292680846371, 0.1797182628040039087 ) ) ;
#45461=CARTESIAN_POINT ( 'NONE',  ( -0.06523048226347956391, -0.4138779527559053317, 0.1574803149606297803 ) ) ;
#45473=CARTESIAN_POINT ( 'NONE',  ( 0.1264236179284866091, -0.5664370078202519698, -0.1264236179284866091 ) ) ;
#45474=CIRCLE ( 'NONE', #14894, 0.2471922904502826812 ) ;
#45481=CARTESIAN_POINT ( 'NONE',  ( 0.07405724077823318263, -1.759842519631276581, 0.1787899950787401604 ) ) ;
#45482=CARTESIAN_POINT ( 'NONE',  ( -1.094772975963752103E-17, -0.8420275590013542866, -0.1787899950787401882 ) ) ;
#45483=CARTESIAN_POINT ( 'NONE',  ( 0.1113553986120547346, -1.430118110236220597, 0.1113553986120547346 ) ) ;
#45491=CARTESIAN_POINT ( 'NONE',  ( -9.642888182262618425E-18, 0.01181102372957427288, -0.1574803149606299191 ) ) ;
#45505=CARTESIAN_POINT ( 'NONE',  ( 0.02848443417738397848, -0.09842519685039370636, 0.2212455112941330848 ) ) ;
#45515=CARTESIAN_POINT ( 'NONE',  ( 0.07405724077823318263, -1.041338582623402287, -0.1787899950787401604 ) ) ;
#45516=CARTESIAN_POINT ( 'NONE',  ( -0.1787899950787401882, -1.181594488135212506, 0.000000000000000000 ) ) ;
#45518=CARTESIAN_POINT ( 'NONE',  ( 0.07444174185955065859, -0.4611658568271400083, 0.1797182628040039087 ) ) ;
#45520=CARTESIAN_POINT ( 'NONE',  ( -0.1574803149606297803, -0.06446850393700798154, 0.06523048226347956391 ) ) ;
#45521=CARTESIAN_POINT ( 'NONE',  ( -1.094772975963752103E-17, -0.1333661416785198728, -0.1787899950787401882 ) ) ;
#45528=CARTESIAN_POINT ( 'NONE',  ( 2.458936486476969154E-17, 0.1102362204724409434, -0.2007874015748031815 ) ) ;
#45529=CARTESIAN_POINT ( 'NONE',  ( 0.1787899950787401604, -0.4950787401037172186, -0.07405724077823318263 ) ) ;
#45531=CARTESIAN_POINT ( 'NONE',  ( 3.284318927891251994E-17, -1.447342519631275692, 0.1787899950787401882 ) ) ;
#45541=CARTESIAN_POINT ( 'NONE',  ( 0.09142434311106251155, -0.09842519841270444547, -0.1536472792661565945 ) ) ;
#45551=CARTESIAN_POINT ( 'NONE',  ( -0.2333684585041059245, -0.09851385095130453518, 0.05222081355495307442 ) ) ;
#45555=CARTESIAN_POINT ( 'NONE',  ( 0.1264236179284866091, -1.655143653268608572, 0.1264236179284866091 ) ) ;
#45558=CARTESIAN_POINT ( 'NONE',  ( -0.1787899950787401604, -0.6279527558517482566, 0.07405724077823318263 ) ) ;
#45560=ORIENTED_EDGE ( 'NONE', *, *, #7469, .T. ) ;
#45563=B_SPLINE_CURVE_WITH_KNOTS ( 'NONE', 3,
 ( #16351, #44364, #12532, #15407, #37673, #15884, #34329, #11571, #15649, #1460, #11812, #26436, #26903, #40999, #44596, #41221, #30054, #26198, #40764, #16119, #4825, #8187, #18970, #7960, #4337, #5069, #37193, #45314, #992, #30287, #37425, #33632, #746, #8425, #4579, #19448, #19214, #30742, #37914, #44839, #27152, #34552, #12049, #23053, #34103, #1230, #30508, #45069, #8907, #12284, #23538, #41463, #8661, #23297, #38139, #19685, #5303, #19920, #46261, #35504, #34806, #2180, #10090, #45541, #5546, #31210, #5788, #2645, #20157, #28086, #1951, #13457, #42648, #27632, #9860, #20627, #24471, #28312, #16802, #38841, #16581, #24701, #13234, #46496, #23763, #38610, #17278, #31441, #42880, #42185, #9391, #31682 ),
 .UNSPECIFIED., .F., .F.,
 ( 4, 2, 2, 2, 1, 1, 1, 1, 2, 2, 2, 2, 2, 1, 1, 1, 2, 2, 2, 2, 2, 1, 1, 1, 1, 1, 2, 2, 2, 2, 2, 1, 1, 2, 2, 2, 2, 1, 1, 2, 2, 2, 2, 2, 1, 1, 1, 1, 2, 2, 2, 2, 2, 2, 2, 4 ),
 ( 0.000000000000000000, 0.06249999999997683797, 0.09374999999996522226, 0.1093749999999593936, 0.1171874999999565209, 0.1210937499999550498, 0.1230468749999542588, 0.1240234374999538702, 0.1245117187499537037, 0.1249999999999535372, 0.1874999999999236167, 0.2187499999999085454, 0.2343749999999009959, 0.2421874999998971656, 0.2460937499998952227, 0.2480468749998942790, 0.2490234374998938072, 0.2499999999998933353, 0.3749999999998249733, 0.4374999999997907230, 0.4687499999997736255, 0.4843749999997650213, 0.4921874999997607469, 0.4960937499997586375, 0.4980468749997575828, 0.4990234374997570832, 0.4995117187497568056, 0.4999999999997565836, 0.5312499999997701838, 0.5468749999997769562, 0.5546874999997801758, 0.5585937499997818412, 0.5605468749997827294, 0.5615234374997831734, 0.5624999999997835065, 0.5937499999997979394, 0.6093749999998051559, 0.6171874999998085976, 0.6210937499998103739, 0.6230468749998112621, 0.6249999999998121503, 0.6874999999998441247, 0.7187499999998601119, 0.7343749999998679945, 0.7421874999998719913, 0.7460937499998739897, 0.7480468749998748779, 0.7490234374998753220, 0.7495117187498755440, 0.7499999999998757660, 0.8124999999999069633, 0.8437499999999225064, 0.8593749999999301670, 0.8749999999999379385, 0.9374999999999690248, 1.000000000000000000 ),
 .UNSPECIFIED. ) ;
#45565=CARTESIAN_POINT ( 'NONE',  ( -0.07405724077823318263, -0.2096456692375751329, -0.1787899950787401604 ) ) ;
#45569=CARTESIAN_POINT ( 'NONE',  ( -0.1787899950787401604, 0.02546658295186362761, 0.07405724077823318263 ) ) ;
#45570=CARTESIAN_POINT ( 'NONE',  ( 3.284318927891251994E-17, -1.762303149552535642, 0.1787899950787401882 ) ) ;
#45575=CARTESIAN_POINT ( 'NONE',  ( -0.06523048226347956391, -0.7042322834645671215, -0.1574803149606300301 ) ) ;
#45577=CARTESIAN_POINT ( 'NONE',  ( 3.301370929368692659E-17, -1.565988691472808947, 0.1797182628040039365 ) ) ;
#45579=CARTESIAN_POINT ( 'NONE',  ( -0.1264236179284866091, -0.3597440944344256208, -0.1264236179284866091 ) ) ;
#45580=CARTESIAN_POINT ( 'NONE',  ( 0.2471922904502826257, 0.07695608958885345741, -0.07926021241888737967 ) ) ;
#45584=EDGE_CURVE ( 'NONE', #46651, #26985, #26917, .T. ) ;
#45591=CARTESIAN_POINT ( 'NONE',  ( -0.1787899950787401604, -0.002952755851748290004, 0.07405724077823318263 ) ) ;
#45602=ORIENTED_EDGE ( 'NONE', *, *, #32770, .F. ) ;
#45603=CARTESIAN_POINT ( 'NONE',  ( -0.1787899950787401882, -1.343996062938362268, 0.000000000000000000 ) ) ;
#45618=CARTESIAN_POINT ( 'NONE',  ( -9.642888182262618425E-18, -0.1456692912310557086, -0.1574803149606299191 ) ) ;
#45624=CARTESIAN_POINT ( 'NONE',  ( -0.1787899950787401604, -1.081816881615065062, -0.07405724077823318263 ) ) ;
#45626=CARTESIAN_POINT ( 'NONE',  ( 3.284318927891251994E-17, 0.04872047249470835839, 0.1787899950787401882 ) ) ;
#45632=CARTESIAN_POINT ( 'NONE',  ( -0.1787899950787401604, -0.5590551180564723444, -0.07405724077823318263 ) ) ;
#45637=CARTESIAN_POINT ( 'NONE',  ( 0.1797182628040039087, -1.120614675724778353, -0.07444174185955065859 ) ) ;
#45647=CARTESIAN_POINT ( 'NONE',  ( -0.1113553986120547346, -0.7214566928058583350, 0.1113553986120547346 ) ) ;
#45648=CARTESIAN_POINT ( 'NONE',  ( -0.1264236179284866091, 0.1126968504474643862, -0.1264236179284866091 ) ) ;
#45655=CARTESIAN_POINT ( 'NONE',  ( -0.1113553986120547346, -1.626968503829480328, 0.1113553986120547346 ) ) ;
#45658=CARTESIAN_POINT ( 'NONE',  ( 0.08392772586502213195, -0.09126532511095285238, 0.2369773207360968970 ) ) ;
#45659=CARTESIAN_POINT ( 'NONE',  ( -0.1113553986120547346, -1.754921259842519676, 0.1113553986120547346 ) ) ;
#45666=CARTESIAN_POINT ( 'NONE',  ( -9.642888182262618425E-18, -0.3818897636720003930, -0.1574803149606299191 ) ) ;
#45667=CARTESIAN_POINT ( 'NONE',  ( -0.1787899950787401604, -1.543307086560409713, -0.07405724077823318263 ) ) ;
#45674=CARTESIAN_POINT ( 'NONE',  ( 0.1519342447269234064, 0.1255575381907582666, -0.05895817643753602233 ) ) ;
#45676=CARTESIAN_POINT ( 'NONE',  ( 0.1787899950787401604, -0.7422499524812067317, -0.07405724077823318263 ) ) ;
#45678=CARTESIAN_POINT ( 'NONE',  ( -0.09427829952974546568, -0.08956099458637047095, -0.1542373040544813001 ) ) ;
#45686=CARTESIAN_POINT ( 'NONE',  ( 0.07405724077823318263, -1.528543307032852239, 0.1787899950787401604 ) ) ;
#45693=CARTESIAN_POINT ( 'NONE',  ( -0.1797182628040039087, -0.7121501087956446652, -0.07444174185955065859 ) ) ;
#45697=CARTESIAN_POINT ( 'NONE',  ( 0.1574803149606300301, -0.4827755905511812440, 0.06523048226347956391 ) ) ;
#45708=CARTESIAN_POINT ( 'NONE',  ( 0.1574803149606300301, -0.5861220471365676810, -0.06523048226347956391 ) ) ;
#45713=CARTESIAN_POINT ( 'NONE',  ( -0.1787899950787401604, -0.4753937007336378473, -0.07405724077823318263 ) ) ;
#45714=ORIENTED_EDGE ( 'NONE', *, *, #28957, .T. ) ;
#45718=CARTESIAN_POINT ( 'NONE',  ( -0.05729443792182730560, 0.07836113345104929462, -0.2523541117089064811 ) ) ;
#45720=CARTESIAN_POINT ( 'NONE',  ( -0.07405724077823318263, -1.646653543253324026, 0.1787899950787401604 ) ) ;
#45721=CARTESIAN_POINT ( 'NONE',  ( -0.1787899950787401604, -0.8740157479777336258, -0.07405724077823318263 ) ) ;
#45722=CARTESIAN_POINT ( 'NONE',  ( -0.1574803149606300301, -1.368602362204723866, -0.06523048226347956391 ) ) ;
#45731=CARTESIAN_POINT ( 'NONE',  ( -0.1113553986120547346, -1.361220472333417364, -0.1113553986120547346 ) ) ;
#45743=CARTESIAN_POINT ( 'NONE',  ( -0.1631888523359988907, 0.09129006187719393428, 0.1912159430412066763 ) ) ;
#45747=CARTESIAN_POINT ( 'NONE',  ( -0.06405282830903208380, -0.09842519685039370636, 0.2182790088969204789 ) ) ;
#45751=CARTESIAN_POINT ( 'NONE',  ( 0.1787899950787401604, -1.090551181048598606, 0.07405724077823318263 ) ) ;
#45752=CARTESIAN_POINT ( 'NONE',  ( 0.1264236179284866091, -1.166830708607653477, 0.1264236179284866091 ) ) ;
#45756=CARTESIAN_POINT ( 'NONE',  ( 0.1797182628040039087, -0.4513233371421007667, -0.07444174185955065859 ) ) ;
#45757=CARTESIAN_POINT ( 'NONE',  ( 2.892866454678787531E-17, -1.818897637687747926, 0.1574803149606299191 ) ) ;
#45759=CARTESIAN_POINT ( 'NONE',  ( -0.1113553986120547346, -0.07185039370078739884, -0.1113553986120547346 ) ) ;
#45767=CARTESIAN_POINT ( 'NONE',  ( -9.642888182262618425E-18, -0.9724409447743621593, -0.1574803149606299191 ) ) ;
#45768=CARTESIAN_POINT ( 'NONE',  ( -0.1787899950787401604, -0.3966535432533230265, 0.07405724077823318263 ) ) ;
#45770=CARTESIAN_POINT ( 'NONE',  ( 0.1787899950787401604, -1.435039370024976391, -0.07405724077823318263 ) ) ;
#45779=CARTESIAN_POINT ( 'NONE',  ( -9.642888182262618425E-18, -1.248031495955464365, -0.1574803149606299191 ) ) ;
#45787=CARTESIAN_POINT ( 'NONE',  ( 0.1351206911648761555, -0.09842519685039370636, 0.2074211034490122396 ) ) ;
#45789=CARTESIAN_POINT ( 'NONE',  ( 0.1574803149606300301, -0.08907480314960623813, 0.06523048226347956391 ) ) ;
#45794=CARTESIAN_POINT ( 'NONE',  ( -0.1637895306277413476, -0.09851385224194922352, 0.1653590908675625915 ) ) ;
#45798=CARTESIAN_POINT ( 'NONE',  ( -1.094772975963752103E-17, -1.561639716260734279, -0.1787899950787401882 ) ) ;
#45801=CARTESIAN_POINT ( 'NONE',  ( 0.1787899950787401604, -0.5688976377415115859, -0.07405724077823318263 ) ) ;
#45807=CARTESIAN_POINT ( 'NONE',  ( 0.1264236179284866091, -0.3351377952218271283, -0.1264236179284866091 ) ) ;
#45812=CARTESIAN_POINT ( 'NONE',  ( 0.1787899950787401604, 0.08452170106209991318, -0.07405724077823318263 ) ) ;
#45813=CARTESIAN_POINT ( 'NONE',  ( 0.1787899950787401604, 0.1299212598962831977, 0.07405724077823318263 ) ) ;
#45819=CARTESIAN_POINT ( 'NONE',  ( -0.1113553986120547346, -0.9675196850393701364, 0.1113553986120547346 ) ) ;
#45821=CARTESIAN_POINT ( 'NONE',  ( -0.1797182628040039087, -1.652110738716903615, 0.07444174185955065859 ) ) ;
#45823=CARTESIAN_POINT ( 'NONE',  ( 0.1264236179284866091, -0.3400590550643468601, 0.1264236179284866091 ) ) ;
#45832=CARTESIAN_POINT ( 'NONE',  ( -0.1264236179284866091, 0.06840551186478720236, -0.1264236179284866091 ) ) ;
#45846=CARTESIAN_POINT ( 'NONE',  ( -0.07405724077823318263, -1.351377952702143004, -0.1787899950787401604 ) ) ;
#45857=CARTESIAN_POINT ( 'NONE',  ( 0.07405724077823318263, 0.1003937008411650705, -0.1787899950787401604 ) ) ;
#45859=CARTESIAN_POINT ( 'NONE',  ( 2.892866454678787531E-17, -0.2440944880814492068, 0.1574803149606299191 ) ) ;
#45865=CARTESIAN_POINT ( 'NONE',  ( -0.1787899950787401604, -1.116265700512703907, 0.07405724077823318263 ) ) ;
#45867=CARTESIAN_POINT ( 'NONE',  ( 3.284318927891251994E-17, -0.1481299212060791237, 0.1787899950787401882 ) ) ;
#45877=CARTESIAN_POINT ( 'NONE',  ( -1.094772975963752103E-17, -0.6058070865604094912, -0.1787899950787401882 ) ) ;
#45881=CARTESIAN_POINT ( 'NONE',  ( -1.100456976456230270E-17, -1.152602864701155472, -0.1797182628040039365 ) ) ;
#45898=CARTESIAN_POINT ( 'NONE',  ( -0.1574803149606300301, -1.634350393593259954, -0.06523048226347956391 ) ) ;
#45902=CARTESIAN_POINT ( 'NONE',  ( 0.06175619828060092270, -0.08093302715463278341, 0.2497778431879231764 ) ) ;
#45903=CARTESIAN_POINT ( 'NONE',  ( 0.1787899950787401604, 0.06102362210100767403, -0.07405724077823318263 ) ) ;
#45908=CARTESIAN_POINT ( 'NONE',  ( -0.07975836855958619298, 0.08959396230938611316, 0.2393845553081392907 ) ) ;
#45912=CARTESIAN_POINT ( 'NONE',  ( -0.1264236179284866091, -1.624507873961984261, -0.1264236179284866091 ) ) ;
#45919=CARTESIAN_POINT ( 'NONE',  ( 0.1531955819909203431, 0.1251005666653343951, -0.05420542381351567407 ) ) ;
#45921=CARTESIAN_POINT ( 'NONE',  ( -0.1787899950787401604, -0.6487460154733331041, -0.07405724077823318263 ) ) ;
#45923=CARTESIAN_POINT ( 'NONE',  ( 0.1979248385815023659, -0.08956033625505079032, 0.06050146127649999594 ) ) ;
#45935=AXIS2_PLACEMENT_3D ( 'NONE', #5118, #31499, #38676 ) ;
#45941=CARTESIAN_POINT ( 'NONE',  ( -0.07444174185955065859, -0.7416776678507621678, 0.1797182628040039087 ) ) ;
#45944=CARTESIAN_POINT ( 'NONE',  ( -0.1113553986120547346, -0.4557086614173228578, 0.1113553986120547346 ) ) ;
#45947=CARTESIAN_POINT ( 'NONE',  ( 0.06523048226347956391, 0.03887795275590551908, -0.1574803149606300301 ) ) ;
#45955=CARTESIAN_POINT ( 'NONE',  ( 3.284318927891251994E-17, -0.5024606298674960669, 0.1787899950787401882 ) ) ;
#45960=CARTESIAN_POINT ( 'NONE',  ( -0.1264236179284866091, -1.688484251914740275, 0.1264236179284866091 ) ) ;
#45961=CARTESIAN_POINT ( 'NONE',  ( 0.07405724077823318263, -1.120078740103715997, -0.1787899950787401604 ) ) ;
#45962=CARTESIAN_POINT ( 'NONE',  ( 0.1574803149606300301, -1.427657480314961091, 0.06523048226347956391 ) ) ;
#45969=CARTESIAN_POINT ( 'NONE',  ( 0.06523048226347956391, -1.368602362097198322, -0.1574803149606300301 ) ) ;
#45979=CARTESIAN_POINT ( 'NONE',  ( -0.2372856289813495834, 0.04209688371797420947, -0.1484361490989300203 ) ) ;
#45981=CARTESIAN_POINT ( 'NONE',  ( -0.1877875577363922188, 0.07959431159475777173, 0.1770138738565733005 ) ) ;
#45984=CARTESIAN_POINT ( 'NONE',  ( -0.1787899950787401604, -0.2501239682292389355, 0.07405724077823318263 ) ) ;
#45987=CARTESIAN_POINT ( 'NONE',  ( 0.1829792162757791496, -0.09842519685039370636, 0.1095673765095881852 ) ) ;
#45994=CARTESIAN_POINT ( 'NONE',  ( -0.1787899950787401604, -0.9872047243556864027, 0.07405724077823318263 ) ) ;
#45995=CARTESIAN_POINT ( 'NONE',  ( -0.1264236179284866091, -1.225885826717889815, -0.1264236179284866091 ) ) ;
#45998=( LENGTH_UNIT ( ) NAMED_UNIT ( * ) SI_UNIT ( $, .METRE. ) ) ;
#46002=CARTESIAN_POINT ( 'NONE',  ( -0.1574803149606297803, 0.01427165354330708555, 0.06523048226347956391 ) ) ;
#46013=CARTESIAN_POINT ( 'NONE',  ( -0.07405724077823318263, -0.5246062991588343882, -0.1787899950787401604 ) ) ;
#46014=CARTESIAN_POINT ( 'NONE',  ( -0.1787899950787401882, -1.378444881836000002, 0.000000000000000000 ) ) ;
#46019=DIRECTION ( 'NONE',  ( 0.000000000000000000, 0.000000000000000000, 1.000000000000000000 ) ) ;
#46020=CARTESIAN_POINT ( 'NONE',  ( -0.06523048226347956391, -1.230807086506645387, 0.1574803149606297803 ) ) ;
#46026=CARTESIAN_POINT ( 'NONE',  ( 0.1908307771205106085, -0.07780576619185783360, 0.1752568734204135448 ) ) ;
#46030=ORIENTED_EDGE ( 'NONE', *, *, #8765, .F. ) ;
#46034=CARTESIAN_POINT ( 'NONE',  ( 0.2067241386142287252, -0.09851384623809882057, 0.03057894068402287543 ) ) ;
#46039=EDGE_CURVE ( 'NONE', #34797, #30178, #24478, .T. ) ;
#46040=CARTESIAN_POINT ( 'NONE',  ( 0.07405724077823318263, -1.539494046969397623, 0.1787899950787401604 ) ) ;
#46043=CARTESIAN_POINT ( 'NONE',  ( -0.1264236179284866091, -0.6254921259304881964, 0.1264236179284866091 ) ) ;
#46047=CARTESIAN_POINT ( 'NONE',  ( 0.07405724077823318263, -0.3326771653005671237, -0.1787899950787401604 ) ) ;
#46048=CARTESIAN_POINT ( 'NONE',  ( -0.1264236179284866091, -0.7829724408911181710, 0.1264236179284866091 ) ) ;
#46052=CARTESIAN_POINT ( 'NONE',  ( -0.07405724077823318263, 0.01562406326682424552, -0.1787899950787401604 ) ) ;
#46059=CARTESIAN_POINT ( 'NONE',  ( -0.06523048226347956391, -0.9404527559055111396, -0.1574803149606300301 ) ) ;
#46061=CARTESIAN_POINT ( 'NONE',  ( -0.1797182628040039087, -1.612740659976745539, 0.07444174185955065859 ) ) ;
#46063=CARTESIAN_POINT ( 'NONE',  ( -0.1574803149606299191, -0.4507874014672755836, 0.000000000000000000 ) ) ;
#46064=CARTESIAN_POINT ( 'NONE',  ( -0.07405724077823318263, -0.3868110235682837295, 0.1787899950787401604 ) ) ;
#46074=CARTESIAN_POINT ( 'NONE',  ( -0.1574803149606297803, -0.8420275589475905154, 0.06523048226347956391 ) ) ;
#46075=CARTESIAN_POINT ( 'NONE',  ( -1.094772975963752103E-17, -0.05462598419820496182, -0.1787899950787401882 ) ) ;
#46077=CARTESIAN_POINT ( 'NONE',  ( -0.1264236179284866091, -0.8617125983714329918, 0.1264236179284866091 ) ) ;
#46083=CARTESIAN_POINT ( 'NONE',  ( -0.1264236179284866091, -1.348917322780881944, -0.1264236179284866091 ) ) ;
#46105=CARTESIAN_POINT ( 'NONE',  ( 0.07405724077823318263, -1.185163338307979597, 0.1787899950787401604 ) ) ;
#46107=CARTESIAN_POINT ( 'NONE',  ( -0.07405724077823318263, -0.07185039364702387743, 0.1787899950787401604 ) ) ;
#46117=CARTESIAN_POINT ( 'NONE',  ( 0.1264236179284866091, -0.6894685038832439883, -0.1264236179284866091 ) ) ;
#46120=CARTESIAN_POINT ( 'NONE',  ( -1.100456976456230270E-17, -1.191972943441313104, -0.1797182628040039365 ) ) ;
#46128=CARTESIAN_POINT ( 'NONE',  ( -0.1574803149606297803, -0.7239173227271186173, 0.06523048226347956391 ) ) ;
#46140=CARTESIAN_POINT ( 'NONE',  ( -9.642888182262618425E-18, -1.011811023514519681, -0.1574803149606299191 ) ) ;
#46142=CARTESIAN_POINT ( 'NONE',  ( 0.1264236179284866091, -0.09399606293836260118, -0.1264236179284866091 ) ) ;
#46146=CARTESIAN_POINT ( 'NONE',  ( 0.1264236179284866091, 0.1028543307624250058, -0.1264236179284866091 ) ) ;
#46155=CARTESIAN_POINT ( 'NONE',  ( 0.1264236179284866091, -1.713090551127338657, -0.1264236179284866091 ) ) ;
#46161=CARTESIAN_POINT ( 'NONE',  ( 0.1489248948074351209, 0.1264776978674661545, -0.06844634442982192035 ) ) ;
#46163=CARTESIAN_POINT ( 'NONE',  ( -0.1787899950787401882, -0.6462853855520729329, 0.000000000000000000 ) ) ;
#46165=CARTESIAN_POINT ( 'NONE',  ( 0.05163519342973015708, -0.08956075397208444755, -0.1825432363577885742 ) ) ;
#46166=PLANE ( 'NONE',  #17990 ) ;
#46167=VERTEX_POINT ( 'NONE', #33896 ) ;
#46180=CARTESIAN_POINT ( 'NONE',  ( -0.1113553986120547346, -0.5049212598425196763, -0.1113553986120547346 ) ) ;
#46187=CARTESIAN_POINT ( 'NONE',  ( 0.06523048226347956391, 0.08809055128862933182, -0.1574803149606297803 ) ) ;
#46194=CARTESIAN_POINT ( 'NONE',  ( 0.1264236179284866091, -0.5762795275052914334, 0.1264236179284866091 ) ) ;
#46199=CARTESIAN_POINT ( 'NONE',  ( -0.06179214533979354718, 0.08095196624129316620, -0.2497573591204075849 ) ) ;
#46201=CARTESIAN_POINT ( 'NONE',  ( 0.07444174185955046430, 0.1047790250626238068, -0.1797182628040039087 ) ) ;
#46202=CARTESIAN_POINT ( 'NONE',  ( -0.1787899950787401882, -0.9896653542769447975, 0.000000000000000000 ) ) ;
#46203=CARTESIAN_POINT ( 'NONE',  ( -0.1113553986120547346, -1.361220472440944906, 0.1113553986120547346 ) ) ;
#46214=CARTESIAN_POINT ( 'NONE',  ( -0.2471922904502826812, 0.03219022224904098672, -0.1427165354330708902 ) ) ;
#46219=CARTESIAN_POINT ( 'NONE',  ( 0.1787899950787401604, -0.2304389288591599250, -0.07405724077823318263 ) ) ;
#46220=CARTESIAN_POINT ( 'NONE',  ( 0.2066882016312708570, -0.09842519685039370636, 0.03057550915391468727 ) ) ;
#46226=CARTESIAN_POINT ( 'NONE',  ( -0.1787899950787401604, -1.223425196796630532, -0.07405724077823318263 ) ) ;
#46228=CARTESIAN_POINT ( 'NONE',  ( 0.07444174185955065859, -0.5005359355672972521, 0.1797182628040039087 ) ) ;
#46232=CARTESIAN_POINT ( 'NONE',  ( 0.1574803149606300301, 0.07332677165354323234, -0.06523048226347956391 ) ) ;
#46247=CARTESIAN_POINT ( 'NONE',  ( -0.07405724077823318263, -0.6279527558517482566, 0.1787899950787401604 ) ) ;
#46248=CARTESIAN_POINT ( 'NONE',  ( 0.07405724077823318263, -1.366141732229700478, 0.1787899950787401604 ) ) ;
#46257=CYLINDRICAL_SURFACE ( 'NONE', #36694, 0.1574803149606299191 ) ;
#46258=CARTESIAN_POINT ( 'NONE',  ( -0.1574803149606297803, -1.275098425089322696, 0.06523048226347956391 ) ) ;
#46261=CARTESIAN_POINT ( 'NONE',  ( 0.08577540572602856961, -0.09842547777292044719, -0.1568821689687208421 ) ) ;
#46265=DIRECTION ( 'NONE',  ( 0.000000000000000000, 0.000000000000000000, 1.000000000000000000 ) ) ;
#46273=CARTESIAN_POINT ( 'NONE',  ( 0.2033951071932515731, -0.09851384550996260259, -0.03145358857524988005 ) ) ;
#46282=CARTESIAN_POINT ( 'NONE',  ( 0.1787899950787401604, -0.6476377952218281830, -0.07405724077823318263 ) ) ;
#46286=CARTESIAN_POINT ( 'NONE',  ( -0.07405724077823318263, -0.3129921259304885850, 0.1787899950787401604 ) ) ;
#46287=CARTESIAN_POINT ( 'NONE',  ( -0.1264236179284866091, -0.7928149605761574126, -0.1264236179284866091 ) ) ;
#46291=CARTESIAN_POINT ( 'NONE',  ( 0.1264236179284866091, 0.08698233098335965419, -0.1264236179284866091 ) ) ;
#46292=CARTESIAN_POINT ( 'NONE',  ( 0.1264236179284866091, 0.01919291343959031448, -0.1264236179284866091 ) ) ;
#46298=CARTESIAN_POINT ( 'NONE',  ( -0.1574803149606297803, -0.8518700787401587426, 0.06523048226347956391 ) ) ;
#46300=CARTESIAN_POINT ( 'NONE',  ( -0.07444174185955065859, -1.661953258401944300, -0.1797182628040039087 ) ) ;
#46302=CARTESIAN_POINT ( 'NONE',  ( -0.1574803149606300301, -0.4926181101286939423, -0.06523048226347956391 ) ) ;
#46303=AXIS2_PLACEMENT_3D ( 'NONE', #7856, #22474, #33528 ) ;
#46306=CARTESIAN_POINT ( 'NONE',  ( 0.1528720448724809056, 0.09445537554013616610, -0.1971723546074463096 ) ) ;
#46311=CARTESIAN_POINT ( 'NONE',  ( -0.1235961452251415349, -0.09842519685039370636, -0.2140748031496062798 ) ) ;
#46316=CARTESIAN_POINT ( 'NONE',  ( -0.1113553986120547346, -0.8887795274515276622, -0.1113553986120547346 ) ) ;
#46317=CARTESIAN_POINT ( 'NONE',  ( 0.1264236179284866091, -0.1776574802611972648, -0.1264236179284866091 ) ) ;
#46319=CARTESIAN_POINT ( 'NONE',  ( -0.1787899950787401604, -0.8641732282926931630, 0.07405724077823318263 ) ) ;
#46337=CARTESIAN_POINT ( 'NONE',  ( -0.2471922904502826812, 0.09123121687245379363, -0.04590630800384516014 ) ) ;
#46339=CARTESIAN_POINT ( 'NONE',  ( -0.07405724077823318263, -1.111344440670184897, 0.1787899950787401604 ) ) ;
#46341=CARTESIAN_POINT ( 'NONE',  ( -0.07405724077823318263, -0.1653543306548978520, -0.1787899950787401604 ) ) ;
#46350=CARTESIAN_POINT ( 'NONE',  ( -0.07444174185955065859, -0.1904965654885572290, 0.1797182628040039087 ) ) ;
#46351=CARTESIAN_POINT ( 'NONE',  ( 0.1264236179284866091, -0.8075787401037164415, -0.1264236179284866091 ) ) ;
#46354=CARTESIAN_POINT ( 'NONE',  ( 0.07444174185955065859, -1.327307589110604980, 0.1797182628040039087 ) ) ;
#46367=CARTESIAN_POINT ( 'NONE',  ( 0.1787899950787401604, -0.01771653537930737918, -0.07405724077823318263 ) ) ;
#46382=CARTESIAN_POINT ( 'NONE',  ( -0.1264236179284866091, -0.03494094482812625663, 0.1264236179284866091 ) ) ;
#46390=CARTESIAN_POINT ( 'NONE',  ( -0.1574803149606297803, -0.4089566928058585571, 0.06523048226347956391 ) ) ;
#46391=CARTESIAN_POINT ( 'NONE',  ( 0.1264236179284866091, -1.762303149552535642, 0.1264236179284866091 ) ) ;
#46411=CARTESIAN_POINT ( 'NONE',  ( 0.1270800023317771588, -0.6949256993468247989, 0.1270800023317771588 ) ) ;
#46412=CARTESIAN_POINT ( 'NONE',  ( 0.2471922904502826257, 0.09379707428445177575, 0.03645092102367950004 ) ) ;
#46415=CARTESIAN_POINT ( 'NONE',  ( 0.1574803149606299191, -0.5590551181102362266, -1.928577636452523993E-17 ) ) ;
#46424=CARTESIAN_POINT ( 'NONE',  ( -0.1574803149606297803, -0.6058070865066461641, 0.06523048226347956391 ) ) ;
#46428=CARTESIAN_POINT ( 'NONE',  ( 0.1429759811007342563, 0.1299212598425197041, 0.1098622232965498907 ) ) ;
#46431=CARTESIAN_POINT ( 'NONE',  ( 0.000000000000000000, 0.1102362204724409434, -0.2204724409448818867 ) ) ;
#46432=CARTESIAN_POINT ( 'NONE',  ( -0.1787899950787401882, -1.811515747977732405, 0.000000000000000000 ) ) ;
#46433=CARTESIAN_POINT ( 'NONE',  ( -0.1264236179284866091, -1.024114173174582643, 0.1264236179284866091 ) ) ;
#46434=CARTESIAN_POINT ( 'NONE',  ( -0.1113553986120547346, -1.479330708661417360, 0.1113553986120547346 ) ) ;
#46442=CARTESIAN_POINT ( 'NONE',  ( -0.1574803149606299191, -1.435039369971212508, 0.000000000000000000 ) ) ;
#46445=DIRECTION ( 'NONE',  ( 0.000000000000000000, -1.000000000000000000, 0.000000000000000000 ) ) ;
#46448=CARTESIAN_POINT ( 'NONE',  ( -0.2471922904502826257, 0.07780974138651210181, 0.07762775726530198039 ) ) ;
#46452=CARTESIAN_POINT ( 'NONE',  ( -0.1264236179284866091, -0.2870334170481366187, 0.1264236179284866091 ) ) ;
#46453=CARTESIAN_POINT ( 'NONE',  ( 0.1430309448599517697, -0.09842519685039370636, -0.1381503230155334827 ) ) ;
#46462=CARTESIAN_POINT ( 'NONE',  ( 0.07405724077823318263, -1.120078740103715997, -0.1787899950787401604 ) ) ;
#46463=CARTESIAN_POINT ( 'NONE',  ( -1.094772975963752103E-17, -1.230807086560409269, -0.1787899950787401882 ) ) ;
#46465=LENGTH_MEASURE_WITH_UNIT ( LENGTH_MEASURE( 0.02539999999999999897 ), #45998 ) ;
#46466=CARTESIAN_POINT ( 'NONE',  ( -0.1797182628040039087, -0.5546697938350136914, -0.07444174185955065859 ) ) ;
#46470=CARTESIAN_POINT ( 'NONE',  ( -0.06523048226347956391, -0.1530511811023622937, -0.1574803149606300301 ) ) ;
#46476=CARTESIAN_POINT ( 'NONE',  ( -9.642888182262618425E-18, -0.07677165354330708902, -0.1574803149606299191 ) ) ;
#46479=DIRECTION ( 'NONE',  ( 0.000000000000000000, 1.000000000000000000, 0.000000000000000000 ) ) ;
#46484=CARTESIAN_POINT ( 'NONE',  ( 0.1264236179284866091, -0.6107283464029291675, -0.1264236179284866091 ) ) ;
#46485=CARTESIAN_POINT ( 'NONE',  ( -0.1787899950787401604, -1.420275590497418250, -0.07405724077823318263 ) ) ;
#46493=CARTESIAN_POINT ( 'NONE',  ( -0.1113553986120547346, -1.282480314853102321, -0.1113553986120547346 ) ) ;
#46496=CARTESIAN_POINT ( 'NONE',  ( 0.1585082349939047064, -0.09842394368956142170, -0.08275592341139960395 ) ) ;
#46507=CARTESIAN_POINT ( 'NONE',  ( 0.1830111034970090533, -0.09851384631394094482, 0.1095843003117216580 ) ) ;
#46514=CARTESIAN_POINT ( 'NONE',  ( 0.07405724077823318263, -1.682210582402467791, -0.1787899950787401604 ) ) ;
#46515=CARTESIAN_POINT ( 'NONE',  ( 3.284318927891251994E-17, -0.6599409448281259305, 0.1787899950787401882 ) ) ;
#46521=CARTESIAN_POINT ( 'NONE',  ( -0.1787899950787401604, -0.7460629920722210429, 0.07405724077823318263 ) ) ;
#46526=CARTESIAN_POINT ( 'NONE',  ( -0.1264236179284866091, -0.01144286586703399666, 0.1264236179284866091 ) ) ;
#46527=CARTESIAN_POINT ( 'NONE',  ( -0.1787899950787401604, 0.03149606304588949135, -0.07405724077823318263 ) ) ;
#46532=CARTESIAN_POINT ( 'NONE',  ( -0.1574803149606297803, -0.8912401574803148208, 0.06523048226347956391 ) ) ;
#46534=CARTESIAN_POINT ( 'NONE',  ( -0.1797182628040039087, -1.696402077299580702, -0.07444174185955065859 ) ) ;
#46538=CARTESIAN_POINT ( 'NONE',  ( -9.642888182262618425E-18, 0.001968503937007873988, -0.1574803149606299191 ) ) ;
#46543=CARTESIAN_POINT ( 'NONE',  ( -0.07405724077823318263, -0.1161417322297011862, 0.1787899950787401604 ) ) ;
#46545=CARTESIAN_POINT ( 'NONE',  ( -0.1787899950787401604, -0.9478346456155283262, -0.07405724077823318263 ) ) ;
#46565=CARTESIAN_POINT ( 'NONE',  ( -0.1787899950787401604, 0.1151574803687242243, 0.07405724077823318263 ) ) ;
#46566=ORIENTED_EDGE ( 'NONE', *, *, #36802, .T. ) ;
#46570=CARTESIAN_POINT ( 'NONE',  ( 0.1787899950787401882, -1.476870078686393750, -2.189545951927503898E-17 ) ) ;
#46574=CARTESIAN_POINT ( 'NONE',  ( -0.07405724077823318263, -1.204848377678058524, -0.1787899950787401604 ) ) ;
#46576=CARTESIAN_POINT ( 'NONE',  ( 0.07405724077823318263, -0.09153543301710270752, -0.1787899950787401604 ) ) ;
#46585=CARTESIAN_POINT ( 'NONE',  ( 0.1264236179284866091, -1.555610236166708571, -0.1264236179284866091 ) ) ;
#46597=CARTESIAN_POINT ( 'NONE',  ( 2.892866454678787531E-17, -0.7559055117034961802, 0.1574803149606299191 ) ) ;
#46599=CARTESIAN_POINT ( 'NONE',  ( 0.07405724077823318263, 0.01181102367581074800, 0.1787899950787401604 ) ) ;
#46609=VERTEX_POINT ( 'NONE', #46755 ) ;
#46613=CARTESIAN_POINT ( 'NONE',  ( -0.1787899950787401604, 0.001968503990771383692, 0.07405724077823318263 ) ) ;
#46623=CARTESIAN_POINT ( 'NONE',  ( 0.1787899950787401604, -1.676181102308441639, -0.07405724077823318263 ) ) ;
#46631=CARTESIAN_POINT ( 'NONE',  ( -0.1787899950787401882, -0.7250255430323878647, 0.000000000000000000 ) ) ;
#46633=CARTESIAN_POINT ( 'NONE',  ( -0.1570894919835442993, -0.08956159021719448110, 0.05351830911520212564 ) ) ;
#46645=CARTESIAN_POINT ( 'NONE',  ( -0.1797182628040039365, -0.7884296363546987596, 0.000000000000000000 ) ) ;
#46649=CARTESIAN_POINT ( 'NONE',  ( 0.06523048226347956391, -0.5516732283464562681, -0.1574803149606300301 ) ) ;
#46651=VERTEX_POINT ( 'NONE', #32655 ) ;
#46667=CYLINDRICAL_SURFACE ( 'NONE', #35021, 0.1574803149606299191 ) ;
#46668=CARTESIAN_POINT ( 'NONE',  ( -0.1797182628040039087, 0.07525146600750569348, -0.07444174185955065859 ) ) ;
#46669=CARTESIAN_POINT ( 'NONE',  ( -0.07405724077823318263, -1.061023621993481214, 0.1787899950787401604 ) ) ;
#46670=CARTESIAN_POINT ( 'NONE',  ( 0.1574803149606300301, -1.580216535433071723, -0.06523048226347956391 ) ) ;
#46675=ORIENTED_EDGE ( 'NONE', *, *, #35064, .F. ) ;
#46695=CARTESIAN_POINT ( 'NONE',  ( 3.284318927891251994E-17, -1.255413385773007873, 0.1787899950787401882 ) ) ;
#46696=CARTESIAN_POINT ( 'NONE',  ( -0.1264236179284866091, -1.452263779473795369, 0.1264236179284866091 ) ) ;
#46697=CARTESIAN_POINT ( 'NONE',  ( 0.000000000000000000, 0.09842519685039370636, 0.000000000000000000 ) ) ;
#46698=CARTESIAN_POINT ( 'NONE',  ( -0.07444174185955065859, -0.6383312111578482995, -0.1797182628040039087 ) ) ;
#46702=CARTESIAN_POINT ( 'NONE',  ( 0.1113553986120547346, -0.2096456692913385711, 0.1113553986120547346 ) ) ;
#46716=CARTESIAN_POINT ( 'NONE',  ( -9.642888182262618425E-18, -0.07677165354330708902, -0.1574803149606299191 ) ) ;
#46718=CARTESIAN_POINT ( 'NONE',  ( 0.1264236179284866091, -0.5418307086076535883, 0.1264236179284866091 ) ) ;
#46720=CARTESIAN_POINT ( 'NONE',  ( -0.06523048226347956391, -1.122539370078741827, 0.1574803149606297803 ) ) ;
#46736=FACE_OUTER_BOUND ( 'NONE', #40665, .T. ) ;
#46739=CARTESIAN_POINT ( 'NONE',  ( -0.1113553986120547346, -0.2194881888688507976, -0.1113553986120547346 ) ) ;
#46743=CARTESIAN_POINT ( 'NONE',  ( -0.1729752768006175279, -0.09851383664320945144, -0.02639418254170881883 ) ) ;
#46744=EDGE_LOOP ( 'NONE', ( #16065, #43527, #36349, #13937 ) ) ;
#46749=CARTESIAN_POINT ( 'NONE',  ( -0.1264236179284866091, -1.664986172953647925, 0.1264236179284866091 ) ) ;
#46750=ORIENTED_EDGE ( 'NONE', *, *, #33255, .T. ) ;
#46755=CARTESIAN_POINT ( 'NONE',  ( -9.642888182262618425E-18, 0.08070866141732284393, -0.1574803149606299191 ) ) ;
#46756=CARTESIAN_POINT ( 'NONE',  ( -0.1787899950787401604, -0.2785433070328505734, 0.07405724077823318263 ) ) ;
#46757=CARTESIAN_POINT ( 'NONE',  ( 0.1264236179284866091, -0.7731299212060788184, 0.1264236179284866091 ) ) ;
#46759=DIRECTION ( 'NONE',  ( 0.000000000000000000, 1.000000000000000000, 0.000000000000000000 ) ) ;
#46761=CARTESIAN_POINT ( 'NONE',  ( 0.1264236179284866091, -0.07049798397727027877, -0.1264236179284866091 ) ) ;
#46762=CARTESIAN_POINT ( 'NONE',  ( -0.1264236179284866091, -0.2317913385289138151, 0.1264236179284866091 ) ) ;
#46763=CARTESIAN_POINT ( 'NONE',  ( 0.1787899950787401604, 0.05610236225848794223, -0.07405724077823318263 ) ) ;
#46764=CARTESIAN_POINT ( 'NONE',  ( 0.02970261290376345273, -0.09842519685039373412, 0.1606413281782796409 ) ) ;
#46769=CARTESIAN_POINT ( 'NONE',  ( 0.07444174185955065859, -1.760378455252336938, 0.1797182628040039087 ) ) ;
#46770=CARTESIAN_POINT ( 'NONE',  ( -0.1264236179284866091, -0.4286417322297008115, 0.1264236179284866091 ) ) ;
#46773=CARTESIAN_POINT ( 'NONE',  ( 0.1894960330211038768, 0.07859832706092066690, -0.1760274851910411664 ) ) ;
#46776=CARTESIAN_POINT ( 'NONE',  ( -0.1675084398163183552, -0.08956740676313401650, -0.1887210895732543414 ) ) ;
#46779=CARTESIAN_POINT ( 'NONE',  ( -0.06523048226347956391, -0.8912401573727871673, -0.1574803149606300301 ) ) ;
#46780=CARTESIAN_POINT ( 'NONE',  ( 3.284318927891251994E-17, -0.07431102356828367395, 0.1787899950787401882 ) ) ;
#46782=CARTESIAN_POINT ( 'NONE',  ( -0.1787899950787401882, -1.102854330654897685, 0.000000000000000000 ) ) ;
#46805=CARTESIAN_POINT ( 'NONE',  ( 0.1264236179284866091, 0.04872047249470835839, 0.1264236179284866091 ) ) ;
#46811=CARTESIAN_POINT ( 'NONE',  ( 0.1787899950787401604, -1.293431054843413142, -0.07405724077823318263 ) ) ;
#46813=CARTESIAN_POINT ( 'NONE',  ( -0.07405724077823318263, -0.2687007873478113318, 0.1787899950787401604 ) ) ;
#46821=CARTESIAN_POINT ( 'NONE',  ( -0.1787899950787401604, -1.503937007820251637, -0.07405724077823318263 ) ) ;
#46822=CARTESIAN_POINT ( 'NONE',  ( -0.1264236179284866091, -0.7878937007336378473, 0.1264236179284866091 ) ) ;
#46824=CARTESIAN_POINT ( 'NONE',  ( -0.1797182628040039087, -1.297780030055485589, 0.07444174185955065859 ) ) ;
#46850=CARTESIAN_POINT ( 'NONE',  ( -0.07405724077823318263, -0.07185039364702387743, 0.1787899950787401604 ) ) ;
#46855=CARTESIAN_POINT ( 'NONE',  ( 0.1944374611862057511, 0.07559918600398417288, 0.1731745503097384398 ) ) ;
#46860=CARTESIAN_POINT ( 'NONE',  ( -0.1787899950787401604, -1.661417322780881500, -0.07405724077823318263 ) ) ;
#46868=CARTESIAN_POINT ( 'NONE',  ( 4.801428276353606495E-17, 0.03219022224904102836, 0.2854330708661417804 ) ) ;
#46870=CARTESIAN_POINT ( 'NONE',  ( -0.1787899950787401604, -0.7619349918512856590, 0.07405724077823318263 ) ) ;
#46886=CARTESIAN_POINT ( 'NONE',  ( -0.07444174185955065859, -0.7810477465909202444, 0.1797182628040039087 ) ) ;
#46890=CARTESIAN_POINT ( 'NONE',  ( 0.1113553986120547346, -0.6328740157480314821, -0.1113553986120547346 ) ) ;
#46892=LINE ( 'NONE', #21975, #14655 ) ;
#46910=CARTESIAN_POINT ( 'NONE',  ( -0.1270800023317771588, 0.07279083608624586921, -0.1270800023317771588 ) ) ;
#46911=CARTESIAN_POINT ( 'NONE',  ( -1.094772975963752103E-17, -1.275098425143086578, -0.1787899950787401882 ) ) ;
#46912=CARTESIAN_POINT ( 'NONE',  ( -0.1574803149606299191, -1.484251968503937036, 0.000000000000000000 ) ) ;
#46925=AXIS2_PLACEMENT_3D ( 'NONE', #17194, #18074, #20316 ) ;
#46926=CARTESIAN_POINT ( 'NONE',  ( -0.1908328281150615813, 0.07780450164205222896, -0.1752556861836934432 ) ) ;
#46929=CARTESIAN_POINT ( 'NONE',  ( -0.07405724077823318263, -0.3239428658670340799, 0.1787899950787401604 ) ) ;
#46936=ORIENTED_EDGE ( 'NONE', *, *, #5061, .T. ) ;
#46940=CARTESIAN_POINT ( 'NONE',  ( -0.1787899950787401882, -1.147145669237574772, 0.000000000000000000 ) ) ;
#46941=CARTESIAN_POINT ( 'NONE',  ( 3.284318927891251994E-17, -1.368602362150960650, 0.1787899950787401882 ) ) ;
#46947=CARTESIAN_POINT ( 'NONE',  ( 2.892866454678787531E-17, -0.1358267716535433156, 0.1574803149606299191 ) ) ;
#46954=CARTESIAN_POINT ( 'NONE',  ( -0.06523048226347956391, -0.07431102362204729250, -0.1574803149606300301 ) ) ;
#46962=CARTESIAN_POINT ( 'NONE',  ( -0.1113553986120547346, 0.1053149607374482266, 0.1113553986120547346 ) ) ;
#46963=CARTESIAN_POINT ( 'NONE',  ( 2.892866454678787531E-17, -1.503937007766488199, 0.1574803149606299191 ) ) ;
#46964=CARTESIAN_POINT ( 'NONE',  ( -0.1264236179284866091, -0.6304133857730078727, 0.1264236179284866091 ) ) ;
#46965=CARTESIAN_POINT ( 'NONE',  ( 0.1113553986120547346, -1.115157480314960647, 0.1113553986120547346 ) ) ;
#46979=CARTESIAN_POINT ( 'NONE',  ( 0.1574803149606299191, -0.2736220471365672924, -1.928577636452523993E-17 ) ) ;
#46981=DIRECTION ( 'NONE',  ( 0.000000000000000000, 1.000000000000000000, 0.000000000000000000 ) ) ;
#46985=CARTESIAN_POINT ( 'NONE',  ( -0.1604542604227535418, -0.09851383291672559384, 0.05492199793948401854 ) ) ;
#46990=CARTESIAN_POINT ( 'NONE',  ( 3.284318927891251994E-17, -1.738805070591442847, 0.1787899950787401882 ) ) ;
#46995=CARTESIAN_POINT ( 'NONE',  ( -0.07405724077823318263, -0.8346456692375755493, -0.1787899950787401604 ) ) ;
#46996=CARTESIAN_POINT ( 'NONE',  ( -0.2471915046496347967, -0.08339338023411900502, -0.06619788746946630997 ) ) ;
#47000=CARTESIAN_POINT ( 'NONE',  ( 0.1787899950787401604, -0.07787987374104976546, 0.07405724077823318263 ) ) ;
#47001=CARTESIAN_POINT ( 'NONE',  ( -0.1787899950787401882, -0.2760826771115909573, 0.000000000000000000 ) ) ;
#47002=CARTESIAN_POINT ( 'NONE',  ( -0.1264236179284866091, -0.0004921259304884456750, 0.1264236179284866091 ) ) ;
#47004=CARTESIAN_POINT ( 'NONE',  ( 0.2471904733175533664, -0.07069887449118136824, -0.09042980707038553168 ) ) ;
#47010=CARTESIAN_POINT ( 'NONE',  ( 0.1270800023317771588, -1.748075305646037414, -0.1270800023317771588 ) ) ;
#47020=CARTESIAN_POINT ( 'NONE',  ( 0.07405724077823318263, -0.1358267715997797664, -0.1787899950787401604 ) ) ;
#47023=CARTESIAN_POINT ( 'NONE',  ( -0.1264236179284866091, -1.068405511757259951, -0.1264236179284866091 ) ) ;
#47034=CARTESIAN_POINT ( 'NONE',  ( -0.1574803149606300301, -1.161909448711369919, -0.06523048226347956391 ) ) ;
#47045=CARTESIAN_POINT ( 'NONE',  ( -0.07405724077823318263, -0.07677165348954355373, 0.1787899950787401604 ) ) ;
#47052=CARTESIAN_POINT ( 'NONE',  ( 3.284318927891251994E-17, -1.226994046969395624, 0.1787899950787401882 ) ) ;
#47054=CARTESIAN_POINT ( 'NONE',  ( 0.1264236179284866091, -0.2908464566391499861, -0.1264236179284866091 ) ) ;
#47059=CARTESIAN_POINT ( 'NONE',  ( -0.2471922711061399491, -0.07744971747242616888, 0.07831899213450065067 ) ) ;
#47065=CARTESIAN_POINT ( 'NONE',  ( 0.1264236179284866091, -1.644192913332062966, 0.1264236179284866091 ) ) ;
#47066=CARTESIAN_POINT ( 'NONE',  ( -0.1787899950787401604, -0.7165354330171036512, -0.07405724077823318263 ) ) ;
#47068=CARTESIAN_POINT ( 'NONE',  ( -0.1181206562389580106, -0.09842519685039372024, 0.1154461398689740764 ) ) ;
#47075=FACE_OUTER_BOUND ( 'NONE', #16434, .T. ) ;
#47092=CARTESIAN_POINT ( 'NONE',  ( -0.1787899950787401882, -0.03986220467064590517, 0.000000000000000000 ) ) ;
#47094=CARTESIAN_POINT ( 'NONE',  ( 2.892866454678787531E-17, -0.08661417312081949593, 0.1574803149606299191 ) ) ;
#47098=CARTESIAN_POINT ( 'NONE',  ( 0.1528784791660942888, -0.09445537554013612447, -0.1971681403756167517 ) ) ;
#47104=CARTESIAN_POINT ( 'NONE',  ( -9.642888182262618425E-18, 0.1299212599500466636, -0.1574803149606299191 ) ) ;
#47113=CARTESIAN_POINT ( 'NONE',  ( -0.1264236179284866091, -0.7988444406701832312, 0.1264236179284866091 ) ) ;
#47114=CARTESIAN_POINT ( 'NONE',  ( -0.004948818435039661207, -0.08956172228597282514, 0.1527134704424525646 ) ) ;
#47119=DIRECTION ( 'NONE',  ( 0.000000000000000000, 0.000000000000000000, 1.000000000000000000 ) ) ;
#47127=EDGE_CURVE ( 'NONE', #44436, #22067, #13936, .T. ) ;
#47134=CARTESIAN_POINT ( 'NONE',  ( -1.100456976456230270E-17, -0.9163823922602106764, -0.1797182628040039365 ) ) ;
#47138=CARTESIAN_POINT ( 'NONE',  ( -0.1113553986120547346, -0.6624015748031496509, -0.1113553986120547346 ) ) ;
#47140=CARTESIAN_POINT ( 'NONE',  ( -0.1626266311456144864, 0.1259158391802847055, -0.01719266890941318487 ) ) ;
#47145=CARTESIAN_POINT ( 'NONE',  ( -0.1235961452251413406, 0.09842519685039370636, -0.2140748031496062798 ) ) ;
#47147=CARTESIAN_POINT ( 'NONE',  ( 0.06523048226347956391, -0.6353346455617642219, 0.1574803149606297803 ) ) ;
#47150=CARTESIAN_POINT ( 'NONE',  ( -0.1787899950787401604, -0.6722440944344262315, -0.07405724077823318263 ) ) ;
#47157=CARTESIAN_POINT ( 'NONE',  ( -0.07405724077823318263, -1.272637795221826629, -0.1787899950787401604 ) ) ;
#47158=CARTESIAN_POINT ( 'NONE',  ( -0.06523048226347956391, -1.516240157480315709, 0.1574803149606297803 ) ) ;
#47159=CARTESIAN_POINT ( 'NONE',  ( -0.2471922904502826812, -0.09842519685039370636, 5.914624404477007554E-17 ) ) ;
#47164=CARTESIAN_POINT ( 'NONE',  ( 0.1264236179284866091, -1.407972440891118282, 0.1264236179284866091 ) ) ;
#47170=CARTESIAN_POINT ( 'NONE',  ( -0.1627568843983587810, 0.09133345722617068618, -0.1914653398462846101 ) ) ;
#47175=CARTESIAN_POINT ( 'NONE',  ( -0.1787899950787401604, -0.3337853855520734325, -0.07405724077823318263 ) ) ;
#47176=CARTESIAN_POINT ( 'NONE',  ( -0.1459546509031376116, -0.09842519685039370636, 0.08266691343448798190 ) ) ;
#47188=CARTESIAN_POINT ( 'NONE',  ( 0.1264236179284866091, -1.161909448765133801, -0.1264236179284866091 ) ) ;
#47189=CARTESIAN_POINT ( 'NONE',  ( 0.07405724077823318263, -1.366141732229700478, 0.1787899950787401604 ) ) ;
#47192=CARTESIAN_POINT ( 'NONE',  ( -0.07444174185955065859, -0.5989611324176910001, -0.1797182628040039087 ) ) ;
#47196=CARTESIAN_POINT ( 'NONE',  ( 0.06523048226347956391, -0.1186023622047245596, -0.1574803149606300301 ) ) ;
#47206=VERTEX_POINT ( 'NONE', #23781 ) ;
#47208=CARTESIAN_POINT ( 'NONE',  ( -0.1574803149606299191, -1.513779527451527329, 0.000000000000000000 ) ) ;
#47209=CARTESIAN_POINT ( 'NONE',  ( 0.1264236179284866091, -0.8075787401037164415, -0.1264236179284866091 ) ) ;
#47211=CARTESIAN_POINT ( 'NONE',  ( 0.1574803149606299191, -1.070866141732283339, -1.928577636452523993E-17 ) ) ;
#47227=CARTESIAN_POINT ( 'NONE',  ( -0.06523048226347956391, -0.2219488187901106635, -0.1574803149606300301 ) ) ;
#47232=CARTESIAN_POINT ( 'NONE',  ( -0.1623731327614419684, -0.09851383322942126874, 0.05011340600964842712 ) ) ;
#47240=CARTESIAN_POINT ( 'NONE',  ( 0.07405724077823318263, -0.3868110235682837295, 0.1787899950787401604 ) ) ;
#47241=( BOUNDED_CURVE ( )  B_SPLINE_CURVE ( 2, ( #32049, #39447, #2317, #27995, #6386, #10240, #38518, #42559, #13581 ),
 .UNSPECIFIED., .F., .T. ) 
 B_SPLINE_CURVE_WITH_KNOTS ( ( 3, 2, 2, 2, 3 ),
 ( 0.04499999999999999833, 0.04750000000000000056, 0.05000000000000000278, 0.05249999999999999806, 0.05500000000000000028 ),
 .UNSPECIFIED. ) 
 CURVE ( )  GEOMETRIC_REPRESENTATION_ITEM ( )  RATIONAL_B_SPLINE_CURVE ( ( 1.000000000000000000, 0.9238795325112869605, 1.000000000000000000, 0.9238795325112869605, 1.000000000000000000, 0.9238795325112869605, 1.000000000000000000, 0.9238795325112869605, 1.000000000000000000 ) ) 
 REPRESENTATION_ITEM ( '' )  ) ;
#47242=CARTESIAN_POINT ( 'NONE',  ( 0.1787899950787401604, -0.8838582676627719792, -0.07405724077823318263 ) ) ;
#47247=CARTESIAN_POINT ( 'NONE',  ( -0.1270800023317771588, -0.1535871166696596291, 0.1270800023317771588 ) ) ;
#47248=CARTESIAN_POINT ( 'NONE',  ( -1.094772975963752103E-17, -0.06557672413475058859, -0.1787899950787401882 ) ) ;
#47249=CARTESIAN_POINT ( 'NONE',  ( 0.1264236179284866091, -0.2908464566391499861, -0.1264236179284866091 ) ) ;
#47250=CARTESIAN_POINT ( 'NONE',  ( -0.07405724077823318263, -0.09153543301710270752, -0.1787899950787401604 ) ) ;
#47257=CARTESIAN_POINT ( 'NONE',  ( -0.1797182628040039087, -1.770220974937375402, 0.07444174185955065859 ) ) ;
#47264=CARTESIAN_POINT ( 'NONE',  ( 0.07405724077823318263, -0.2687007873478113318, 0.1787899950787401604 ) ) ;
#47269=CARTESIAN_POINT ( 'NONE',  ( 0.1787899950787401882, -1.004429133804503937, -2.189545951927503898E-17 ) ) ;
#47277=CARTESIAN_POINT ( 'NONE',  ( 0.1574803149606300301, -1.137303149498771537, -0.06523048226347956391 ) ) ;
#47289=CARTESIAN_POINT ( 'NONE',  ( 0.07405724077823318263, 0.02165354336085014916, -0.1787899950787401604 ) ) ;
#47299=CARTESIAN_POINT ( 'NONE',  ( 0.1787899950787401882, -1.374631842244986357, -2.189545951927503898E-17 ) ) ;
#47301=CARTESIAN_POINT ( 'NONE',  ( 0.1787899950787401882, -0.2563976377415121966, -2.189545951927503898E-17 ) ) ;
#47302=CARTESIAN_POINT ( 'NONE',  ( -0.1113553986120547346, 0.01673228357209397693, -0.1113553986120547346 ) ) ;
#47310=CARTESIAN_POINT ( 'NONE',  ( -0.07405724077823318263, -1.666338582623402953, -0.1787899950787401604 ) ) ;
#47311=CARTESIAN_POINT ( 'NONE',  ( 3.284318927891251994E-17, -1.722933070812378009, 0.1787899950787401882 ) ) ;
#47315=CARTESIAN_POINT ( 'NONE',  ( -0.1270800023317771588, -1.265791841079108027, -0.1270800023317771588 ) ) ;
#47323=CARTESIAN_POINT ( 'NONE',  ( -0.1113553986120547346, -0.8001968502861731558, 0.1113553986120547346 ) ) ;
#47345=CARTESIAN_POINT ( 'NONE',  ( 0.07405724077823318263, -0.05216535427694517224, -0.1787899950787401604 ) ) ;
#47354=CARTESIAN_POINT ( 'NONE',  ( -0.07405724077823318263, -1.784448818843874962, -0.1787899950787401604 ) ) ;
#47359=VECTOR ( 'NONE', #9957, 39.37007874015748143 ) ;
#47363=CARTESIAN_POINT ( 'NONE',  ( -0.07405724077823318263, -0.8898877477567983529, -0.1787899950787401604 ) ) ;
#47365=CARTESIAN_POINT ( 'NONE',  ( 3.284318927891251994E-17, 0.1274606299750234428, 0.1787899950787401882 ) ) ;
#47375=CARTESIAN_POINT ( 'NONE',  ( 3.301370929368692659E-17, -0.8966973528901319712, 0.1797182628040039365 ) ) ;
#47380=CARTESIAN_POINT ( 'NONE',  ( -0.1113553986120547346, -0.6230314960629921295, -0.1113553986120547346 ) ) ;
#47390=CARTESIAN_POINT ( 'NONE',  ( 0.1787899950787401882, -0.6894685038832439883, -2.189545951927503898E-17 ) ) ;
#47397=CARTESIAN_POINT ( 'NONE',  ( -0.1574803149606300301, -1.526082677165353951, -0.06523048226347956391 ) ) ;
#47404=CARTESIAN_POINT ( 'NONE',  ( -0.1574803149606299191, -0.3326771652468035745, 0.000000000000000000 ) ) ;
#47412=CARTESIAN_POINT ( 'NONE',  ( -0.1787899950787401882, -0.4100649131111284151, 0.000000000000000000 ) ) ;
#47413=CARTESIAN_POINT ( 'NONE',  ( -0.1399992916321618208, -0.09842519685039370636, 0.09114338793869390665 ) ) ;
#47415=DIRECTION ( 'NONE',  ( 0.000000000000000000, 1.000000000000000000, 0.000000000000000000 ) ) ;
#47422=( BOUNDED_CURVE ( )  B_SPLINE_CURVE ( 2, ( #22683, #25594, #22440, #44006, #15269 ),
 .UNSPECIFIED., .F., .F. ) 
 B_SPLINE_CURVE_WITH_KNOTS ( ( 3, 2, 3 ),
 ( 0.01000000005912435840, 0.01250000000000000069, 0.01499999999999999944 ),
 .UNSPECIFIED. ) 
 CURVE ( )  GEOMETRIC_REPRESENTATION_ITEM ( )  RATIONAL_B_SPLINE_CURVE ( ( 1.000000000000000000, 0.9238795325112869605, 1.000000000000000000, 0.9238795325112869605, 1.000000000000000000 ) ) 
 REPRESENTATION_ITEM ( '' )  ) ;
#47425=CARTESIAN_POINT ( 'NONE',  ( -0.07405724077823318263, -1.233267716481668774, -0.1787899950787401604 ) ) ;
#47427=CARTESIAN_POINT ( 'NONE',  ( 0.07405724077823318263, -1.430118110182456714, -0.1787899950787401604 ) ) ;
#47428=CARTESIAN_POINT ( 'NONE',  ( 0.000000000000000000, -0.09842519685039370636, 0.000000000000000000 ) ) ;
#47436=CARTESIAN_POINT ( 'NONE',  ( -0.1574803149606297803, -0.1432086614173227745, 0.06523048226347956391 ) ) ;
#47448=CARTESIAN_POINT ( 'NONE',  ( 0.1787899950787401604, -1.636811023568283341, 0.07405724077823318263 ) ) ;
#47449=CARTESIAN_POINT ( 'NONE',  ( -0.1574803149606297803, -1.590059055010582645, 0.06523048226347956391 ) ) ;
#47450=CARTESIAN_POINT ( 'NONE',  ( 0.07405724077823318263, -0.7657480314423001921, -0.1787899950787401604 ) ) ;
#47452=CARTESIAN_POINT ( 'NONE',  ( -0.06523048226347956391, -0.9798228346456692162, -0.1574803149606300301 ) ) ;
#47458=VERTEX_POINT ( 'NONE', #20416 ) ;
ENDSEC;
END-ISO-10303-21;
